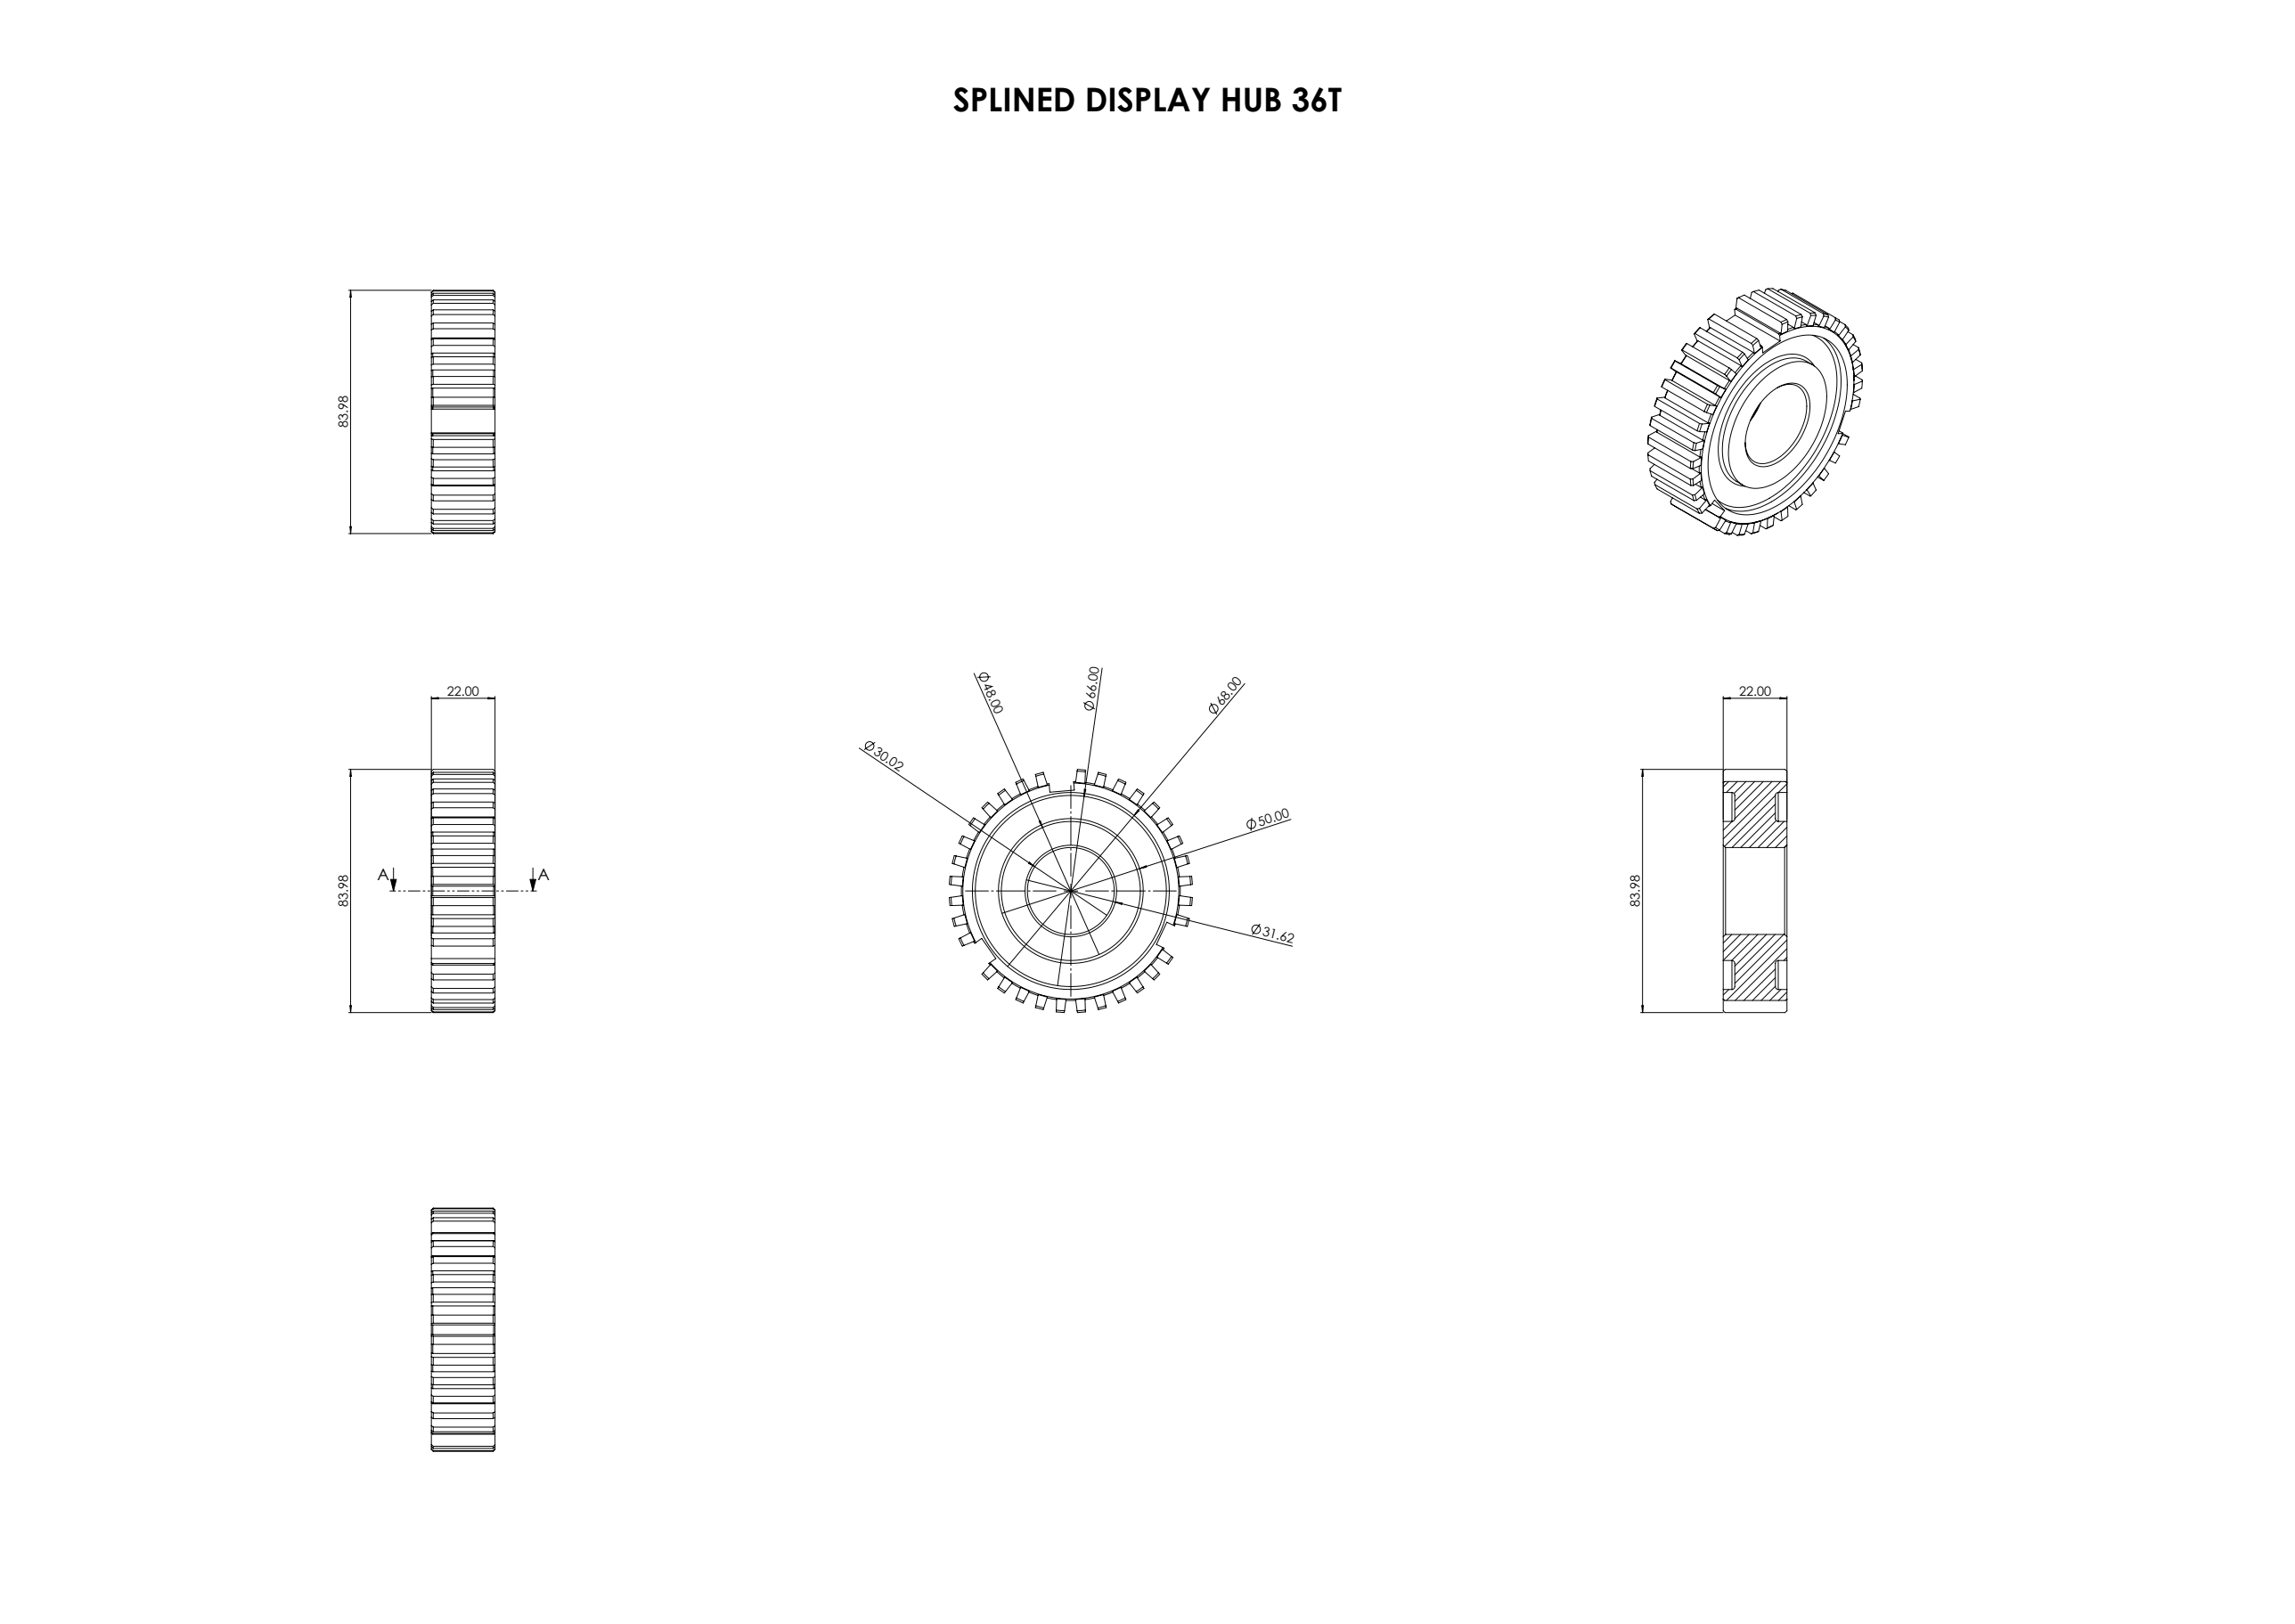
ISO-10303-21;
HEADER;
/* Generated by software containing ST-Developer
 * from STEP Tools, Inc. (www.steptools.com) 
 */

FILE_DESCRIPTION(
/* description */ (''),
/* implementation_level */ '2;1');

FILE_NAME(
/* name */ '02_Splined_Display_Hub_36T.step',
/* time_stamp */ '2026-10-11T08:27:52-07:00',
/* author */ (''),
/* organization */ (''),
/* preprocessor_version */ 'ST-DEVELOPER v20.2',
/* originating_system */ 'Autodesk Translation Framework v15.15.0.0',
/* authorisation */ '');

FILE_SCHEMA (('AUTOMOTIVE_DESIGN { 1 0 10303 214 3 1 1 }'));
ENDSEC;

DATA;
#10=MECHANICAL_DESIGN_GEOMETRIC_PRESENTATION_REPRESENTATION('',(#920),#94301);
#892=SHAPE_REPRESENTATION_RELATIONSHIP('SRR','None',#94372,#906);
#906=ADVANCED_BREP_SHAPE_REPRESENTATION('',(#934),#94288);
#920=STYLED_ITEM('',(#94595),#934);
#934=MANIFOLD_SOLID_BREP('Body1',#51019);
#950=TOROIDAL_SURFACE('',#54103,33.,1.);
#951=TOROIDAL_SURFACE('',#54112,33.,1.);
#952=TOROIDAL_SURFACE('',#54120,25.,1.);
#953=TOROIDAL_SURFACE('',#54126,25.,1.);
#963=FACE_BOUND('',#17327,.T.);
#964=FACE_BOUND('',#17673,.T.);
#965=FACE_BOUND('',#17677,.T.);
#966=FACE_BOUND('',#17686,.T.);
#967=FACE_BOUND('',#17688,.T.);
#968=FACE_BOUND('',#17690,.T.);
#1084=CYLINDRICAL_SURFACE('',#53612,37.8);
#1085=CYLINDRICAL_SURFACE('',#53689,37.8);
#1086=CYLINDRICAL_SURFACE('',#53706,37.8);
#1087=CYLINDRICAL_SURFACE('',#53942,37.8);
#1088=CYLINDRICAL_SURFACE('',#53943,37.8);
#1089=CYLINDRICAL_SURFACE('',#53948,37.8);
#1090=CYLINDRICAL_SURFACE('',#53953,37.8);
#1091=CYLINDRICAL_SURFACE('',#53958,37.8);
#1092=CYLINDRICAL_SURFACE('',#53963,37.8);
#1093=CYLINDRICAL_SURFACE('',#53968,37.8);
#1094=CYLINDRICAL_SURFACE('',#53973,37.8);
#1095=CYLINDRICAL_SURFACE('',#53978,37.8);
#1096=CYLINDRICAL_SURFACE('',#53983,37.8);
#1097=CYLINDRICAL_SURFACE('',#53988,37.8);
#1098=CYLINDRICAL_SURFACE('',#53993,37.8);
#1099=CYLINDRICAL_SURFACE('',#53998,37.8);
#1100=CYLINDRICAL_SURFACE('',#54003,37.8);
#1101=CYLINDRICAL_SURFACE('',#54008,37.8);
#1102=CYLINDRICAL_SURFACE('',#54013,37.8);
#1103=CYLINDRICAL_SURFACE('',#54018,37.8);
#1104=CYLINDRICAL_SURFACE('',#54023,37.8);
#1105=CYLINDRICAL_SURFACE('',#54028,37.8);
#1106=CYLINDRICAL_SURFACE('',#54033,37.8);
#1107=CYLINDRICAL_SURFACE('',#54038,37.8);
#1108=CYLINDRICAL_SURFACE('',#54043,37.8);
#1109=CYLINDRICAL_SURFACE('',#54048,37.8);
#1110=CYLINDRICAL_SURFACE('',#54053,37.8);
#1111=CYLINDRICAL_SURFACE('',#54058,37.8);
#1112=CYLINDRICAL_SURFACE('',#54063,37.8);
#1113=CYLINDRICAL_SURFACE('',#54068,37.8);
#1114=CYLINDRICAL_SURFACE('',#54073,37.8);
#1115=CYLINDRICAL_SURFACE('',#54078,37.8);
#1116=CYLINDRICAL_SURFACE('',#54083,37.8);
#1117=CYLINDRICAL_SURFACE('',#54088,37.8);
#1118=CYLINDRICAL_SURFACE('',#54093,37.8);
#1119=CYLINDRICAL_SURFACE('',#54098,37.8);
#1120=CYLINDRICAL_SURFACE('',#54110,34.);
#1121=CYLINDRICAL_SURFACE('',#54119,34.);
#1122=CYLINDRICAL_SURFACE('',#54124,24.);
#1123=CYLINDRICAL_SURFACE('',#54130,24.);
#1124=CYLINDRICAL_SURFACE('',#54132,15.01);
#4835=LINE('',#77424,#9363);
#4836=LINE('',#77426,#9364);
#4837=LINE('',#77428,#9365);
#4838=LINE('',#77433,#9366);
#4839=LINE('',#77441,#9367);
#4840=LINE('',#77447,#9368);
#4841=LINE('',#77449,#9369);
#4842=LINE('',#77450,#9370);
#4843=LINE('',#77452,#9371);
#4844=LINE('',#77453,#9372);
#4845=LINE('',#77458,#9373);
#4846=LINE('',#77626,#9374);
#4847=LINE('',#77628,#9375);
#4848=LINE('',#77630,#9376);
#4849=LINE('',#77634,#9377);
#4850=LINE('',#77636,#9378);
#4851=LINE('',#77638,#9379);
#4852=LINE('',#77962,#9380);
#4853=LINE('',#77963,#9381);
#4854=LINE('',#77964,#9382);
#4855=LINE('',#77972,#9383);
#4856=LINE('',#77977,#9384);
#4857=LINE('',#77978,#9385);
#4858=LINE('',#77980,#9386);
#4859=LINE('',#78304,#9387);
#4860=LINE('',#78467,#9388);
#4861=LINE('',#78468,#9389);
#4862=LINE('',#78469,#9390);
#4863=LINE('',#78471,#9391);
#4864=LINE('',#78473,#9392);
#4865=LINE('',#78474,#9393);
#4866=LINE('',#78476,#9394);
#4867=LINE('',#78478,#9395);
#4868=LINE('',#78976,#9396);
#4869=LINE('',#78982,#9397);
#4870=LINE('',#78983,#9398);
#4871=LINE('',#78984,#9399);
#4872=LINE('',#78986,#9400);
#4873=LINE('',#78987,#9401);
#4874=LINE('',#78990,#9402);
#4875=LINE('',#78996,#9403);
#4876=LINE('',#79002,#9404);
#4877=LINE('',#79003,#9405);
#4878=LINE('',#79004,#9406);
#4879=LINE('',#79006,#9407);
#4880=LINE('',#79007,#9408);
#4881=LINE('',#79010,#9409);
#4882=LINE('',#79016,#9410);
#4883=LINE('',#79022,#9411);
#4884=LINE('',#79023,#9412);
#4885=LINE('',#79024,#9413);
#4886=LINE('',#79026,#9414);
#4887=LINE('',#79027,#9415);
#4888=LINE('',#79030,#9416);
#4889=LINE('',#79036,#9417);
#4890=LINE('',#79042,#9418);
#4891=LINE('',#79043,#9419);
#4892=LINE('',#79044,#9420);
#4893=LINE('',#79046,#9421);
#4894=LINE('',#79047,#9422);
#4895=LINE('',#79050,#9423);
#4896=LINE('',#79056,#9424);
#4897=LINE('',#79062,#9425);
#4898=LINE('',#79063,#9426);
#4899=LINE('',#79064,#9427);
#4900=LINE('',#79066,#9428);
#4901=LINE('',#79067,#9429);
#4902=LINE('',#79070,#9430);
#4903=LINE('',#79076,#9431);
#4904=LINE('',#79082,#9432);
#4905=LINE('',#79083,#9433);
#4906=LINE('',#79084,#9434);
#4907=LINE('',#79086,#9435);
#4908=LINE('',#79087,#9436);
#4909=LINE('',#79090,#9437);
#4910=LINE('',#79096,#9438);
#4911=LINE('',#79102,#9439);
#4912=LINE('',#79103,#9440);
#4913=LINE('',#79104,#9441);
#4914=LINE('',#79106,#9442);
#4915=LINE('',#79107,#9443);
#4916=LINE('',#79110,#9444);
#4917=LINE('',#79116,#9445);
#4918=LINE('',#79122,#9446);
#4919=LINE('',#79123,#9447);
#4920=LINE('',#79124,#9448);
#4921=LINE('',#79126,#9449);
#4922=LINE('',#79127,#9450);
#4923=LINE('',#79130,#9451);
#4924=LINE('',#79136,#9452);
#4925=LINE('',#79142,#9453);
#4926=LINE('',#79143,#9454);
#4927=LINE('',#79144,#9455);
#4928=LINE('',#79146,#9456);
#4929=LINE('',#79147,#9457);
#4930=LINE('',#79150,#9458);
#4931=LINE('',#79156,#9459);
#4932=LINE('',#79162,#9460);
#4933=LINE('',#79163,#9461);
#4934=LINE('',#79164,#9462);
#4935=LINE('',#79166,#9463);
#4936=LINE('',#79167,#9464);
#4937=LINE('',#79170,#9465);
#4938=LINE('',#79176,#9466);
#4939=LINE('',#79182,#9467);
#4940=LINE('',#79183,#9468);
#4941=LINE('',#79184,#9469);
#4942=LINE('',#79186,#9470);
#4943=LINE('',#79187,#9471);
#4944=LINE('',#79190,#9472);
#4945=LINE('',#79196,#9473);
#4946=LINE('',#79202,#9474);
#4947=LINE('',#79203,#9475);
#4948=LINE('',#79204,#9476);
#4949=LINE('',#79206,#9477);
#4950=LINE('',#79207,#9478);
#4951=LINE('',#79210,#9479);
#4952=LINE('',#79216,#9480);
#4953=LINE('',#79222,#9481);
#4954=LINE('',#79223,#9482);
#4955=LINE('',#79224,#9483);
#4956=LINE('',#79226,#9484);
#4957=LINE('',#79227,#9485);
#4958=LINE('',#79230,#9486);
#4959=LINE('',#79236,#9487);
#4960=LINE('',#79242,#9488);
#4961=LINE('',#79243,#9489);
#4962=LINE('',#79244,#9490);
#4963=LINE('',#79246,#9491);
#4964=LINE('',#79247,#9492);
#4965=LINE('',#79250,#9493);
#4966=LINE('',#79256,#9494);
#4967=LINE('',#79262,#9495);
#4968=LINE('',#79263,#9496);
#4969=LINE('',#79264,#9497);
#4970=LINE('',#79266,#9498);
#4971=LINE('',#79267,#9499);
#4972=LINE('',#79270,#9500);
#4973=LINE('',#79276,#9501);
#4974=LINE('',#79282,#9502);
#4975=LINE('',#79283,#9503);
#4976=LINE('',#79284,#9504);
#4977=LINE('',#79286,#9505);
#4978=LINE('',#79287,#9506);
#4979=LINE('',#79290,#9507);
#4980=LINE('',#79296,#9508);
#4981=LINE('',#79302,#9509);
#4982=LINE('',#79303,#9510);
#4983=LINE('',#79304,#9511);
#4984=LINE('',#79306,#9512);
#4985=LINE('',#79307,#9513);
#4986=LINE('',#79310,#9514);
#4987=LINE('',#79316,#9515);
#4988=LINE('',#79322,#9516);
#4989=LINE('',#79323,#9517);
#4990=LINE('',#79324,#9518);
#4991=LINE('',#79326,#9519);
#4992=LINE('',#79327,#9520);
#4993=LINE('',#79330,#9521);
#4994=LINE('',#79336,#9522);
#4995=LINE('',#79342,#9523);
#4996=LINE('',#79343,#9524);
#4997=LINE('',#79344,#9525);
#4998=LINE('',#79346,#9526);
#4999=LINE('',#79347,#9527);
#5000=LINE('',#79350,#9528);
#5001=LINE('',#79356,#9529);
#5002=LINE('',#79362,#9530);
#5003=LINE('',#79363,#9531);
#5004=LINE('',#79364,#9532);
#5005=LINE('',#79366,#9533);
#5006=LINE('',#79367,#9534);
#5007=LINE('',#79370,#9535);
#5008=LINE('',#79376,#9536);
#5009=LINE('',#79382,#9537);
#5010=LINE('',#79383,#9538);
#5011=LINE('',#79384,#9539);
#5012=LINE('',#79386,#9540);
#5013=LINE('',#79387,#9541);
#5014=LINE('',#79390,#9542);
#5015=LINE('',#79396,#9543);
#5016=LINE('',#79402,#9544);
#5017=LINE('',#79403,#9545);
#5018=LINE('',#79404,#9546);
#5019=LINE('',#79406,#9547);
#5020=LINE('',#79407,#9548);
#5021=LINE('',#79410,#9549);
#5022=LINE('',#79416,#9550);
#5023=LINE('',#79422,#9551);
#5024=LINE('',#79423,#9552);
#5025=LINE('',#79424,#9553);
#5026=LINE('',#79426,#9554);
#5027=LINE('',#79427,#9555);
#5028=LINE('',#79430,#9556);
#5029=LINE('',#79436,#9557);
#5030=LINE('',#79442,#9558);
#5031=LINE('',#79443,#9559);
#5032=LINE('',#79444,#9560);
#5033=LINE('',#79446,#9561);
#5034=LINE('',#79447,#9562);
#5035=LINE('',#79450,#9563);
#5036=LINE('',#79456,#9564);
#5037=LINE('',#79462,#9565);
#5038=LINE('',#79463,#9566);
#5039=LINE('',#79464,#9567);
#5040=LINE('',#79466,#9568);
#5041=LINE('',#79467,#9569);
#5042=LINE('',#79470,#9570);
#5043=LINE('',#79476,#9571);
#5044=LINE('',#79482,#9572);
#5045=LINE('',#79483,#9573);
#5046=LINE('',#79484,#9574);
#5047=LINE('',#79486,#9575);
#5048=LINE('',#79487,#9576);
#5049=LINE('',#79490,#9577);
#5050=LINE('',#79496,#9578);
#5051=LINE('',#79502,#9579);
#5052=LINE('',#79503,#9580);
#5053=LINE('',#79504,#9581);
#5054=LINE('',#79506,#9582);
#5055=LINE('',#79507,#9583);
#5056=LINE('',#79510,#9584);
#5057=LINE('',#79516,#9585);
#5058=LINE('',#79522,#9586);
#5059=LINE('',#79523,#9587);
#5060=LINE('',#79524,#9588);
#5061=LINE('',#79526,#9589);
#5062=LINE('',#79527,#9590);
#5063=LINE('',#79530,#9591);
#5064=LINE('',#79536,#9592);
#5065=LINE('',#79542,#9593);
#5066=LINE('',#79543,#9594);
#5067=LINE('',#79544,#9595);
#5068=LINE('',#79546,#9596);
#5069=LINE('',#79547,#9597);
#5070=LINE('',#79550,#9598);
#5071=LINE('',#79556,#9599);
#5072=LINE('',#79562,#9600);
#5073=LINE('',#79563,#9601);
#5074=LINE('',#79564,#9602);
#5075=LINE('',#79566,#9603);
#5076=LINE('',#79567,#9604);
#5077=LINE('',#79570,#9605);
#5078=LINE('',#79576,#9606);
#5079=LINE('',#79582,#9607);
#5080=LINE('',#79583,#9608);
#5081=LINE('',#79584,#9609);
#5082=LINE('',#79586,#9610);
#5083=LINE('',#79587,#9611);
#5084=LINE('',#79590,#9612);
#5085=LINE('',#79596,#9613);
#5086=LINE('',#79602,#9614);
#5087=LINE('',#79603,#9615);
#5088=LINE('',#79604,#9616);
#5089=LINE('',#79606,#9617);
#5090=LINE('',#79607,#9618);
#5091=LINE('',#79610,#9619);
#5092=LINE('',#79616,#9620);
#5093=LINE('',#79622,#9621);
#5094=LINE('',#79623,#9622);
#5095=LINE('',#79624,#9623);
#5096=LINE('',#79626,#9624);
#5097=LINE('',#79627,#9625);
#5098=LINE('',#79630,#9626);
#5099=LINE('',#79834,#9627);
#5100=LINE('',#79835,#9628);
#5101=LINE('',#79836,#9629);
#5102=LINE('',#79838,#9630);
#5103=LINE('',#79839,#9631);
#5104=LINE('',#79842,#9632);
#5105=LINE('',#79843,#9633);
#5106=LINE('',#79844,#9634);
#5107=LINE('',#79846,#9635);
#5108=LINE('',#79847,#9636);
#5109=LINE('',#79850,#9637);
#5110=LINE('',#79851,#9638);
#5111=LINE('',#79852,#9639);
#5112=LINE('',#79854,#9640);
#5113=LINE('',#79855,#9641);
#5114=LINE('',#79858,#9642);
#5115=LINE('',#79859,#9643);
#5116=LINE('',#79860,#9644);
#5117=LINE('',#79862,#9645);
#5118=LINE('',#79863,#9646);
#5119=LINE('',#79866,#9647);
#5120=LINE('',#79867,#9648);
#5121=LINE('',#79868,#9649);
#5122=LINE('',#79870,#9650);
#5123=LINE('',#79871,#9651);
#5124=LINE('',#79874,#9652);
#5125=LINE('',#79875,#9653);
#5126=LINE('',#79876,#9654);
#5127=LINE('',#79878,#9655);
#5128=LINE('',#79879,#9656);
#5129=LINE('',#79882,#9657);
#5130=LINE('',#79883,#9658);
#5131=LINE('',#79884,#9659);
#5132=LINE('',#79886,#9660);
#5133=LINE('',#79887,#9661);
#5134=LINE('',#79890,#9662);
#5135=LINE('',#79891,#9663);
#5136=LINE('',#79892,#9664);
#5137=LINE('',#79894,#9665);
#5138=LINE('',#79895,#9666);
#5139=LINE('',#79898,#9667);
#5140=LINE('',#79899,#9668);
#5141=LINE('',#79900,#9669);
#5142=LINE('',#79902,#9670);
#5143=LINE('',#79903,#9671);
#5144=LINE('',#79906,#9672);
#5145=LINE('',#79907,#9673);
#5146=LINE('',#79908,#9674);
#5147=LINE('',#79910,#9675);
#5148=LINE('',#79911,#9676);
#5149=LINE('',#79914,#9677);
#5150=LINE('',#79915,#9678);
#5151=LINE('',#79917,#9679);
#5152=LINE('',#79918,#9680);
#5153=LINE('',#79921,#9681);
#5154=LINE('',#79922,#9682);
#5155=LINE('',#79923,#9683);
#5156=LINE('',#79925,#9684);
#5157=LINE('',#79926,#9685);
#5158=LINE('',#79929,#9686);
#5159=LINE('',#79930,#9687);
#5160=LINE('',#79931,#9688);
#5161=LINE('',#79933,#9689);
#5162=LINE('',#79934,#9690);
#5163=LINE('',#79937,#9691);
#5164=LINE('',#79938,#9692);
#5165=LINE('',#79939,#9693);
#5166=LINE('',#79941,#9694);
#5167=LINE('',#79942,#9695);
#5168=LINE('',#79945,#9696);
#5169=LINE('',#79946,#9697);
#5170=LINE('',#79947,#9698);
#5171=LINE('',#79949,#9699);
#5172=LINE('',#79950,#9700);
#5173=LINE('',#79953,#9701);
#5174=LINE('',#79954,#9702);
#5175=LINE('',#79955,#9703);
#5176=LINE('',#79957,#9704);
#5177=LINE('',#79958,#9705);
#5178=LINE('',#79961,#9706);
#5179=LINE('',#79962,#9707);
#5180=LINE('',#79963,#9708);
#5181=LINE('',#79965,#9709);
#5182=LINE('',#79966,#9710);
#5183=LINE('',#79969,#9711);
#5184=LINE('',#79970,#9712);
#5185=LINE('',#79971,#9713);
#5186=LINE('',#79973,#9714);
#5187=LINE('',#79974,#9715);
#5188=LINE('',#79977,#9716);
#5189=LINE('',#79978,#9717);
#5190=LINE('',#79979,#9718);
#5191=LINE('',#79981,#9719);
#5192=LINE('',#79982,#9720);
#5193=LINE('',#79985,#9721);
#5194=LINE('',#79986,#9722);
#5195=LINE('',#79987,#9723);
#5196=LINE('',#79989,#9724);
#5197=LINE('',#79990,#9725);
#5198=LINE('',#79993,#9726);
#5199=LINE('',#79994,#9727);
#5200=LINE('',#79995,#9728);
#5201=LINE('',#79997,#9729);
#5202=LINE('',#79998,#9730);
#5203=LINE('',#80001,#9731);
#5204=LINE('',#80002,#9732);
#5205=LINE('',#80004,#9733);
#5206=LINE('',#80005,#9734);
#5207=LINE('',#80008,#9735);
#5208=LINE('',#80009,#9736);
#5209=LINE('',#80010,#9737);
#5210=LINE('',#80012,#9738);
#5211=LINE('',#80013,#9739);
#5212=LINE('',#80016,#9740);
#5213=LINE('',#80017,#9741);
#5214=LINE('',#80018,#9742);
#5215=LINE('',#80020,#9743);
#5216=LINE('',#80021,#9744);
#5217=LINE('',#80024,#9745);
#5218=LINE('',#80025,#9746);
#5219=LINE('',#80026,#9747);
#5220=LINE('',#80028,#9748);
#5221=LINE('',#80029,#9749);
#5222=LINE('',#80032,#9750);
#5223=LINE('',#80033,#9751);
#5224=LINE('',#80034,#9752);
#5225=LINE('',#80036,#9753);
#5226=LINE('',#80037,#9754);
#5227=LINE('',#80040,#9755);
#5228=LINE('',#80041,#9756);
#5229=LINE('',#80042,#9757);
#5230=LINE('',#80044,#9758);
#5231=LINE('',#80045,#9759);
#5232=LINE('',#80048,#9760);
#5233=LINE('',#80049,#9761);
#5234=LINE('',#80050,#9762);
#5235=LINE('',#80052,#9763);
#5236=LINE('',#80053,#9764);
#5237=LINE('',#80056,#9765);
#5238=LINE('',#80057,#9766);
#5239=LINE('',#80058,#9767);
#5240=LINE('',#80060,#9768);
#5241=LINE('',#80061,#9769);
#5242=LINE('',#80064,#9770);
#5243=LINE('',#80065,#9771);
#5244=LINE('',#80066,#9772);
#5245=LINE('',#80068,#9773);
#5246=LINE('',#80069,#9774);
#5247=LINE('',#80072,#9775);
#5248=LINE('',#80073,#9776);
#5249=LINE('',#80074,#9777);
#5250=LINE('',#80076,#9778);
#5251=LINE('',#80077,#9779);
#5252=LINE('',#80080,#9780);
#5253=LINE('',#80081,#9781);
#5254=LINE('',#80082,#9782);
#5255=LINE('',#80084,#9783);
#5256=LINE('',#80085,#9784);
#5257=LINE('',#80088,#9785);
#5258=LINE('',#80089,#9786);
#5259=LINE('',#80091,#9787);
#5260=LINE('',#80092,#9788);
#5261=LINE('',#80094,#9789);
#5262=LINE('',#80096,#9790);
#5263=LINE('',#80102,#9791);
#5264=LINE('',#80104,#9792);
#5265=LINE('',#80109,#9793);
#5266=LINE('',#80111,#9794);
#5267=LINE('',#80116,#9795);
#5268=LINE('',#80118,#9796);
#5269=LINE('',#80123,#9797);
#5270=LINE('',#80125,#9798);
#5271=LINE('',#80130,#9799);
#5272=LINE('',#80132,#9800);
#5273=LINE('',#80137,#9801);
#5274=LINE('',#80139,#9802);
#5275=LINE('',#80144,#9803);
#5276=LINE('',#80146,#9804);
#5277=LINE('',#80151,#9805);
#5278=LINE('',#80153,#9806);
#5279=LINE('',#80158,#9807);
#5280=LINE('',#80160,#9808);
#5281=LINE('',#80165,#9809);
#5282=LINE('',#80167,#9810);
#5283=LINE('',#80172,#9811);
#5284=LINE('',#80174,#9812);
#5285=LINE('',#80179,#9813);
#5286=LINE('',#80181,#9814);
#5287=LINE('',#80186,#9815);
#5288=LINE('',#80188,#9816);
#5289=LINE('',#80193,#9817);
#5290=LINE('',#80195,#9818);
#5291=LINE('',#80200,#9819);
#5292=LINE('',#80202,#9820);
#5293=LINE('',#80207,#9821);
#5294=LINE('',#80209,#9822);
#5295=LINE('',#80214,#9823);
#5296=LINE('',#80216,#9824);
#5297=LINE('',#80221,#9825);
#5298=LINE('',#80223,#9826);
#5299=LINE('',#80228,#9827);
#5300=LINE('',#80230,#9828);
#5301=LINE('',#80235,#9829);
#5302=LINE('',#80237,#9830);
#5303=LINE('',#80242,#9831);
#5304=LINE('',#80244,#9832);
#5305=LINE('',#80249,#9833);
#5306=LINE('',#80251,#9834);
#5307=LINE('',#80256,#9835);
#5308=LINE('',#80258,#9836);
#5309=LINE('',#80263,#9837);
#5310=LINE('',#80265,#9838);
#5311=LINE('',#80270,#9839);
#5312=LINE('',#80272,#9840);
#5313=LINE('',#80277,#9841);
#5314=LINE('',#80279,#9842);
#5315=LINE('',#80284,#9843);
#5316=LINE('',#80286,#9844);
#5317=LINE('',#80291,#9845);
#5318=LINE('',#80293,#9846);
#5319=LINE('',#80298,#9847);
#5320=LINE('',#80300,#9848);
#5321=LINE('',#80305,#9849);
#5322=LINE('',#80307,#9850);
#5323=LINE('',#80312,#9851);
#5324=LINE('',#80314,#9852);
#5325=LINE('',#80319,#9853);
#5326=LINE('',#80321,#9854);
#5327=LINE('',#80338,#9855);
#5328=LINE('',#80351,#9856);
#5329=LINE('',#80361,#9857);
#5330=LINE('',#80370,#9858);
#5331=LINE('',#80376,#9859);
#5332=LINE('',#80380,#9860);
#5333=LINE('',#80388,#9861);
#9363=VECTOR('',#62889,10.);
#9364=VECTOR('',#62890,10.);
#9365=VECTOR('',#62891,10.);
#9366=VECTOR('',#62892,10.);
#9367=VECTOR('',#62895,10.);
#9368=VECTOR('',#62896,10.);
#9369=VECTOR('',#62897,10.);
#9370=VECTOR('',#62898,10.);
#9371=VECTOR('',#62901,10.);
#9372=VECTOR('',#62902,10.);
#9373=VECTOR('',#62907,10.);
#9374=VECTOR('',#62942,10.);
#9375=VECTOR('',#62943,10.);
#9376=VECTOR('',#62944,10.);
#9377=VECTOR('',#62947,10.);
#9378=VECTOR('',#62948,10.);
#9379=VECTOR('',#62949,10.);
#9380=VECTOR('',#63006,10.);
#9381=VECTOR('',#63007,10.);
#9382=VECTOR('',#63008,10.);
#9383=VECTOR('',#63011,10.);
#9384=VECTOR('',#63012,10.);
#9385=VECTOR('',#63013,10.);
#9386=VECTOR('',#63016,10.);
#9387=VECTOR('',#63073,10.);
#9388=VECTOR('',#63102,10.);
#9389=VECTOR('',#63103,10.);
#9390=VECTOR('',#63104,10.);
#9391=VECTOR('',#63107,10.);
#9392=VECTOR('',#63108,10.);
#9393=VECTOR('',#63109,10.);
#9394=VECTOR('',#63112,10.);
#9395=VECTOR('',#63115,10.);
#9396=VECTOR('',#63250,10.);
#9397=VECTOR('',#63251,10.);
#9398=VECTOR('',#63252,10.);
#9399=VECTOR('',#63253,10.);
#9400=VECTOR('',#63254,10.);
#9401=VECTOR('',#63255,10.);
#9402=VECTOR('',#63258,10.);
#9403=VECTOR('',#63261,10.);
#9404=VECTOR('',#63262,10.);
#9405=VECTOR('',#63263,10.);
#9406=VECTOR('',#63264,10.);
#9407=VECTOR('',#63265,10.);
#9408=VECTOR('',#63266,10.);
#9409=VECTOR('',#63269,10.);
#9410=VECTOR('',#63272,10.);
#9411=VECTOR('',#63273,10.);
#9412=VECTOR('',#63274,10.);
#9413=VECTOR('',#63275,10.);
#9414=VECTOR('',#63276,10.);
#9415=VECTOR('',#63277,10.);
#9416=VECTOR('',#63280,10.);
#9417=VECTOR('',#63283,10.);
#9418=VECTOR('',#63284,10.);
#9419=VECTOR('',#63285,10.);
#9420=VECTOR('',#63286,10.);
#9421=VECTOR('',#63287,10.);
#9422=VECTOR('',#63288,10.);
#9423=VECTOR('',#63291,10.);
#9424=VECTOR('',#63294,10.);
#9425=VECTOR('',#63295,10.);
#9426=VECTOR('',#63296,10.);
#9427=VECTOR('',#63297,10.);
#9428=VECTOR('',#63298,10.);
#9429=VECTOR('',#63299,10.);
#9430=VECTOR('',#63302,10.);
#9431=VECTOR('',#63305,10.);
#9432=VECTOR('',#63306,10.);
#9433=VECTOR('',#63307,10.);
#9434=VECTOR('',#63308,10.);
#9435=VECTOR('',#63309,10.);
#9436=VECTOR('',#63310,10.);
#9437=VECTOR('',#63313,10.);
#9438=VECTOR('',#63316,10.);
#9439=VECTOR('',#63317,10.);
#9440=VECTOR('',#63318,10.);
#9441=VECTOR('',#63319,10.);
#9442=VECTOR('',#63320,10.);
#9443=VECTOR('',#63321,10.);
#9444=VECTOR('',#63324,10.);
#9445=VECTOR('',#63327,10.);
#9446=VECTOR('',#63328,10.);
#9447=VECTOR('',#63329,10.);
#9448=VECTOR('',#63330,10.);
#9449=VECTOR('',#63331,10.);
#9450=VECTOR('',#63332,10.);
#9451=VECTOR('',#63335,10.);
#9452=VECTOR('',#63338,10.);
#9453=VECTOR('',#63339,10.);
#9454=VECTOR('',#63340,10.);
#9455=VECTOR('',#63341,10.);
#9456=VECTOR('',#63342,10.);
#9457=VECTOR('',#63343,10.);
#9458=VECTOR('',#63346,10.);
#9459=VECTOR('',#63349,10.);
#9460=VECTOR('',#63350,10.);
#9461=VECTOR('',#63351,10.);
#9462=VECTOR('',#63352,10.);
#9463=VECTOR('',#63353,10.);
#9464=VECTOR('',#63354,10.);
#9465=VECTOR('',#63357,10.);
#9466=VECTOR('',#63360,10.);
#9467=VECTOR('',#63361,10.);
#9468=VECTOR('',#63362,10.);
#9469=VECTOR('',#63363,10.);
#9470=VECTOR('',#63364,10.);
#9471=VECTOR('',#63365,10.);
#9472=VECTOR('',#63368,10.);
#9473=VECTOR('',#63371,10.);
#9474=VECTOR('',#63372,10.);
#9475=VECTOR('',#63373,10.);
#9476=VECTOR('',#63374,10.);
#9477=VECTOR('',#63375,10.);
#9478=VECTOR('',#63376,10.);
#9479=VECTOR('',#63379,10.);
#9480=VECTOR('',#63382,10.);
#9481=VECTOR('',#63383,10.);
#9482=VECTOR('',#63384,10.);
#9483=VECTOR('',#63385,10.);
#9484=VECTOR('',#63386,10.);
#9485=VECTOR('',#63387,10.);
#9486=VECTOR('',#63390,10.);
#9487=VECTOR('',#63393,10.);
#9488=VECTOR('',#63394,10.);
#9489=VECTOR('',#63395,10.);
#9490=VECTOR('',#63396,10.);
#9491=VECTOR('',#63397,10.);
#9492=VECTOR('',#63398,10.);
#9493=VECTOR('',#63401,10.);
#9494=VECTOR('',#63404,10.);
#9495=VECTOR('',#63405,10.);
#9496=VECTOR('',#63406,10.);
#9497=VECTOR('',#63407,10.);
#9498=VECTOR('',#63408,10.);
#9499=VECTOR('',#63409,10.);
#9500=VECTOR('',#63412,10.);
#9501=VECTOR('',#63415,10.);
#9502=VECTOR('',#63416,10.);
#9503=VECTOR('',#63417,10.);
#9504=VECTOR('',#63418,10.);
#9505=VECTOR('',#63419,10.);
#9506=VECTOR('',#63420,10.);
#9507=VECTOR('',#63423,10.);
#9508=VECTOR('',#63426,10.);
#9509=VECTOR('',#63427,10.);
#9510=VECTOR('',#63428,10.);
#9511=VECTOR('',#63429,10.);
#9512=VECTOR('',#63430,10.);
#9513=VECTOR('',#63431,10.);
#9514=VECTOR('',#63434,10.);
#9515=VECTOR('',#63437,10.);
#9516=VECTOR('',#63438,10.);
#9517=VECTOR('',#63439,10.);
#9518=VECTOR('',#63440,10.);
#9519=VECTOR('',#63441,10.);
#9520=VECTOR('',#63442,10.);
#9521=VECTOR('',#63445,10.);
#9522=VECTOR('',#63448,10.);
#9523=VECTOR('',#63449,10.);
#9524=VECTOR('',#63450,10.);
#9525=VECTOR('',#63451,10.);
#9526=VECTOR('',#63452,10.);
#9527=VECTOR('',#63453,10.);
#9528=VECTOR('',#63456,10.);
#9529=VECTOR('',#63459,10.);
#9530=VECTOR('',#63460,10.);
#9531=VECTOR('',#63461,10.);
#9532=VECTOR('',#63462,10.);
#9533=VECTOR('',#63463,10.);
#9534=VECTOR('',#63464,10.);
#9535=VECTOR('',#63467,10.);
#9536=VECTOR('',#63470,10.);
#9537=VECTOR('',#63471,10.);
#9538=VECTOR('',#63472,10.);
#9539=VECTOR('',#63473,10.);
#9540=VECTOR('',#63474,10.);
#9541=VECTOR('',#63475,10.);
#9542=VECTOR('',#63478,10.);
#9543=VECTOR('',#63481,10.);
#9544=VECTOR('',#63482,10.);
#9545=VECTOR('',#63483,10.);
#9546=VECTOR('',#63484,10.);
#9547=VECTOR('',#63485,10.);
#9548=VECTOR('',#63486,10.);
#9549=VECTOR('',#63489,10.);
#9550=VECTOR('',#63492,10.);
#9551=VECTOR('',#63493,10.);
#9552=VECTOR('',#63494,10.);
#9553=VECTOR('',#63495,10.);
#9554=VECTOR('',#63496,10.);
#9555=VECTOR('',#63497,10.);
#9556=VECTOR('',#63500,10.);
#9557=VECTOR('',#63503,10.);
#9558=VECTOR('',#63504,10.);
#9559=VECTOR('',#63505,10.);
#9560=VECTOR('',#63506,10.);
#9561=VECTOR('',#63507,10.);
#9562=VECTOR('',#63508,10.);
#9563=VECTOR('',#63511,10.);
#9564=VECTOR('',#63514,10.);
#9565=VECTOR('',#63515,10.);
#9566=VECTOR('',#63516,10.);
#9567=VECTOR('',#63517,10.);
#9568=VECTOR('',#63518,10.);
#9569=VECTOR('',#63519,10.);
#9570=VECTOR('',#63522,10.);
#9571=VECTOR('',#63525,10.);
#9572=VECTOR('',#63526,10.);
#9573=VECTOR('',#63527,10.);
#9574=VECTOR('',#63528,10.);
#9575=VECTOR('',#63529,10.);
#9576=VECTOR('',#63530,10.);
#9577=VECTOR('',#63533,10.);
#9578=VECTOR('',#63536,10.);
#9579=VECTOR('',#63537,10.);
#9580=VECTOR('',#63538,10.);
#9581=VECTOR('',#63539,10.);
#9582=VECTOR('',#63540,10.);
#9583=VECTOR('',#63541,10.);
#9584=VECTOR('',#63544,10.);
#9585=VECTOR('',#63547,10.);
#9586=VECTOR('',#63548,10.);
#9587=VECTOR('',#63549,10.);
#9588=VECTOR('',#63550,10.);
#9589=VECTOR('',#63551,10.);
#9590=VECTOR('',#63552,10.);
#9591=VECTOR('',#63555,10.);
#9592=VECTOR('',#63558,10.);
#9593=VECTOR('',#63559,10.);
#9594=VECTOR('',#63560,10.);
#9595=VECTOR('',#63561,10.);
#9596=VECTOR('',#63562,10.);
#9597=VECTOR('',#63563,10.);
#9598=VECTOR('',#63566,10.);
#9599=VECTOR('',#63569,10.);
#9600=VECTOR('',#63570,10.);
#9601=VECTOR('',#63571,10.);
#9602=VECTOR('',#63572,10.);
#9603=VECTOR('',#63573,10.);
#9604=VECTOR('',#63574,10.);
#9605=VECTOR('',#63577,10.);
#9606=VECTOR('',#63580,10.);
#9607=VECTOR('',#63581,10.);
#9608=VECTOR('',#63582,10.);
#9609=VECTOR('',#63583,10.);
#9610=VECTOR('',#63584,10.);
#9611=VECTOR('',#63585,10.);
#9612=VECTOR('',#63588,10.);
#9613=VECTOR('',#63591,10.);
#9614=VECTOR('',#63592,10.);
#9615=VECTOR('',#63593,10.);
#9616=VECTOR('',#63594,10.);
#9617=VECTOR('',#63595,10.);
#9618=VECTOR('',#63596,10.);
#9619=VECTOR('',#63599,10.);
#9620=VECTOR('',#63602,10.);
#9621=VECTOR('',#63603,10.);
#9622=VECTOR('',#63604,10.);
#9623=VECTOR('',#63605,10.);
#9624=VECTOR('',#63606,10.);
#9625=VECTOR('',#63607,10.);
#9626=VECTOR('',#63610,10.);
#9627=VECTOR('',#63745,10.);
#9628=VECTOR('',#63746,10.);
#9629=VECTOR('',#63747,10.);
#9630=VECTOR('',#63748,10.);
#9631=VECTOR('',#63749,10.);
#9632=VECTOR('',#63752,10.);
#9633=VECTOR('',#63753,10.);
#9634=VECTOR('',#63754,10.);
#9635=VECTOR('',#63755,10.);
#9636=VECTOR('',#63756,10.);
#9637=VECTOR('',#63759,10.);
#9638=VECTOR('',#63760,10.);
#9639=VECTOR('',#63761,10.);
#9640=VECTOR('',#63762,10.);
#9641=VECTOR('',#63763,10.);
#9642=VECTOR('',#63766,10.);
#9643=VECTOR('',#63767,10.);
#9644=VECTOR('',#63768,10.);
#9645=VECTOR('',#63769,10.);
#9646=VECTOR('',#63770,10.);
#9647=VECTOR('',#63773,10.);
#9648=VECTOR('',#63774,10.);
#9649=VECTOR('',#63775,10.);
#9650=VECTOR('',#63776,10.);
#9651=VECTOR('',#63777,10.);
#9652=VECTOR('',#63780,10.);
#9653=VECTOR('',#63781,10.);
#9654=VECTOR('',#63782,10.);
#9655=VECTOR('',#63783,10.);
#9656=VECTOR('',#63784,10.);
#9657=VECTOR('',#63787,10.);
#9658=VECTOR('',#63788,10.);
#9659=VECTOR('',#63789,10.);
#9660=VECTOR('',#63790,10.);
#9661=VECTOR('',#63791,10.);
#9662=VECTOR('',#63794,10.);
#9663=VECTOR('',#63795,10.);
#9664=VECTOR('',#63796,10.);
#9665=VECTOR('',#63797,10.);
#9666=VECTOR('',#63798,10.);
#9667=VECTOR('',#63801,10.);
#9668=VECTOR('',#63802,10.);
#9669=VECTOR('',#63803,10.);
#9670=VECTOR('',#63804,10.);
#9671=VECTOR('',#63805,10.);
#9672=VECTOR('',#63808,10.);
#9673=VECTOR('',#63809,10.);
#9674=VECTOR('',#63810,10.);
#9675=VECTOR('',#63811,10.);
#9676=VECTOR('',#63812,10.);
#9677=VECTOR('',#63815,10.);
#9678=VECTOR('',#63816,10.);
#9679=VECTOR('',#63817,10.);
#9680=VECTOR('',#63818,10.);
#9681=VECTOR('',#63821,10.);
#9682=VECTOR('',#63822,10.);
#9683=VECTOR('',#63823,10.);
#9684=VECTOR('',#63824,10.);
#9685=VECTOR('',#63825,10.);
#9686=VECTOR('',#63828,10.);
#9687=VECTOR('',#63829,10.);
#9688=VECTOR('',#63830,10.);
#9689=VECTOR('',#63831,10.);
#9690=VECTOR('',#63832,10.);
#9691=VECTOR('',#63835,10.);
#9692=VECTOR('',#63836,10.);
#9693=VECTOR('',#63837,10.);
#9694=VECTOR('',#63838,10.);
#9695=VECTOR('',#63839,10.);
#9696=VECTOR('',#63842,10.);
#9697=VECTOR('',#63843,10.);
#9698=VECTOR('',#63844,10.);
#9699=VECTOR('',#63845,10.);
#9700=VECTOR('',#63846,10.);
#9701=VECTOR('',#63849,10.);
#9702=VECTOR('',#63850,10.);
#9703=VECTOR('',#63851,10.);
#9704=VECTOR('',#63852,10.);
#9705=VECTOR('',#63853,10.);
#9706=VECTOR('',#63856,10.);
#9707=VECTOR('',#63857,10.);
#9708=VECTOR('',#63858,10.);
#9709=VECTOR('',#63859,10.);
#9710=VECTOR('',#63860,10.);
#9711=VECTOR('',#63863,10.);
#9712=VECTOR('',#63864,10.);
#9713=VECTOR('',#63865,10.);
#9714=VECTOR('',#63866,10.);
#9715=VECTOR('',#63867,10.);
#9716=VECTOR('',#63870,10.);
#9717=VECTOR('',#63871,10.);
#9718=VECTOR('',#63872,10.);
#9719=VECTOR('',#63873,10.);
#9720=VECTOR('',#63874,10.);
#9721=VECTOR('',#63877,10.);
#9722=VECTOR('',#63878,10.);
#9723=VECTOR('',#63879,10.);
#9724=VECTOR('',#63880,10.);
#9725=VECTOR('',#63881,10.);
#9726=VECTOR('',#63884,10.);
#9727=VECTOR('',#63885,10.);
#9728=VECTOR('',#63886,10.);
#9729=VECTOR('',#63887,10.);
#9730=VECTOR('',#63888,10.);
#9731=VECTOR('',#63891,10.);
#9732=VECTOR('',#63892,10.);
#9733=VECTOR('',#63893,10.);
#9734=VECTOR('',#63894,10.);
#9735=VECTOR('',#63897,10.);
#9736=VECTOR('',#63898,10.);
#9737=VECTOR('',#63899,10.);
#9738=VECTOR('',#63900,10.);
#9739=VECTOR('',#63901,10.);
#9740=VECTOR('',#63904,10.);
#9741=VECTOR('',#63905,10.);
#9742=VECTOR('',#63906,10.);
#9743=VECTOR('',#63907,10.);
#9744=VECTOR('',#63908,10.);
#9745=VECTOR('',#63911,10.);
#9746=VECTOR('',#63912,10.);
#9747=VECTOR('',#63913,10.);
#9748=VECTOR('',#63914,10.);
#9749=VECTOR('',#63915,10.);
#9750=VECTOR('',#63918,10.);
#9751=VECTOR('',#63919,10.);
#9752=VECTOR('',#63920,10.);
#9753=VECTOR('',#63921,10.);
#9754=VECTOR('',#63922,10.);
#9755=VECTOR('',#63925,10.);
#9756=VECTOR('',#63926,10.);
#9757=VECTOR('',#63927,10.);
#9758=VECTOR('',#63928,10.);
#9759=VECTOR('',#63929,10.);
#9760=VECTOR('',#63932,10.);
#9761=VECTOR('',#63933,10.);
#9762=VECTOR('',#63934,10.);
#9763=VECTOR('',#63935,10.);
#9764=VECTOR('',#63936,10.);
#9765=VECTOR('',#63939,10.);
#9766=VECTOR('',#63940,10.);
#9767=VECTOR('',#63941,10.);
#9768=VECTOR('',#63942,10.);
#9769=VECTOR('',#63943,10.);
#9770=VECTOR('',#63946,10.);
#9771=VECTOR('',#63947,10.);
#9772=VECTOR('',#63948,10.);
#9773=VECTOR('',#63949,10.);
#9774=VECTOR('',#63950,10.);
#9775=VECTOR('',#63953,10.);
#9776=VECTOR('',#63954,10.);
#9777=VECTOR('',#63955,10.);
#9778=VECTOR('',#63956,10.);
#9779=VECTOR('',#63957,10.);
#9780=VECTOR('',#63960,10.);
#9781=VECTOR('',#63961,10.);
#9782=VECTOR('',#63962,10.);
#9783=VECTOR('',#63963,10.);
#9784=VECTOR('',#63964,10.);
#9785=VECTOR('',#63967,10.);
#9786=VECTOR('',#63968,10.);
#9787=VECTOR('',#63969,10.);
#9788=VECTOR('',#63970,10.);
#9789=VECTOR('',#63973,10.);
#9790=VECTOR('',#63976,10.);
#9791=VECTOR('',#63987,10.);
#9792=VECTOR('',#63990,10.);
#9793=VECTOR('',#63999,10.);
#9794=VECTOR('',#64002,10.);
#9795=VECTOR('',#64011,10.);
#9796=VECTOR('',#64014,10.);
#9797=VECTOR('',#64023,10.);
#9798=VECTOR('',#64026,10.);
#9799=VECTOR('',#64035,10.);
#9800=VECTOR('',#64038,10.);
#9801=VECTOR('',#64047,10.);
#9802=VECTOR('',#64050,10.);
#9803=VECTOR('',#64059,10.);
#9804=VECTOR('',#64062,10.);
#9805=VECTOR('',#64071,10.);
#9806=VECTOR('',#64074,10.);
#9807=VECTOR('',#64083,10.);
#9808=VECTOR('',#64086,10.);
#9809=VECTOR('',#64095,10.);
#9810=VECTOR('',#64098,10.);
#9811=VECTOR('',#64107,10.);
#9812=VECTOR('',#64110,10.);
#9813=VECTOR('',#64119,10.);
#9814=VECTOR('',#64122,10.);
#9815=VECTOR('',#64131,10.);
#9816=VECTOR('',#64134,10.);
#9817=VECTOR('',#64143,10.);
#9818=VECTOR('',#64146,10.);
#9819=VECTOR('',#64155,10.);
#9820=VECTOR('',#64158,10.);
#9821=VECTOR('',#64167,10.);
#9822=VECTOR('',#64170,10.);
#9823=VECTOR('',#64179,10.);
#9824=VECTOR('',#64182,10.);
#9825=VECTOR('',#64191,10.);
#9826=VECTOR('',#64194,10.);
#9827=VECTOR('',#64203,10.);
#9828=VECTOR('',#64206,10.);
#9829=VECTOR('',#64215,10.);
#9830=VECTOR('',#64218,10.);
#9831=VECTOR('',#64227,10.);
#9832=VECTOR('',#64230,10.);
#9833=VECTOR('',#64239,10.);
#9834=VECTOR('',#64242,10.);
#9835=VECTOR('',#64251,10.);
#9836=VECTOR('',#64254,10.);
#9837=VECTOR('',#64263,10.);
#9838=VECTOR('',#64266,10.);
#9839=VECTOR('',#64275,10.);
#9840=VECTOR('',#64278,10.);
#9841=VECTOR('',#64287,10.);
#9842=VECTOR('',#64290,10.);
#9843=VECTOR('',#64299,10.);
#9844=VECTOR('',#64302,10.);
#9845=VECTOR('',#64311,10.);
#9846=VECTOR('',#64314,10.);
#9847=VECTOR('',#64323,10.);
#9848=VECTOR('',#64326,10.);
#9849=VECTOR('',#64335,10.);
#9850=VECTOR('',#64338,10.);
#9851=VECTOR('',#64347,10.);
#9852=VECTOR('',#64350,10.);
#9853=VECTOR('',#64359,10.);
#9854=VECTOR('',#64362,10.);
#9855=VECTOR('',#64385,34.);
#9856=VECTOR('',#64402,34.);
#9857=VECTOR('',#64415,24.);
#9858=VECTOR('',#64426,24.);
#9859=VECTOR('',#64433,15.01);
#9860=VECTOR('',#64438,15.41);
#9861=VECTOR('',#64451,15.41);
#12480=PLANE('',#53609);
#12481=PLANE('',#53610);
#12482=PLANE('',#53611);
#12483=PLANE('',#53629);
#12484=PLANE('',#53659);
#12485=PLANE('',#53660);
#12486=PLANE('',#53661);
#12487=PLANE('',#53703);
#12488=PLANE('',#53704);
#12489=PLANE('',#53705);
#12490=PLANE('',#53773);
#12491=PLANE('',#53774);
#12492=PLANE('',#53775);
#12493=PLANE('',#53776);
#12494=PLANE('',#53777);
#12495=PLANE('',#53778);
#12496=PLANE('',#53779);
#12497=PLANE('',#53780);
#12498=PLANE('',#53781);
#12499=PLANE('',#53782);
#12500=PLANE('',#53783);
#12501=PLANE('',#53784);
#12502=PLANE('',#53785);
#12503=PLANE('',#53786);
#12504=PLANE('',#53787);
#12505=PLANE('',#53788);
#12506=PLANE('',#53789);
#12507=PLANE('',#53790);
#12508=PLANE('',#53791);
#12509=PLANE('',#53792);
#12510=PLANE('',#53793);
#12511=PLANE('',#53794);
#12512=PLANE('',#53795);
#12513=PLANE('',#53796);
#12514=PLANE('',#53797);
#12515=PLANE('',#53798);
#12516=PLANE('',#53799);
#12517=PLANE('',#53800);
#12518=PLANE('',#53801);
#12519=PLANE('',#53802);
#12520=PLANE('',#53803);
#12521=PLANE('',#53804);
#12522=PLANE('',#53805);
#12523=PLANE('',#53806);
#12524=PLANE('',#53807);
#12525=PLANE('',#53808);
#12526=PLANE('',#53809);
#12527=PLANE('',#53810);
#12528=PLANE('',#53811);
#12529=PLANE('',#53812);
#12530=PLANE('',#53813);
#12531=PLANE('',#53814);
#12532=PLANE('',#53815);
#12533=PLANE('',#53816);
#12534=PLANE('',#53817);
#12535=PLANE('',#53818);
#12536=PLANE('',#53819);
#12537=PLANE('',#53820);
#12538=PLANE('',#53821);
#12539=PLANE('',#53822);
#12540=PLANE('',#53823);
#12541=PLANE('',#53824);
#12542=PLANE('',#53825);
#12543=PLANE('',#53826);
#12544=PLANE('',#53827);
#12545=PLANE('',#53828);
#12546=PLANE('',#53829);
#12547=PLANE('',#53830);
#12548=PLANE('',#53831);
#12549=PLANE('',#53832);
#12550=PLANE('',#53833);
#12551=PLANE('',#53834);
#12552=PLANE('',#53835);
#12553=PLANE('',#53836);
#12554=PLANE('',#53837);
#12555=PLANE('',#53838);
#12556=PLANE('',#53905);
#12557=PLANE('',#53906);
#12558=PLANE('',#53907);
#12559=PLANE('',#53908);
#12560=PLANE('',#53909);
#12561=PLANE('',#53910);
#12562=PLANE('',#53911);
#12563=PLANE('',#53912);
#12564=PLANE('',#53913);
#12565=PLANE('',#53914);
#12566=PLANE('',#53915);
#12567=PLANE('',#53916);
#12568=PLANE('',#53917);
#12569=PLANE('',#53918);
#12570=PLANE('',#53919);
#12571=PLANE('',#53920);
#12572=PLANE('',#53921);
#12573=PLANE('',#53922);
#12574=PLANE('',#53923);
#12575=PLANE('',#53924);
#12576=PLANE('',#53925);
#12577=PLANE('',#53926);
#12578=PLANE('',#53927);
#12579=PLANE('',#53928);
#12580=PLANE('',#53929);
#12581=PLANE('',#53930);
#12582=PLANE('',#53931);
#12583=PLANE('',#53932);
#12584=PLANE('',#53933);
#12585=PLANE('',#53934);
#12586=PLANE('',#53935);
#12587=PLANE('',#53936);
#12588=PLANE('',#53937);
#12589=PLANE('',#53938);
#12590=PLANE('',#53939);
#12591=PLANE('',#53940);
#12592=PLANE('',#53941);
#12593=PLANE('',#53944);
#12594=PLANE('',#53945);
#12595=PLANE('',#53946);
#12596=PLANE('',#53947);
#12597=PLANE('',#53949);
#12598=PLANE('',#53950);
#12599=PLANE('',#53951);
#12600=PLANE('',#53952);
#12601=PLANE('',#53954);
#12602=PLANE('',#53955);
#12603=PLANE('',#53956);
#12604=PLANE('',#53957);
#12605=PLANE('',#53959);
#12606=PLANE('',#53960);
#12607=PLANE('',#53961);
#12608=PLANE('',#53962);
#12609=PLANE('',#53964);
#12610=PLANE('',#53965);
#12611=PLANE('',#53966);
#12612=PLANE('',#53967);
#12613=PLANE('',#53969);
#12614=PLANE('',#53970);
#12615=PLANE('',#53971);
#12616=PLANE('',#53972);
#12617=PLANE('',#53974);
#12618=PLANE('',#53975);
#12619=PLANE('',#53976);
#12620=PLANE('',#53977);
#12621=PLANE('',#53979);
#12622=PLANE('',#53980);
#12623=PLANE('',#53981);
#12624=PLANE('',#53982);
#12625=PLANE('',#53984);
#12626=PLANE('',#53985);
#12627=PLANE('',#53986);
#12628=PLANE('',#53987);
#12629=PLANE('',#53989);
#12630=PLANE('',#53990);
#12631=PLANE('',#53991);
#12632=PLANE('',#53992);
#12633=PLANE('',#53994);
#12634=PLANE('',#53995);
#12635=PLANE('',#53996);
#12636=PLANE('',#53997);
#12637=PLANE('',#53999);
#12638=PLANE('',#54000);
#12639=PLANE('',#54001);
#12640=PLANE('',#54002);
#12641=PLANE('',#54004);
#12642=PLANE('',#54005);
#12643=PLANE('',#54006);
#12644=PLANE('',#54007);
#12645=PLANE('',#54009);
#12646=PLANE('',#54010);
#12647=PLANE('',#54011);
#12648=PLANE('',#54012);
#12649=PLANE('',#54014);
#12650=PLANE('',#54015);
#12651=PLANE('',#54016);
#12652=PLANE('',#54017);
#12653=PLANE('',#54019);
#12654=PLANE('',#54020);
#12655=PLANE('',#54021);
#12656=PLANE('',#54022);
#12657=PLANE('',#54024);
#12658=PLANE('',#54025);
#12659=PLANE('',#54026);
#12660=PLANE('',#54027);
#12661=PLANE('',#54029);
#12662=PLANE('',#54030);
#12663=PLANE('',#54031);
#12664=PLANE('',#54032);
#12665=PLANE('',#54034);
#12666=PLANE('',#54035);
#12667=PLANE('',#54036);
#12668=PLANE('',#54037);
#12669=PLANE('',#54039);
#12670=PLANE('',#54040);
#12671=PLANE('',#54041);
#12672=PLANE('',#54042);
#12673=PLANE('',#54044);
#12674=PLANE('',#54045);
#12675=PLANE('',#54046);
#12676=PLANE('',#54047);
#12677=PLANE('',#54049);
#12678=PLANE('',#54050);
#12679=PLANE('',#54051);
#12680=PLANE('',#54052);
#12681=PLANE('',#54054);
#12682=PLANE('',#54055);
#12683=PLANE('',#54056);
#12684=PLANE('',#54057);
#12685=PLANE('',#54059);
#12686=PLANE('',#54060);
#12687=PLANE('',#54061);
#12688=PLANE('',#54062);
#12689=PLANE('',#54064);
#12690=PLANE('',#54065);
#12691=PLANE('',#54066);
#12692=PLANE('',#54067);
#12693=PLANE('',#54069);
#12694=PLANE('',#54070);
#12695=PLANE('',#54071);
#12696=PLANE('',#54072);
#12697=PLANE('',#54074);
#12698=PLANE('',#54075);
#12699=PLANE('',#54076);
#12700=PLANE('',#54077);
#12701=PLANE('',#54079);
#12702=PLANE('',#54080);
#12703=PLANE('',#54081);
#12704=PLANE('',#54082);
#12705=PLANE('',#54084);
#12706=PLANE('',#54085);
#12707=PLANE('',#54086);
#12708=PLANE('',#54087);
#12709=PLANE('',#54089);
#12710=PLANE('',#54090);
#12711=PLANE('',#54091);
#12712=PLANE('',#54092);
#12713=PLANE('',#54094);
#12714=PLANE('',#54095);
#12715=PLANE('',#54096);
#12716=PLANE('',#54097);
#12717=PLANE('',#54099);
#12718=PLANE('',#54100);
#12719=PLANE('',#54101);
#12720=PLANE('',#54102);
#12721=PLANE('',#54108);
#12722=PLANE('',#54117);
#12723=PLANE('',#54137);
#12724=PLANE('',#54138);
#12725=PLANE('',#54139);
#14635=FACE_OUTER_BOUND('',#17321,.T.);
#14636=FACE_OUTER_BOUND('',#17322,.T.);
#14637=FACE_OUTER_BOUND('',#17323,.T.);
#14638=FACE_OUTER_BOUND('',#17324,.T.);
#14639=FACE_OUTER_BOUND('',#17325,.T.);
#14640=FACE_OUTER_BOUND('',#17326,.T.);
#14641=FACE_OUTER_BOUND('',#17328,.T.);
#14642=FACE_OUTER_BOUND('',#17329,.T.);
#14643=FACE_OUTER_BOUND('',#17330,.T.);
#14644=FACE_OUTER_BOUND('',#17331,.T.);
#14645=FACE_OUTER_BOUND('',#17332,.T.);
#14646=FACE_OUTER_BOUND('',#17333,.T.);
#14647=FACE_OUTER_BOUND('',#17334,.T.);
#14648=FACE_OUTER_BOUND('',#17335,.T.);
#14649=FACE_OUTER_BOUND('',#17336,.T.);
#14650=FACE_OUTER_BOUND('',#17337,.T.);
#14651=FACE_OUTER_BOUND('',#17338,.T.);
#14652=FACE_OUTER_BOUND('',#17339,.T.);
#14653=FACE_OUTER_BOUND('',#17340,.T.);
#14654=FACE_OUTER_BOUND('',#17341,.T.);
#14655=FACE_OUTER_BOUND('',#17342,.T.);
#14656=FACE_OUTER_BOUND('',#17343,.T.);
#14657=FACE_OUTER_BOUND('',#17344,.T.);
#14658=FACE_OUTER_BOUND('',#17345,.T.);
#14659=FACE_OUTER_BOUND('',#17346,.T.);
#14660=FACE_OUTER_BOUND('',#17347,.T.);
#14661=FACE_OUTER_BOUND('',#17348,.T.);
#14662=FACE_OUTER_BOUND('',#17349,.T.);
#14663=FACE_OUTER_BOUND('',#17350,.T.);
#14664=FACE_OUTER_BOUND('',#17351,.T.);
#14665=FACE_OUTER_BOUND('',#17352,.T.);
#14666=FACE_OUTER_BOUND('',#17353,.T.);
#14667=FACE_OUTER_BOUND('',#17354,.T.);
#14668=FACE_OUTER_BOUND('',#17355,.T.);
#14669=FACE_OUTER_BOUND('',#17356,.T.);
#14670=FACE_OUTER_BOUND('',#17357,.T.);
#14671=FACE_OUTER_BOUND('',#17358,.T.);
#14672=FACE_OUTER_BOUND('',#17359,.T.);
#14673=FACE_OUTER_BOUND('',#17360,.T.);
#14674=FACE_OUTER_BOUND('',#17361,.T.);
#14675=FACE_OUTER_BOUND('',#17362,.T.);
#14676=FACE_OUTER_BOUND('',#17363,.T.);
#14677=FACE_OUTER_BOUND('',#17364,.T.);
#14678=FACE_OUTER_BOUND('',#17365,.T.);
#14679=FACE_OUTER_BOUND('',#17366,.T.);
#14680=FACE_OUTER_BOUND('',#17367,.T.);
#14681=FACE_OUTER_BOUND('',#17368,.T.);
#14682=FACE_OUTER_BOUND('',#17369,.T.);
#14683=FACE_OUTER_BOUND('',#17370,.T.);
#14684=FACE_OUTER_BOUND('',#17371,.T.);
#14685=FACE_OUTER_BOUND('',#17372,.T.);
#14686=FACE_OUTER_BOUND('',#17373,.T.);
#14687=FACE_OUTER_BOUND('',#17374,.T.);
#14688=FACE_OUTER_BOUND('',#17375,.T.);
#14689=FACE_OUTER_BOUND('',#17376,.T.);
#14690=FACE_OUTER_BOUND('',#17377,.T.);
#14691=FACE_OUTER_BOUND('',#17378,.T.);
#14692=FACE_OUTER_BOUND('',#17379,.T.);
#14693=FACE_OUTER_BOUND('',#17380,.T.);
#14694=FACE_OUTER_BOUND('',#17381,.T.);
#14695=FACE_OUTER_BOUND('',#17382,.T.);
#14696=FACE_OUTER_BOUND('',#17383,.T.);
#14697=FACE_OUTER_BOUND('',#17384,.T.);
#14698=FACE_OUTER_BOUND('',#17385,.T.);
#14699=FACE_OUTER_BOUND('',#17386,.T.);
#14700=FACE_OUTER_BOUND('',#17387,.T.);
#14701=FACE_OUTER_BOUND('',#17388,.T.);
#14702=FACE_OUTER_BOUND('',#17389,.T.);
#14703=FACE_OUTER_BOUND('',#17390,.T.);
#14704=FACE_OUTER_BOUND('',#17391,.T.);
#14705=FACE_OUTER_BOUND('',#17392,.T.);
#14706=FACE_OUTER_BOUND('',#17393,.T.);
#14707=FACE_OUTER_BOUND('',#17394,.T.);
#14708=FACE_OUTER_BOUND('',#17395,.T.);
#14709=FACE_OUTER_BOUND('',#17396,.T.);
#14710=FACE_OUTER_BOUND('',#17397,.T.);
#14711=FACE_OUTER_BOUND('',#17398,.T.);
#14712=FACE_OUTER_BOUND('',#17399,.T.);
#14713=FACE_OUTER_BOUND('',#17400,.T.);
#14714=FACE_OUTER_BOUND('',#17401,.T.);
#14715=FACE_OUTER_BOUND('',#17402,.T.);
#14716=FACE_OUTER_BOUND('',#17403,.T.);
#14717=FACE_OUTER_BOUND('',#17404,.T.);
#14718=FACE_OUTER_BOUND('',#17405,.T.);
#14719=FACE_OUTER_BOUND('',#17406,.T.);
#14720=FACE_OUTER_BOUND('',#17407,.T.);
#14721=FACE_OUTER_BOUND('',#17408,.T.);
#14722=FACE_OUTER_BOUND('',#17409,.T.);
#14723=FACE_OUTER_BOUND('',#17410,.T.);
#14724=FACE_OUTER_BOUND('',#17411,.T.);
#14725=FACE_OUTER_BOUND('',#17412,.T.);
#14726=FACE_OUTER_BOUND('',#17413,.T.);
#14727=FACE_OUTER_BOUND('',#17414,.T.);
#14728=FACE_OUTER_BOUND('',#17415,.T.);
#14729=FACE_OUTER_BOUND('',#17416,.T.);
#14730=FACE_OUTER_BOUND('',#17417,.T.);
#14731=FACE_OUTER_BOUND('',#17418,.T.);
#14732=FACE_OUTER_BOUND('',#17419,.T.);
#14733=FACE_OUTER_BOUND('',#17420,.T.);
#14734=FACE_OUTER_BOUND('',#17421,.T.);
#14735=FACE_OUTER_BOUND('',#17422,.T.);
#14736=FACE_OUTER_BOUND('',#17423,.T.);
#14737=FACE_OUTER_BOUND('',#17424,.T.);
#14738=FACE_OUTER_BOUND('',#17425,.T.);
#14739=FACE_OUTER_BOUND('',#17426,.T.);
#14740=FACE_OUTER_BOUND('',#17427,.T.);
#14741=FACE_OUTER_BOUND('',#17428,.T.);
#14742=FACE_OUTER_BOUND('',#17429,.T.);
#14743=FACE_OUTER_BOUND('',#17430,.T.);
#14744=FACE_OUTER_BOUND('',#17431,.T.);
#14745=FACE_OUTER_BOUND('',#17432,.T.);
#14746=FACE_OUTER_BOUND('',#17433,.T.);
#14747=FACE_OUTER_BOUND('',#17434,.T.);
#14748=FACE_OUTER_BOUND('',#17435,.T.);
#14749=FACE_OUTER_BOUND('',#17436,.T.);
#14750=FACE_OUTER_BOUND('',#17437,.T.);
#14751=FACE_OUTER_BOUND('',#17438,.T.);
#14752=FACE_OUTER_BOUND('',#17439,.T.);
#14753=FACE_OUTER_BOUND('',#17440,.T.);
#14754=FACE_OUTER_BOUND('',#17441,.T.);
#14755=FACE_OUTER_BOUND('',#17442,.T.);
#14756=FACE_OUTER_BOUND('',#17443,.T.);
#14757=FACE_OUTER_BOUND('',#17444,.T.);
#14758=FACE_OUTER_BOUND('',#17445,.T.);
#14759=FACE_OUTER_BOUND('',#17446,.T.);
#14760=FACE_OUTER_BOUND('',#17447,.T.);
#14761=FACE_OUTER_BOUND('',#17448,.T.);
#14762=FACE_OUTER_BOUND('',#17449,.T.);
#14763=FACE_OUTER_BOUND('',#17450,.T.);
#14764=FACE_OUTER_BOUND('',#17451,.T.);
#14765=FACE_OUTER_BOUND('',#17452,.T.);
#14766=FACE_OUTER_BOUND('',#17453,.T.);
#14767=FACE_OUTER_BOUND('',#17454,.T.);
#14768=FACE_OUTER_BOUND('',#17455,.T.);
#14769=FACE_OUTER_BOUND('',#17456,.T.);
#14770=FACE_OUTER_BOUND('',#17457,.T.);
#14771=FACE_OUTER_BOUND('',#17458,.T.);
#14772=FACE_OUTER_BOUND('',#17459,.T.);
#14773=FACE_OUTER_BOUND('',#17460,.T.);
#14774=FACE_OUTER_BOUND('',#17461,.T.);
#14775=FACE_OUTER_BOUND('',#17462,.T.);
#14776=FACE_OUTER_BOUND('',#17463,.T.);
#14777=FACE_OUTER_BOUND('',#17464,.T.);
#14778=FACE_OUTER_BOUND('',#17465,.T.);
#14779=FACE_OUTER_BOUND('',#17466,.T.);
#14780=FACE_OUTER_BOUND('',#17467,.T.);
#14781=FACE_OUTER_BOUND('',#17468,.T.);
#14782=FACE_OUTER_BOUND('',#17469,.T.);
#14783=FACE_OUTER_BOUND('',#17470,.T.);
#14784=FACE_OUTER_BOUND('',#17471,.T.);
#14785=FACE_OUTER_BOUND('',#17472,.T.);
#14786=FACE_OUTER_BOUND('',#17473,.T.);
#14787=FACE_OUTER_BOUND('',#17474,.T.);
#14788=FACE_OUTER_BOUND('',#17475,.T.);
#14789=FACE_OUTER_BOUND('',#17476,.T.);
#14790=FACE_OUTER_BOUND('',#17477,.T.);
#14791=FACE_OUTER_BOUND('',#17478,.T.);
#14792=FACE_OUTER_BOUND('',#17479,.T.);
#14793=FACE_OUTER_BOUND('',#17480,.T.);
#14794=FACE_OUTER_BOUND('',#17481,.T.);
#14795=FACE_OUTER_BOUND('',#17482,.T.);
#14796=FACE_OUTER_BOUND('',#17483,.T.);
#14797=FACE_OUTER_BOUND('',#17484,.T.);
#14798=FACE_OUTER_BOUND('',#17485,.T.);
#14799=FACE_OUTER_BOUND('',#17486,.T.);
#14800=FACE_OUTER_BOUND('',#17487,.T.);
#14801=FACE_OUTER_BOUND('',#17488,.T.);
#14802=FACE_OUTER_BOUND('',#17489,.T.);
#14803=FACE_OUTER_BOUND('',#17490,.T.);
#14804=FACE_OUTER_BOUND('',#17491,.T.);
#14805=FACE_OUTER_BOUND('',#17492,.T.);
#14806=FACE_OUTER_BOUND('',#17493,.T.);
#14807=FACE_OUTER_BOUND('',#17494,.T.);
#14808=FACE_OUTER_BOUND('',#17495,.T.);
#14809=FACE_OUTER_BOUND('',#17496,.T.);
#14810=FACE_OUTER_BOUND('',#17497,.T.);
#14811=FACE_OUTER_BOUND('',#17498,.T.);
#14812=FACE_OUTER_BOUND('',#17499,.T.);
#14813=FACE_OUTER_BOUND('',#17500,.T.);
#14814=FACE_OUTER_BOUND('',#17501,.T.);
#14815=FACE_OUTER_BOUND('',#17502,.T.);
#14816=FACE_OUTER_BOUND('',#17503,.T.);
#14817=FACE_OUTER_BOUND('',#17504,.T.);
#14818=FACE_OUTER_BOUND('',#17505,.T.);
#14819=FACE_OUTER_BOUND('',#17506,.T.);
#14820=FACE_OUTER_BOUND('',#17507,.T.);
#14821=FACE_OUTER_BOUND('',#17508,.T.);
#14822=FACE_OUTER_BOUND('',#17509,.T.);
#14823=FACE_OUTER_BOUND('',#17510,.T.);
#14824=FACE_OUTER_BOUND('',#17511,.T.);
#14825=FACE_OUTER_BOUND('',#17512,.T.);
#14826=FACE_OUTER_BOUND('',#17513,.T.);
#14827=FACE_OUTER_BOUND('',#17514,.T.);
#14828=FACE_OUTER_BOUND('',#17515,.T.);
#14829=FACE_OUTER_BOUND('',#17516,.T.);
#14830=FACE_OUTER_BOUND('',#17517,.T.);
#14831=FACE_OUTER_BOUND('',#17518,.T.);
#14832=FACE_OUTER_BOUND('',#17519,.T.);
#14833=FACE_OUTER_BOUND('',#17520,.T.);
#14834=FACE_OUTER_BOUND('',#17521,.T.);
#14835=FACE_OUTER_BOUND('',#17522,.T.);
#14836=FACE_OUTER_BOUND('',#17523,.T.);
#14837=FACE_OUTER_BOUND('',#17524,.T.);
#14838=FACE_OUTER_BOUND('',#17525,.T.);
#14839=FACE_OUTER_BOUND('',#17526,.T.);
#14840=FACE_OUTER_BOUND('',#17527,.T.);
#14841=FACE_OUTER_BOUND('',#17528,.T.);
#14842=FACE_OUTER_BOUND('',#17529,.T.);
#14843=FACE_OUTER_BOUND('',#17530,.T.);
#14844=FACE_OUTER_BOUND('',#17531,.T.);
#14845=FACE_OUTER_BOUND('',#17532,.T.);
#14846=FACE_OUTER_BOUND('',#17533,.T.);
#14847=FACE_OUTER_BOUND('',#17534,.T.);
#14848=FACE_OUTER_BOUND('',#17535,.T.);
#14849=FACE_OUTER_BOUND('',#17536,.T.);
#14850=FACE_OUTER_BOUND('',#17537,.T.);
#14851=FACE_OUTER_BOUND('',#17538,.T.);
#14852=FACE_OUTER_BOUND('',#17539,.T.);
#14853=FACE_OUTER_BOUND('',#17540,.T.);
#14854=FACE_OUTER_BOUND('',#17541,.T.);
#14855=FACE_OUTER_BOUND('',#17542,.T.);
#14856=FACE_OUTER_BOUND('',#17543,.T.);
#14857=FACE_OUTER_BOUND('',#17544,.T.);
#14858=FACE_OUTER_BOUND('',#17545,.T.);
#14859=FACE_OUTER_BOUND('',#17546,.T.);
#14860=FACE_OUTER_BOUND('',#17547,.T.);
#14861=FACE_OUTER_BOUND('',#17548,.T.);
#14862=FACE_OUTER_BOUND('',#17549,.T.);
#14863=FACE_OUTER_BOUND('',#17550,.T.);
#14864=FACE_OUTER_BOUND('',#17551,.T.);
#14865=FACE_OUTER_BOUND('',#17552,.T.);
#14866=FACE_OUTER_BOUND('',#17553,.T.);
#14867=FACE_OUTER_BOUND('',#17554,.T.);
#14868=FACE_OUTER_BOUND('',#17555,.T.);
#14869=FACE_OUTER_BOUND('',#17556,.T.);
#14870=FACE_OUTER_BOUND('',#17557,.T.);
#14871=FACE_OUTER_BOUND('',#17558,.T.);
#14872=FACE_OUTER_BOUND('',#17559,.T.);
#14873=FACE_OUTER_BOUND('',#17560,.T.);
#14874=FACE_OUTER_BOUND('',#17561,.T.);
#14875=FACE_OUTER_BOUND('',#17562,.T.);
#14876=FACE_OUTER_BOUND('',#17563,.T.);
#14877=FACE_OUTER_BOUND('',#17564,.T.);
#14878=FACE_OUTER_BOUND('',#17565,.T.);
#14879=FACE_OUTER_BOUND('',#17566,.T.);
#14880=FACE_OUTER_BOUND('',#17567,.T.);
#14881=FACE_OUTER_BOUND('',#17568,.T.);
#14882=FACE_OUTER_BOUND('',#17569,.T.);
#14883=FACE_OUTER_BOUND('',#17570,.T.);
#14884=FACE_OUTER_BOUND('',#17571,.T.);
#14885=FACE_OUTER_BOUND('',#17572,.T.);
#14886=FACE_OUTER_BOUND('',#17573,.T.);
#14887=FACE_OUTER_BOUND('',#17574,.T.);
#14888=FACE_OUTER_BOUND('',#17575,.T.);
#14889=FACE_OUTER_BOUND('',#17576,.T.);
#14890=FACE_OUTER_BOUND('',#17577,.T.);
#14891=FACE_OUTER_BOUND('',#17578,.T.);
#14892=FACE_OUTER_BOUND('',#17579,.T.);
#14893=FACE_OUTER_BOUND('',#17580,.T.);
#14894=FACE_OUTER_BOUND('',#17581,.T.);
#14895=FACE_OUTER_BOUND('',#17582,.T.);
#14896=FACE_OUTER_BOUND('',#17583,.T.);
#14897=FACE_OUTER_BOUND('',#17584,.T.);
#14898=FACE_OUTER_BOUND('',#17585,.T.);
#14899=FACE_OUTER_BOUND('',#17586,.T.);
#14900=FACE_OUTER_BOUND('',#17587,.T.);
#14901=FACE_OUTER_BOUND('',#17588,.T.);
#14902=FACE_OUTER_BOUND('',#17589,.T.);
#14903=FACE_OUTER_BOUND('',#17590,.T.);
#14904=FACE_OUTER_BOUND('',#17591,.T.);
#14905=FACE_OUTER_BOUND('',#17592,.T.);
#14906=FACE_OUTER_BOUND('',#17593,.T.);
#14907=FACE_OUTER_BOUND('',#17594,.T.);
#14908=FACE_OUTER_BOUND('',#17595,.T.);
#14909=FACE_OUTER_BOUND('',#17596,.T.);
#14910=FACE_OUTER_BOUND('',#17597,.T.);
#14911=FACE_OUTER_BOUND('',#17598,.T.);
#14912=FACE_OUTER_BOUND('',#17599,.T.);
#14913=FACE_OUTER_BOUND('',#17600,.T.);
#14914=FACE_OUTER_BOUND('',#17601,.T.);
#14915=FACE_OUTER_BOUND('',#17602,.T.);
#14916=FACE_OUTER_BOUND('',#17603,.T.);
#14917=FACE_OUTER_BOUND('',#17604,.T.);
#14918=FACE_OUTER_BOUND('',#17605,.T.);
#14919=FACE_OUTER_BOUND('',#17606,.T.);
#14920=FACE_OUTER_BOUND('',#17607,.T.);
#14921=FACE_OUTER_BOUND('',#17608,.T.);
#14922=FACE_OUTER_BOUND('',#17609,.T.);
#14923=FACE_OUTER_BOUND('',#17610,.T.);
#14924=FACE_OUTER_BOUND('',#17611,.T.);
#14925=FACE_OUTER_BOUND('',#17612,.T.);
#14926=FACE_OUTER_BOUND('',#17613,.T.);
#14927=FACE_OUTER_BOUND('',#17614,.T.);
#14928=FACE_OUTER_BOUND('',#17615,.T.);
#14929=FACE_OUTER_BOUND('',#17616,.T.);
#14930=FACE_OUTER_BOUND('',#17617,.T.);
#14931=FACE_OUTER_BOUND('',#17618,.T.);
#14932=FACE_OUTER_BOUND('',#17619,.T.);
#14933=FACE_OUTER_BOUND('',#17620,.T.);
#14934=FACE_OUTER_BOUND('',#17621,.T.);
#14935=FACE_OUTER_BOUND('',#17622,.T.);
#14936=FACE_OUTER_BOUND('',#17623,.T.);
#14937=FACE_OUTER_BOUND('',#17624,.T.);
#14938=FACE_OUTER_BOUND('',#17625,.T.);
#14939=FACE_OUTER_BOUND('',#17626,.T.);
#14940=FACE_OUTER_BOUND('',#17627,.T.);
#14941=FACE_OUTER_BOUND('',#17628,.T.);
#14942=FACE_OUTER_BOUND('',#17629,.T.);
#14943=FACE_OUTER_BOUND('',#17630,.T.);
#14944=FACE_OUTER_BOUND('',#17631,.T.);
#14945=FACE_OUTER_BOUND('',#17632,.T.);
#14946=FACE_OUTER_BOUND('',#17633,.T.);
#14947=FACE_OUTER_BOUND('',#17634,.T.);
#14948=FACE_OUTER_BOUND('',#17635,.T.);
#14949=FACE_OUTER_BOUND('',#17636,.T.);
#14950=FACE_OUTER_BOUND('',#17637,.T.);
#14951=FACE_OUTER_BOUND('',#17638,.T.);
#14952=FACE_OUTER_BOUND('',#17639,.T.);
#14953=FACE_OUTER_BOUND('',#17640,.T.);
#14954=FACE_OUTER_BOUND('',#17641,.T.);
#14955=FACE_OUTER_BOUND('',#17642,.T.);
#14956=FACE_OUTER_BOUND('',#17643,.T.);
#14957=FACE_OUTER_BOUND('',#17644,.T.);
#14958=FACE_OUTER_BOUND('',#17645,.T.);
#14959=FACE_OUTER_BOUND('',#17646,.T.);
#14960=FACE_OUTER_BOUND('',#17647,.T.);
#14961=FACE_OUTER_BOUND('',#17648,.T.);
#14962=FACE_OUTER_BOUND('',#17649,.T.);
#14963=FACE_OUTER_BOUND('',#17650,.T.);
#14964=FACE_OUTER_BOUND('',#17651,.T.);
#14965=FACE_OUTER_BOUND('',#17652,.T.);
#14966=FACE_OUTER_BOUND('',#17653,.T.);
#14967=FACE_OUTER_BOUND('',#17654,.T.);
#14968=FACE_OUTER_BOUND('',#17655,.T.);
#14969=FACE_OUTER_BOUND('',#17656,.T.);
#14970=FACE_OUTER_BOUND('',#17657,.T.);
#14971=FACE_OUTER_BOUND('',#17658,.T.);
#14972=FACE_OUTER_BOUND('',#17659,.T.);
#14973=FACE_OUTER_BOUND('',#17660,.T.);
#14974=FACE_OUTER_BOUND('',#17661,.T.);
#14975=FACE_OUTER_BOUND('',#17662,.T.);
#14976=FACE_OUTER_BOUND('',#17663,.T.);
#14977=FACE_OUTER_BOUND('',#17664,.T.);
#14978=FACE_OUTER_BOUND('',#17665,.T.);
#14979=FACE_OUTER_BOUND('',#17666,.T.);
#14980=FACE_OUTER_BOUND('',#17667,.T.);
#14981=FACE_OUTER_BOUND('',#17668,.T.);
#14982=FACE_OUTER_BOUND('',#17669,.T.);
#14983=FACE_OUTER_BOUND('',#17670,.T.);
#14984=FACE_OUTER_BOUND('',#17671,.T.);
#14985=FACE_OUTER_BOUND('',#17672,.T.);
#14986=FACE_OUTER_BOUND('',#17674,.T.);
#14987=FACE_OUTER_BOUND('',#17675,.T.);
#14988=FACE_OUTER_BOUND('',#17676,.T.);
#14989=FACE_OUTER_BOUND('',#17678,.T.);
#14990=FACE_OUTER_BOUND('',#17679,.T.);
#14991=FACE_OUTER_BOUND('',#17680,.T.);
#14992=FACE_OUTER_BOUND('',#17681,.T.);
#14993=FACE_OUTER_BOUND('',#17682,.T.);
#14994=FACE_OUTER_BOUND('',#17683,.T.);
#14995=FACE_OUTER_BOUND('',#17684,.T.);
#14996=FACE_OUTER_BOUND('',#17685,.T.);
#14997=FACE_OUTER_BOUND('',#17687,.T.);
#14998=FACE_OUTER_BOUND('',#17689,.T.);
#14999=FACE_OUTER_BOUND('',#17691,.T.);
#17321=EDGE_LOOP('',(#41203,#41204,#41205,#41206,#41207,#41208));
#17322=EDGE_LOOP('',(#41209,#41210,#41211,#41212,#41213,#41214));
#17323=EDGE_LOOP('',(#41215,#41216,#41217,#41218));
#17324=EDGE_LOOP('',(#41219,#41220,#41221,#41222));
#17325=EDGE_LOOP('',(#41223,#41224,#41225,#41226,#41227,#41228,#41229,#41230,
#41231,#41232,#41233,#41234,#41235,#41236,#41237,#41238,#41239,#41240,#41241,
#41242,#41243,#41244,#41245,#41246,#41247,#41248,#41249,#41250,#41251,#41252,
#41253,#41254,#41255,#41256,#41257,#41258,#41259,#41260,#41261,#41262,#41263,
#41264,#41265,#41266,#41267,#41268,#41269,#41270));
#17326=EDGE_LOOP('',(#41271,#41272,#41273,#41274,#41275,#41276,#41277,#41278,
#41279,#41280,#41281,#41282));
#17327=EDGE_LOOP('',(#41283));
#17328=EDGE_LOOP('',(#41284,#41285,#41286,#41287,#41288,#41289,#41290,#41291,
#41292,#41293,#41294,#41295,#41296,#41297,#41298,#41299,#41300,#41301,#41302,
#41303,#41304,#41305,#41306,#41307,#41308,#41309,#41310,#41311,#41312,#41313,
#41314,#41315,#41316,#41317,#41318,#41319,#41320,#41321,#41322,#41323,#41324,
#41325,#41326,#41327,#41328,#41329,#41330,#41331));
#17329=EDGE_LOOP('',(#41332,#41333,#41334,#41335,#41336,#41337,#41338,#41339,
#41340,#41341,#41342,#41343,#41344,#41345,#41346,#41347,#41348,#41349,#41350,
#41351,#41352,#41353,#41354,#41355,#41356,#41357,#41358,#41359,#41360,#41361,
#41362,#41363,#41364,#41365,#41366,#41367,#41368,#41369,#41370,#41371,#41372,
#41373,#41374,#41375,#41376,#41377,#41378,#41379));
#17330=EDGE_LOOP('',(#41380,#41381,#41382,#41383,#41384,#41385));
#17331=EDGE_LOOP('',(#41386,#41387,#41388,#41389,#41390,#41391));
#17332=EDGE_LOOP('',(#41392,#41393,#41394,#41395));
#17333=EDGE_LOOP('',(#41396,#41397,#41398,#41399,#41400,#41401,#41402,#41403,
#41404,#41405,#41406,#41407,#41408,#41409,#41410,#41411,#41412,#41413,#41414,
#41415,#41416,#41417,#41418,#41419,#41420,#41421,#41422,#41423,#41424,#41425,
#41426,#41427,#41428,#41429,#41430,#41431,#41432,#41433,#41434,#41435,#41436,
#41437,#41438,#41439,#41440,#41441,#41442,#41443));
#17334=EDGE_LOOP('',(#41444,#41445,#41446,#41447,#41448,#41449,#41450,#41451,
#41452,#41453,#41454,#41455,#41456,#41457,#41458,#41459,#41460,#41461,#41462,
#41463,#41464,#41465,#41466,#41467,#41468,#41469,#41470,#41471,#41472,#41473,
#41474,#41475,#41476,#41477,#41478,#41479,#41480,#41481,#41482,#41483,#41484,
#41485,#41486,#41487,#41488,#41489,#41490,#41491));
#17335=EDGE_LOOP('',(#41492,#41493,#41494,#41495));
#17336=EDGE_LOOP('',(#41496,#41497,#41498,#41499,#41500,#41501,#41502,#41503,
#41504,#41505,#41506,#41507,#41508,#41509,#41510,#41511,#41512,#41513,#41514,
#41515,#41516,#41517,#41518,#41519,#41520,#41521,#41522,#41523,#41524,#41525,
#41526,#41527,#41528,#41529,#41530,#41531,#41532,#41533,#41534,#41535,#41536,
#41537,#41538,#41539,#41540,#41541,#41542,#41543));
#17337=EDGE_LOOP('',(#41544,#41545,#41546,#41547,#41548,#41549));
#17338=EDGE_LOOP('',(#41550,#41551,#41552,#41553,#41554,#41555));
#17339=EDGE_LOOP('',(#41556,#41557,#41558,#41559));
#17340=EDGE_LOOP('',(#41560,#41561,#41562,#41563));
#17341=EDGE_LOOP('',(#41564,#41565,#41566,#41567));
#17342=EDGE_LOOP('',(#41568,#41569,#41570,#41571));
#17343=EDGE_LOOP('',(#41572,#41573,#41574,#41575));
#17344=EDGE_LOOP('',(#41576,#41577,#41578,#41579));
#17345=EDGE_LOOP('',(#41580,#41581,#41582,#41583));
#17346=EDGE_LOOP('',(#41584,#41585,#41586,#41587));
#17347=EDGE_LOOP('',(#41588,#41589,#41590,#41591));
#17348=EDGE_LOOP('',(#41592,#41593,#41594,#41595));
#17349=EDGE_LOOP('',(#41596,#41597,#41598,#41599));
#17350=EDGE_LOOP('',(#41600,#41601,#41602,#41603));
#17351=EDGE_LOOP('',(#41604,#41605,#41606,#41607));
#17352=EDGE_LOOP('',(#41608,#41609,#41610,#41611));
#17353=EDGE_LOOP('',(#41612,#41613,#41614,#41615));
#17354=EDGE_LOOP('',(#41616,#41617,#41618,#41619));
#17355=EDGE_LOOP('',(#41620,#41621,#41622,#41623));
#17356=EDGE_LOOP('',(#41624,#41625,#41626,#41627));
#17357=EDGE_LOOP('',(#41628,#41629,#41630,#41631));
#17358=EDGE_LOOP('',(#41632,#41633,#41634,#41635));
#17359=EDGE_LOOP('',(#41636,#41637,#41638,#41639));
#17360=EDGE_LOOP('',(#41640,#41641,#41642,#41643));
#17361=EDGE_LOOP('',(#41644,#41645,#41646,#41647));
#17362=EDGE_LOOP('',(#41648,#41649,#41650,#41651));
#17363=EDGE_LOOP('',(#41652,#41653,#41654,#41655));
#17364=EDGE_LOOP('',(#41656,#41657,#41658,#41659));
#17365=EDGE_LOOP('',(#41660,#41661,#41662,#41663));
#17366=EDGE_LOOP('',(#41664,#41665,#41666,#41667));
#17367=EDGE_LOOP('',(#41668,#41669,#41670,#41671));
#17368=EDGE_LOOP('',(#41672,#41673,#41674,#41675));
#17369=EDGE_LOOP('',(#41676,#41677,#41678,#41679));
#17370=EDGE_LOOP('',(#41680,#41681,#41682,#41683));
#17371=EDGE_LOOP('',(#41684,#41685,#41686,#41687));
#17372=EDGE_LOOP('',(#41688,#41689,#41690,#41691));
#17373=EDGE_LOOP('',(#41692,#41693,#41694,#41695));
#17374=EDGE_LOOP('',(#41696,#41697,#41698,#41699,#41700,#41701,#41702,#41703,
#41704,#41705));
#17375=EDGE_LOOP('',(#41706,#41707,#41708,#41709));
#17376=EDGE_LOOP('',(#41710,#41711,#41712,#41713,#41714,#41715,#41716,#41717,
#41718,#41719));
#17377=EDGE_LOOP('',(#41720,#41721,#41722,#41723));
#17378=EDGE_LOOP('',(#41724,#41725,#41726,#41727,#41728,#41729,#41730,#41731,
#41732,#41733));
#17379=EDGE_LOOP('',(#41734,#41735,#41736,#41737));
#17380=EDGE_LOOP('',(#41738,#41739,#41740,#41741,#41742,#41743,#41744,#41745,
#41746,#41747));
#17381=EDGE_LOOP('',(#41748,#41749,#41750,#41751));
#17382=EDGE_LOOP('',(#41752,#41753,#41754,#41755,#41756,#41757,#41758,#41759,
#41760,#41761));
#17383=EDGE_LOOP('',(#41762,#41763,#41764,#41765));
#17384=EDGE_LOOP('',(#41766,#41767,#41768,#41769,#41770,#41771,#41772,#41773,
#41774,#41775));
#17385=EDGE_LOOP('',(#41776,#41777,#41778,#41779));
#17386=EDGE_LOOP('',(#41780,#41781,#41782,#41783,#41784,#41785,#41786,#41787,
#41788,#41789));
#17387=EDGE_LOOP('',(#41790,#41791,#41792,#41793));
#17388=EDGE_LOOP('',(#41794,#41795,#41796,#41797,#41798,#41799,#41800,#41801,
#41802,#41803));
#17389=EDGE_LOOP('',(#41804,#41805,#41806,#41807));
#17390=EDGE_LOOP('',(#41808,#41809,#41810,#41811,#41812,#41813,#41814,#41815,
#41816,#41817));
#17391=EDGE_LOOP('',(#41818,#41819,#41820,#41821));
#17392=EDGE_LOOP('',(#41822,#41823,#41824,#41825,#41826,#41827,#41828,#41829,
#41830,#41831));
#17393=EDGE_LOOP('',(#41832,#41833,#41834,#41835));
#17394=EDGE_LOOP('',(#41836,#41837,#41838,#41839,#41840,#41841,#41842,#41843,
#41844,#41845));
#17395=EDGE_LOOP('',(#41846,#41847,#41848,#41849));
#17396=EDGE_LOOP('',(#41850,#41851,#41852,#41853,#41854,#41855,#41856,#41857,
#41858,#41859));
#17397=EDGE_LOOP('',(#41860,#41861,#41862,#41863));
#17398=EDGE_LOOP('',(#41864,#41865,#41866,#41867,#41868,#41869,#41870,#41871,
#41872,#41873));
#17399=EDGE_LOOP('',(#41874,#41875,#41876,#41877));
#17400=EDGE_LOOP('',(#41878,#41879,#41880,#41881,#41882,#41883,#41884,#41885,
#41886,#41887));
#17401=EDGE_LOOP('',(#41888,#41889,#41890,#41891));
#17402=EDGE_LOOP('',(#41892,#41893,#41894,#41895,#41896,#41897,#41898,#41899,
#41900,#41901));
#17403=EDGE_LOOP('',(#41902,#41903,#41904,#41905));
#17404=EDGE_LOOP('',(#41906,#41907,#41908,#41909,#41910,#41911,#41912,#41913,
#41914,#41915));
#17405=EDGE_LOOP('',(#41916,#41917,#41918,#41919));
#17406=EDGE_LOOP('',(#41920,#41921,#41922,#41923,#41924,#41925,#41926,#41927,
#41928,#41929));
#17407=EDGE_LOOP('',(#41930,#41931,#41932,#41933));
#17408=EDGE_LOOP('',(#41934,#41935,#41936,#41937,#41938,#41939,#41940,#41941,
#41942,#41943));
#17409=EDGE_LOOP('',(#41944,#41945,#41946,#41947));
#17410=EDGE_LOOP('',(#41948,#41949,#41950,#41951,#41952,#41953,#41954,#41955,
#41956,#41957));
#17411=EDGE_LOOP('',(#41958,#41959,#41960,#41961));
#17412=EDGE_LOOP('',(#41962,#41963,#41964,#41965,#41966,#41967,#41968,#41969,
#41970,#41971));
#17413=EDGE_LOOP('',(#41972,#41973,#41974,#41975));
#17414=EDGE_LOOP('',(#41976,#41977,#41978,#41979,#41980,#41981,#41982,#41983,
#41984,#41985));
#17415=EDGE_LOOP('',(#41986,#41987,#41988,#41989));
#17416=EDGE_LOOP('',(#41990,#41991,#41992,#41993,#41994,#41995,#41996,#41997,
#41998,#41999));
#17417=EDGE_LOOP('',(#42000,#42001,#42002,#42003));
#17418=EDGE_LOOP('',(#42004,#42005,#42006,#42007,#42008,#42009,#42010,#42011,
#42012,#42013));
#17419=EDGE_LOOP('',(#42014,#42015,#42016,#42017));
#17420=EDGE_LOOP('',(#42018,#42019,#42020,#42021,#42022,#42023,#42024,#42025,
#42026,#42027));
#17421=EDGE_LOOP('',(#42028,#42029,#42030,#42031));
#17422=EDGE_LOOP('',(#42032,#42033,#42034,#42035,#42036,#42037,#42038,#42039,
#42040,#42041));
#17423=EDGE_LOOP('',(#42042,#42043,#42044,#42045));
#17424=EDGE_LOOP('',(#42046,#42047,#42048,#42049,#42050,#42051,#42052,#42053,
#42054,#42055));
#17425=EDGE_LOOP('',(#42056,#42057,#42058,#42059));
#17426=EDGE_LOOP('',(#42060,#42061,#42062,#42063,#42064,#42065,#42066,#42067,
#42068,#42069));
#17427=EDGE_LOOP('',(#42070,#42071,#42072,#42073));
#17428=EDGE_LOOP('',(#42074,#42075,#42076,#42077,#42078,#42079,#42080,#42081,
#42082,#42083));
#17429=EDGE_LOOP('',(#42084,#42085,#42086,#42087));
#17430=EDGE_LOOP('',(#42088,#42089,#42090,#42091,#42092,#42093,#42094,#42095,
#42096,#42097));
#17431=EDGE_LOOP('',(#42098,#42099,#42100,#42101));
#17432=EDGE_LOOP('',(#42102,#42103,#42104,#42105,#42106,#42107,#42108,#42109,
#42110,#42111));
#17433=EDGE_LOOP('',(#42112,#42113,#42114,#42115));
#17434=EDGE_LOOP('',(#42116,#42117,#42118,#42119,#42120,#42121,#42122,#42123,
#42124,#42125));
#17435=EDGE_LOOP('',(#42126,#42127,#42128,#42129));
#17436=EDGE_LOOP('',(#42130,#42131,#42132,#42133,#42134,#42135,#42136,#42137,
#42138,#42139));
#17437=EDGE_LOOP('',(#42140,#42141,#42142,#42143));
#17438=EDGE_LOOP('',(#42144,#42145,#42146,#42147,#42148,#42149,#42150,#42151,
#42152,#42153));
#17439=EDGE_LOOP('',(#42154,#42155,#42156,#42157));
#17440=EDGE_LOOP('',(#42158,#42159,#42160,#42161));
#17441=EDGE_LOOP('',(#42162,#42163,#42164,#42165));
#17442=EDGE_LOOP('',(#42166,#42167,#42168,#42169));
#17443=EDGE_LOOP('',(#42170,#42171,#42172,#42173));
#17444=EDGE_LOOP('',(#42174,#42175,#42176,#42177));
#17445=EDGE_LOOP('',(#42178,#42179,#42180,#42181));
#17446=EDGE_LOOP('',(#42182,#42183,#42184,#42185));
#17447=EDGE_LOOP('',(#42186,#42187,#42188,#42189));
#17448=EDGE_LOOP('',(#42190,#42191,#42192,#42193));
#17449=EDGE_LOOP('',(#42194,#42195,#42196,#42197));
#17450=EDGE_LOOP('',(#42198,#42199,#42200,#42201));
#17451=EDGE_LOOP('',(#42202,#42203,#42204,#42205));
#17452=EDGE_LOOP('',(#42206,#42207,#42208,#42209));
#17453=EDGE_LOOP('',(#42210,#42211,#42212,#42213));
#17454=EDGE_LOOP('',(#42214,#42215,#42216,#42217));
#17455=EDGE_LOOP('',(#42218,#42219,#42220,#42221));
#17456=EDGE_LOOP('',(#42222,#42223,#42224,#42225));
#17457=EDGE_LOOP('',(#42226,#42227,#42228,#42229));
#17458=EDGE_LOOP('',(#42230,#42231,#42232,#42233));
#17459=EDGE_LOOP('',(#42234,#42235,#42236,#42237));
#17460=EDGE_LOOP('',(#42238,#42239,#42240,#42241));
#17461=EDGE_LOOP('',(#42242,#42243,#42244,#42245));
#17462=EDGE_LOOP('',(#42246,#42247,#42248,#42249));
#17463=EDGE_LOOP('',(#42250,#42251,#42252,#42253));
#17464=EDGE_LOOP('',(#42254,#42255,#42256,#42257));
#17465=EDGE_LOOP('',(#42258,#42259,#42260,#42261));
#17466=EDGE_LOOP('',(#42262,#42263,#42264,#42265));
#17467=EDGE_LOOP('',(#42266,#42267,#42268,#42269));
#17468=EDGE_LOOP('',(#42270,#42271,#42272,#42273));
#17469=EDGE_LOOP('',(#42274,#42275,#42276,#42277));
#17470=EDGE_LOOP('',(#42278,#42279,#42280,#42281));
#17471=EDGE_LOOP('',(#42282,#42283,#42284,#42285));
#17472=EDGE_LOOP('',(#42286,#42287,#42288,#42289));
#17473=EDGE_LOOP('',(#42290,#42291,#42292,#42293,#42294,#42295,#42296,#42297,
#42298,#42299));
#17474=EDGE_LOOP('',(#42300,#42301,#42302,#42303,#42304,#42305,#42306,#42307,
#42308,#42309));
#17475=EDGE_LOOP('',(#42310,#42311,#42312,#42313,#42314,#42315,#42316,#42317,
#42318,#42319));
#17476=EDGE_LOOP('',(#42320,#42321,#42322,#42323,#42324,#42325,#42326,#42327,
#42328,#42329));
#17477=EDGE_LOOP('',(#42330,#42331,#42332,#42333,#42334,#42335,#42336,#42337,
#42338,#42339));
#17478=EDGE_LOOP('',(#42340,#42341,#42342,#42343,#42344,#42345,#42346,#42347,
#42348,#42349));
#17479=EDGE_LOOP('',(#42350,#42351,#42352,#42353,#42354,#42355,#42356,#42357,
#42358,#42359));
#17480=EDGE_LOOP('',(#42360,#42361,#42362,#42363,#42364,#42365,#42366,#42367,
#42368,#42369));
#17481=EDGE_LOOP('',(#42370,#42371,#42372,#42373,#42374,#42375,#42376,#42377,
#42378,#42379));
#17482=EDGE_LOOP('',(#42380,#42381,#42382,#42383,#42384,#42385,#42386,#42387,
#42388,#42389));
#17483=EDGE_LOOP('',(#42390,#42391,#42392,#42393,#42394,#42395,#42396,#42397,
#42398,#42399));
#17484=EDGE_LOOP('',(#42400,#42401,#42402,#42403,#42404,#42405,#42406,#42407,
#42408,#42409));
#17485=EDGE_LOOP('',(#42410,#42411,#42412,#42413,#42414,#42415,#42416,#42417,
#42418,#42419));
#17486=EDGE_LOOP('',(#42420,#42421,#42422,#42423,#42424,#42425,#42426,#42427,
#42428,#42429));
#17487=EDGE_LOOP('',(#42430,#42431,#42432,#42433,#42434,#42435,#42436,#42437,
#42438,#42439));
#17488=EDGE_LOOP('',(#42440,#42441,#42442,#42443,#42444,#42445,#42446,#42447,
#42448,#42449));
#17489=EDGE_LOOP('',(#42450,#42451,#42452,#42453,#42454,#42455,#42456,#42457,
#42458,#42459));
#17490=EDGE_LOOP('',(#42460,#42461,#42462,#42463,#42464,#42465,#42466,#42467,
#42468,#42469));
#17491=EDGE_LOOP('',(#42470,#42471,#42472,#42473,#42474,#42475,#42476,#42477,
#42478,#42479));
#17492=EDGE_LOOP('',(#42480,#42481,#42482,#42483,#42484,#42485,#42486,#42487,
#42488,#42489));
#17493=EDGE_LOOP('',(#42490,#42491,#42492,#42493,#42494,#42495,#42496,#42497,
#42498,#42499));
#17494=EDGE_LOOP('',(#42500,#42501,#42502,#42503,#42504,#42505,#42506,#42507,
#42508,#42509));
#17495=EDGE_LOOP('',(#42510,#42511,#42512,#42513,#42514,#42515,#42516,#42517,
#42518,#42519));
#17496=EDGE_LOOP('',(#42520,#42521,#42522,#42523,#42524,#42525,#42526,#42527,
#42528,#42529));
#17497=EDGE_LOOP('',(#42530,#42531,#42532,#42533,#42534,#42535,#42536,#42537,
#42538,#42539));
#17498=EDGE_LOOP('',(#42540,#42541,#42542,#42543,#42544,#42545,#42546,#42547,
#42548,#42549));
#17499=EDGE_LOOP('',(#42550,#42551,#42552,#42553,#42554,#42555,#42556,#42557,
#42558,#42559));
#17500=EDGE_LOOP('',(#42560,#42561,#42562,#42563,#42564,#42565,#42566,#42567,
#42568,#42569));
#17501=EDGE_LOOP('',(#42570,#42571,#42572,#42573,#42574,#42575,#42576,#42577,
#42578,#42579));
#17502=EDGE_LOOP('',(#42580,#42581,#42582,#42583,#42584,#42585,#42586,#42587,
#42588,#42589));
#17503=EDGE_LOOP('',(#42590,#42591,#42592,#42593,#42594,#42595,#42596,#42597,
#42598,#42599));
#17504=EDGE_LOOP('',(#42600,#42601,#42602,#42603,#42604,#42605,#42606,#42607,
#42608,#42609));
#17505=EDGE_LOOP('',(#42610,#42611,#42612,#42613,#42614,#42615,#42616,#42617,
#42618,#42619));
#17506=EDGE_LOOP('',(#42620,#42621,#42622,#42623));
#17507=EDGE_LOOP('',(#42624,#42625,#42626,#42627));
#17508=EDGE_LOOP('',(#42628,#42629,#42630,#42631));
#17509=EDGE_LOOP('',(#42632,#42633,#42634,#42635));
#17510=EDGE_LOOP('',(#42636,#42637,#42638,#42639));
#17511=EDGE_LOOP('',(#42640,#42641,#42642,#42643));
#17512=EDGE_LOOP('',(#42644,#42645,#42646,#42647));
#17513=EDGE_LOOP('',(#42648,#42649,#42650,#42651));
#17514=EDGE_LOOP('',(#42652,#42653,#42654,#42655));
#17515=EDGE_LOOP('',(#42656,#42657,#42658,#42659));
#17516=EDGE_LOOP('',(#42660,#42661,#42662,#42663));
#17517=EDGE_LOOP('',(#42664,#42665,#42666,#42667));
#17518=EDGE_LOOP('',(#42668,#42669,#42670,#42671));
#17519=EDGE_LOOP('',(#42672,#42673,#42674,#42675));
#17520=EDGE_LOOP('',(#42676,#42677,#42678,#42679));
#17521=EDGE_LOOP('',(#42680,#42681,#42682,#42683));
#17522=EDGE_LOOP('',(#42684,#42685,#42686,#42687));
#17523=EDGE_LOOP('',(#42688,#42689,#42690,#42691));
#17524=EDGE_LOOP('',(#42692,#42693,#42694,#42695));
#17525=EDGE_LOOP('',(#42696,#42697,#42698,#42699));
#17526=EDGE_LOOP('',(#42700,#42701,#42702,#42703));
#17527=EDGE_LOOP('',(#42704,#42705,#42706,#42707));
#17528=EDGE_LOOP('',(#42708,#42709,#42710,#42711));
#17529=EDGE_LOOP('',(#42712,#42713,#42714,#42715));
#17530=EDGE_LOOP('',(#42716,#42717,#42718,#42719));
#17531=EDGE_LOOP('',(#42720,#42721,#42722,#42723));
#17532=EDGE_LOOP('',(#42724,#42725,#42726,#42727));
#17533=EDGE_LOOP('',(#42728,#42729,#42730,#42731));
#17534=EDGE_LOOP('',(#42732,#42733,#42734,#42735));
#17535=EDGE_LOOP('',(#42736,#42737,#42738,#42739));
#17536=EDGE_LOOP('',(#42740,#42741,#42742,#42743));
#17537=EDGE_LOOP('',(#42744,#42745,#42746,#42747));
#17538=EDGE_LOOP('',(#42748,#42749,#42750,#42751));
#17539=EDGE_LOOP('',(#42752,#42753,#42754,#42755));
#17540=EDGE_LOOP('',(#42756,#42757,#42758,#42759));
#17541=EDGE_LOOP('',(#42760,#42761,#42762,#42763));
#17542=EDGE_LOOP('',(#42764,#42765,#42766,#42767));
#17543=EDGE_LOOP('',(#42768,#42769,#42770,#42771));
#17544=EDGE_LOOP('',(#42772,#42773,#42774,#42775));
#17545=EDGE_LOOP('',(#42776,#42777,#42778,#42779));
#17546=EDGE_LOOP('',(#42780,#42781,#42782,#42783));
#17547=EDGE_LOOP('',(#42784,#42785,#42786,#42787));
#17548=EDGE_LOOP('',(#42788,#42789,#42790,#42791));
#17549=EDGE_LOOP('',(#42792,#42793,#42794,#42795));
#17550=EDGE_LOOP('',(#42796,#42797,#42798,#42799));
#17551=EDGE_LOOP('',(#42800,#42801,#42802,#42803));
#17552=EDGE_LOOP('',(#42804,#42805,#42806,#42807));
#17553=EDGE_LOOP('',(#42808,#42809,#42810,#42811));
#17554=EDGE_LOOP('',(#42812,#42813,#42814,#42815));
#17555=EDGE_LOOP('',(#42816,#42817,#42818,#42819));
#17556=EDGE_LOOP('',(#42820,#42821,#42822,#42823));
#17557=EDGE_LOOP('',(#42824,#42825,#42826,#42827));
#17558=EDGE_LOOP('',(#42828,#42829,#42830,#42831));
#17559=EDGE_LOOP('',(#42832,#42833,#42834,#42835));
#17560=EDGE_LOOP('',(#42836,#42837,#42838,#42839));
#17561=EDGE_LOOP('',(#42840,#42841,#42842,#42843));
#17562=EDGE_LOOP('',(#42844,#42845,#42846,#42847));
#17563=EDGE_LOOP('',(#42848,#42849,#42850,#42851));
#17564=EDGE_LOOP('',(#42852,#42853,#42854,#42855));
#17565=EDGE_LOOP('',(#42856,#42857,#42858,#42859));
#17566=EDGE_LOOP('',(#42860,#42861,#42862,#42863));
#17567=EDGE_LOOP('',(#42864,#42865,#42866,#42867));
#17568=EDGE_LOOP('',(#42868,#42869,#42870,#42871));
#17569=EDGE_LOOP('',(#42872,#42873,#42874,#42875));
#17570=EDGE_LOOP('',(#42876,#42877,#42878,#42879));
#17571=EDGE_LOOP('',(#42880,#42881,#42882,#42883));
#17572=EDGE_LOOP('',(#42884,#42885,#42886,#42887));
#17573=EDGE_LOOP('',(#42888,#42889,#42890,#42891));
#17574=EDGE_LOOP('',(#42892,#42893,#42894,#42895));
#17575=EDGE_LOOP('',(#42896,#42897,#42898,#42899));
#17576=EDGE_LOOP('',(#42900,#42901,#42902,#42903));
#17577=EDGE_LOOP('',(#42904,#42905,#42906,#42907));
#17578=EDGE_LOOP('',(#42908,#42909,#42910,#42911));
#17579=EDGE_LOOP('',(#42912,#42913,#42914,#42915));
#17580=EDGE_LOOP('',(#42916,#42917,#42918,#42919));
#17581=EDGE_LOOP('',(#42920,#42921,#42922,#42923));
#17582=EDGE_LOOP('',(#42924,#42925,#42926,#42927));
#17583=EDGE_LOOP('',(#42928,#42929,#42930,#42931));
#17584=EDGE_LOOP('',(#42932,#42933,#42934,#42935));
#17585=EDGE_LOOP('',(#42936,#42937,#42938,#42939));
#17586=EDGE_LOOP('',(#42940,#42941,#42942,#42943));
#17587=EDGE_LOOP('',(#42944,#42945,#42946,#42947));
#17588=EDGE_LOOP('',(#42948,#42949,#42950,#42951));
#17589=EDGE_LOOP('',(#42952,#42953,#42954,#42955));
#17590=EDGE_LOOP('',(#42956,#42957,#42958,#42959));
#17591=EDGE_LOOP('',(#42960,#42961,#42962,#42963));
#17592=EDGE_LOOP('',(#42964,#42965,#42966,#42967));
#17593=EDGE_LOOP('',(#42968,#42969,#42970,#42971));
#17594=EDGE_LOOP('',(#42972,#42973,#42974,#42975));
#17595=EDGE_LOOP('',(#42976,#42977,#42978,#42979));
#17596=EDGE_LOOP('',(#42980,#42981,#42982,#42983));
#17597=EDGE_LOOP('',(#42984,#42985,#42986,#42987));
#17598=EDGE_LOOP('',(#42988,#42989,#42990,#42991));
#17599=EDGE_LOOP('',(#42992,#42993,#42994,#42995));
#17600=EDGE_LOOP('',(#42996,#42997,#42998,#42999));
#17601=EDGE_LOOP('',(#43000,#43001,#43002,#43003));
#17602=EDGE_LOOP('',(#43004,#43005,#43006,#43007));
#17603=EDGE_LOOP('',(#43008,#43009,#43010,#43011));
#17604=EDGE_LOOP('',(#43012,#43013,#43014,#43015));
#17605=EDGE_LOOP('',(#43016,#43017,#43018,#43019));
#17606=EDGE_LOOP('',(#43020,#43021,#43022,#43023));
#17607=EDGE_LOOP('',(#43024,#43025,#43026,#43027));
#17608=EDGE_LOOP('',(#43028,#43029,#43030,#43031));
#17609=EDGE_LOOP('',(#43032,#43033,#43034,#43035));
#17610=EDGE_LOOP('',(#43036,#43037,#43038,#43039));
#17611=EDGE_LOOP('',(#43040,#43041,#43042,#43043));
#17612=EDGE_LOOP('',(#43044,#43045,#43046,#43047));
#17613=EDGE_LOOP('',(#43048,#43049,#43050,#43051));
#17614=EDGE_LOOP('',(#43052,#43053,#43054,#43055));
#17615=EDGE_LOOP('',(#43056,#43057,#43058,#43059));
#17616=EDGE_LOOP('',(#43060,#43061,#43062,#43063));
#17617=EDGE_LOOP('',(#43064,#43065,#43066,#43067));
#17618=EDGE_LOOP('',(#43068,#43069,#43070,#43071));
#17619=EDGE_LOOP('',(#43072,#43073,#43074,#43075));
#17620=EDGE_LOOP('',(#43076,#43077,#43078,#43079));
#17621=EDGE_LOOP('',(#43080,#43081,#43082,#43083));
#17622=EDGE_LOOP('',(#43084,#43085,#43086,#43087));
#17623=EDGE_LOOP('',(#43088,#43089,#43090,#43091));
#17624=EDGE_LOOP('',(#43092,#43093,#43094,#43095));
#17625=EDGE_LOOP('',(#43096,#43097,#43098,#43099));
#17626=EDGE_LOOP('',(#43100,#43101,#43102,#43103));
#17627=EDGE_LOOP('',(#43104,#43105,#43106,#43107));
#17628=EDGE_LOOP('',(#43108,#43109,#43110,#43111));
#17629=EDGE_LOOP('',(#43112,#43113,#43114,#43115));
#17630=EDGE_LOOP('',(#43116,#43117,#43118,#43119));
#17631=EDGE_LOOP('',(#43120,#43121,#43122,#43123));
#17632=EDGE_LOOP('',(#43124,#43125,#43126,#43127));
#17633=EDGE_LOOP('',(#43128,#43129,#43130,#43131));
#17634=EDGE_LOOP('',(#43132,#43133,#43134,#43135));
#17635=EDGE_LOOP('',(#43136,#43137,#43138,#43139));
#17636=EDGE_LOOP('',(#43140,#43141,#43142,#43143));
#17637=EDGE_LOOP('',(#43144,#43145,#43146,#43147));
#17638=EDGE_LOOP('',(#43148,#43149,#43150,#43151));
#17639=EDGE_LOOP('',(#43152,#43153,#43154,#43155));
#17640=EDGE_LOOP('',(#43156,#43157,#43158,#43159));
#17641=EDGE_LOOP('',(#43160,#43161,#43162,#43163));
#17642=EDGE_LOOP('',(#43164,#43165,#43166,#43167));
#17643=EDGE_LOOP('',(#43168,#43169,#43170,#43171));
#17644=EDGE_LOOP('',(#43172,#43173,#43174,#43175));
#17645=EDGE_LOOP('',(#43176,#43177,#43178,#43179));
#17646=EDGE_LOOP('',(#43180,#43181,#43182,#43183));
#17647=EDGE_LOOP('',(#43184,#43185,#43186,#43187));
#17648=EDGE_LOOP('',(#43188,#43189,#43190,#43191));
#17649=EDGE_LOOP('',(#43192,#43193,#43194,#43195));
#17650=EDGE_LOOP('',(#43196,#43197,#43198,#43199));
#17651=EDGE_LOOP('',(#43200,#43201,#43202,#43203));
#17652=EDGE_LOOP('',(#43204,#43205,#43206,#43207));
#17653=EDGE_LOOP('',(#43208,#43209,#43210,#43211));
#17654=EDGE_LOOP('',(#43212,#43213,#43214,#43215));
#17655=EDGE_LOOP('',(#43216,#43217,#43218,#43219));
#17656=EDGE_LOOP('',(#43220,#43221,#43222,#43223));
#17657=EDGE_LOOP('',(#43224,#43225,#43226,#43227));
#17658=EDGE_LOOP('',(#43228,#43229,#43230,#43231));
#17659=EDGE_LOOP('',(#43232,#43233,#43234,#43235));
#17660=EDGE_LOOP('',(#43236,#43237,#43238,#43239));
#17661=EDGE_LOOP('',(#43240,#43241,#43242,#43243));
#17662=EDGE_LOOP('',(#43244,#43245,#43246,#43247));
#17663=EDGE_LOOP('',(#43248,#43249,#43250,#43251));
#17664=EDGE_LOOP('',(#43252,#43253,#43254,#43255));
#17665=EDGE_LOOP('',(#43256,#43257,#43258,#43259));
#17666=EDGE_LOOP('',(#43260,#43261,#43262,#43263));
#17667=EDGE_LOOP('',(#43264,#43265,#43266,#43267));
#17668=EDGE_LOOP('',(#43268,#43269,#43270,#43271));
#17669=EDGE_LOOP('',(#43272,#43273,#43274,#43275));
#17670=EDGE_LOOP('',(#43276,#43277,#43278,#43279));
#17671=EDGE_LOOP('',(#43280,#43281,#43282,#43283,#43284));
#17672=EDGE_LOOP('',(#43285));
#17673=EDGE_LOOP('',(#43286));
#17674=EDGE_LOOP('',(#43287,#43288,#43289,#43290,#43291));
#17675=EDGE_LOOP('',(#43292,#43293,#43294,#43295,#43296));
#17676=EDGE_LOOP('',(#43297));
#17677=EDGE_LOOP('',(#43298));
#17678=EDGE_LOOP('',(#43299,#43300,#43301,#43302,#43303));
#17679=EDGE_LOOP('',(#43304,#43305,#43306,#43307,#43308));
#17680=EDGE_LOOP('',(#43309,#43310,#43311,#43312,#43313));
#17681=EDGE_LOOP('',(#43314,#43315,#43316,#43317,#43318));
#17682=EDGE_LOOP('',(#43319,#43320,#43321,#43322,#43323));
#17683=EDGE_LOOP('',(#43324,#43325,#43326,#43327));
#17684=EDGE_LOOP('',(#43328,#43329,#43330,#43331));
#17685=EDGE_LOOP('',(#43332));
#17686=EDGE_LOOP('',(#43333));
#17687=EDGE_LOOP('',(#43334,#43335,#43336,#43337,#43338,#43339,#43340,#43341,
#43342,#43343,#43344,#43345));
#17688=EDGE_LOOP('',(#43346));
#17689=EDGE_LOOP('',(#43347));
#17690=EDGE_LOOP('',(#43348));
#17691=EDGE_LOOP('',(#43349,#43350,#43351,#43352));
#19132=(
BOUNDED_CURVE()
B_SPLINE_CURVE(2,(#77420,#77421,#77422),.UNSPECIFIED.,.F.,.F.)
B_SPLINE_CURVE_WITH_KNOTS((3,3),(0.,0.0709397118056797),.UNSPECIFIED.)
CURVE()
GEOMETRIC_REPRESENTATION_ITEM()
RATIONAL_B_SPLINE_CURVE((1.,1.00002244954425,1.))
REPRESENTATION_ITEM('')
);
#19133=(
BOUNDED_CURVE()
B_SPLINE_CURVE(2,(#77430,#77431,#77432),.UNSPECIFIED.,.F.,.F.)
B_SPLINE_CURVE_WITH_KNOTS((3,3),(0.,0.0709397118056795),.UNSPECIFIED.)
CURVE()
GEOMETRIC_REPRESENTATION_ITEM()
RATIONAL_B_SPLINE_CURVE((1.,1.00002245192274,1.))
REPRESENTATION_ITEM('')
);
#19134=(
BOUNDED_CURVE()
B_SPLINE_CURVE(2,(#77437,#77438,#77439),.UNSPECIFIED.,.F.,.F.)
B_SPLINE_CURVE_WITH_KNOTS((3,3),(0.,0.0709397118056794),.UNSPECIFIED.)
CURVE()
GEOMETRIC_REPRESENTATION_ITEM()
RATIONAL_B_SPLINE_CURVE((1.,1.00002245169207,1.))
REPRESENTATION_ITEM('')
);
#19135=(
BOUNDED_CURVE()
B_SPLINE_CURVE(2,(#77443,#77444,#77445),.UNSPECIFIED.,.F.,.F.)
B_SPLINE_CURVE_WITH_KNOTS((3,3),(0.,0.0709397118056792),.UNSPECIFIED.)
CURVE()
GEOMETRIC_REPRESENTATION_ITEM()
RATIONAL_B_SPLINE_CURVE((1.,1.00002245215096,1.))
REPRESENTATION_ITEM('')
);
#19136=(
BOUNDED_CURVE()
B_SPLINE_CURVE(2,(#77464,#77465,#77466),.UNSPECIFIED.,.F.,.F.)
B_SPLINE_CURVE_WITH_KNOTS((3,3),(0.,0.0709397118056795),.UNSPECIFIED.)
CURVE()
GEOMETRIC_REPRESENTATION_ITEM()
RATIONAL_B_SPLINE_CURVE((1.,1.00002245040396,1.))
REPRESENTATION_ITEM('')
);
#19137=(
BOUNDED_CURVE()
B_SPLINE_CURVE(2,(#77470,#77471,#77472),.UNSPECIFIED.,.F.,.F.)
B_SPLINE_CURVE_WITH_KNOTS((3,3),(0.,0.0424100228697519),.UNSPECIFIED.)
CURVE()
GEOMETRIC_REPRESENTATION_ITEM()
RATIONAL_B_SPLINE_CURVE((1.,1.00001338511468,1.0000107512927))
REPRESENTATION_ITEM('')
);
#19138=(
BOUNDED_CURVE()
B_SPLINE_CURVE(2,(#77474,#77475,#77476),.UNSPECIFIED.,.F.,.F.)
B_SPLINE_CURVE_WITH_KNOTS((3,3),(0.339146964126514,0.668418076018302),
 .UNSPECIFIED.)
CURVE()
GEOMETRIC_REPRESENTATION_ITEM()
RATIONAL_B_SPLINE_CURVE((1.00400190544534,1.00495889669788,1.00400190544534))
REPRESENTATION_ITEM('')
);
#19139=(
BOUNDED_CURVE()
B_SPLINE_CURVE(2,(#77478,#77479,#77480),.UNSPECIFIED.,.F.,.F.)
B_SPLINE_CURVE_WITH_KNOTS((3,3),(0.0284639715386128,0.07087399516029),
 .UNSPECIFIED.)
CURVE()
GEOMETRIC_REPRESENTATION_ITEM()
RATIONAL_B_SPLINE_CURVE((1.00001075071627,1.00001338439739,1.))
REPRESENTATION_ITEM('')
);
#19140=(
BOUNDED_CURVE()
B_SPLINE_CURVE(2,(#77484,#77485,#77486),.UNSPECIFIED.,.F.,.F.)
B_SPLINE_CURVE_WITH_KNOTS((3,3),(0.,0.0424100228448336),.UNSPECIFIED.)
CURVE()
GEOMETRIC_REPRESENTATION_ITEM()
RATIONAL_B_SPLINE_CURVE((1.,1.00001338576537,1.00001075181536))
REPRESENTATION_ITEM('')
);
#19141=(
BOUNDED_CURVE()
B_SPLINE_CURVE(2,(#77488,#77489,#77490),.UNSPECIFIED.,.F.,.F.)
B_SPLINE_CURVE_WITH_KNOTS((3,3),(0.339146964126517,0.668418076018306),
 .UNSPECIFIED.)
CURVE()
GEOMETRIC_REPRESENTATION_ITEM()
RATIONAL_B_SPLINE_CURVE((1.00400190544534,1.00495889669788,1.00400190544534))
REPRESENTATION_ITEM('')
);
#19142=(
BOUNDED_CURVE()
B_SPLINE_CURVE(2,(#77492,#77493,#77494),.UNSPECIFIED.,.F.,.F.)
B_SPLINE_CURVE_WITH_KNOTS((3,3),(0.0284639718304313,0.0708739951602905),
 .UNSPECIFIED.)
CURVE()
GEOMETRIC_REPRESENTATION_ITEM()
RATIONAL_B_SPLINE_CURVE((1.00001075171905,1.00001338564569,1.))
REPRESENTATION_ITEM('')
);
#19143=(
BOUNDED_CURVE()
B_SPLINE_CURVE(2,(#77498,#77499,#77500),.UNSPECIFIED.,.F.,.F.)
B_SPLINE_CURVE_WITH_KNOTS((3,3),(0.,0.0424100233232146),.UNSPECIFIED.)
CURVE()
GEOMETRIC_REPRESENTATION_ITEM()
RATIONAL_B_SPLINE_CURVE((1.,1.00001338411593,1.00001075049031))
REPRESENTATION_ITEM('')
);
#19144=(
BOUNDED_CURVE()
B_SPLINE_CURVE(2,(#77502,#77503,#77504),.UNSPECIFIED.,.F.,.F.)
B_SPLINE_CURVE_WITH_KNOTS((3,3),(0.339146964126517,0.668418076018303),
 .UNSPECIFIED.)
CURVE()
GEOMETRIC_REPRESENTATION_ITEM()
RATIONAL_B_SPLINE_CURVE((1.00400190544534,1.00495889669787,1.00400190544534))
REPRESENTATION_ITEM('')
);
#19145=(
BOUNDED_CURVE()
B_SPLINE_CURVE(2,(#77506,#77507,#77508),.UNSPECIFIED.,.F.,.F.)
B_SPLINE_CURVE_WITH_KNOTS((3,3),(0.0284639713681571,0.0708739951602903),
 .UNSPECIFIED.)
CURVE()
GEOMETRIC_REPRESENTATION_ITEM()
RATIONAL_B_SPLINE_CURVE((1.00001075037836,1.00001338397678,1.))
REPRESENTATION_ITEM('')
);
#19146=(
BOUNDED_CURVE()
B_SPLINE_CURVE(2,(#77512,#77513,#77514),.UNSPECIFIED.,.F.,.F.)
B_SPLINE_CURVE_WITH_KNOTS((3,3),(0.,0.0424100226311801),.UNSPECIFIED.)
CURVE()
GEOMETRIC_REPRESENTATION_ITEM()
RATIONAL_B_SPLINE_CURVE((1.,1.00001338548565,1.00001075159076))
REPRESENTATION_ITEM('')
);
#19147=(
BOUNDED_CURVE()
B_SPLINE_CURVE(2,(#77516,#77517,#77518),.UNSPECIFIED.,.F.,.F.)
B_SPLINE_CURVE_WITH_KNOTS((3,3),(0.339146964126518,0.668418076018302),
 .UNSPECIFIED.)
CURVE()
GEOMETRIC_REPRESENTATION_ITEM()
RATIONAL_B_SPLINE_CURVE((1.00400190544533,1.00495889669787,1.00400190544533))
REPRESENTATION_ITEM('')
);
#19148=(
BOUNDED_CURVE()
B_SPLINE_CURVE(2,(#77520,#77521,#77522),.UNSPECIFIED.,.F.,.F.)
B_SPLINE_CURVE_WITH_KNOTS((3,3),(0.0284639720100238,0.07087399516029),
 .UNSPECIFIED.)
CURVE()
GEOMETRIC_REPRESENTATION_ITEM()
RATIONAL_B_SPLINE_CURVE((1.00001075118356,1.00001338497894,1.))
REPRESENTATION_ITEM('')
);
#19149=(
BOUNDED_CURVE()
B_SPLINE_CURVE(2,(#77526,#77527,#77528),.UNSPECIFIED.,.F.,.F.)
B_SPLINE_CURVE_WITH_KNOTS((3,3),(0.,0.0424100230241298),.UNSPECIFIED.)
CURVE()
GEOMETRIC_REPRESENTATION_ITEM()
RATIONAL_B_SPLINE_CURVE((1.,1.00001338698316,1.00001075279346))
REPRESENTATION_ITEM('')
);
#19150=(
BOUNDED_CURVE()
B_SPLINE_CURVE(2,(#77530,#77531,#77532),.UNSPECIFIED.,.F.,.F.)
B_SPLINE_CURVE_WITH_KNOTS((3,3),(0.339146964126515,0.668418076018307),
 .UNSPECIFIED.)
CURVE()
GEOMETRIC_REPRESENTATION_ITEM()
RATIONAL_B_SPLINE_CURVE((1.00400190544536,1.0049588966979,1.00400190544536))
REPRESENTATION_ITEM('')
);
#19151=(
BOUNDED_CURVE()
B_SPLINE_CURVE(2,(#77534,#77535,#77536),.UNSPECIFIED.,.F.,.F.)
B_SPLINE_CURVE_WITH_KNOTS((3,3),(0.0284639721115161,0.0708739951602901),
 .UNSPECIFIED.)
CURVE()
GEOMETRIC_REPRESENTATION_ITEM()
RATIONAL_B_SPLINE_CURVE((1.00001075066776,1.00001338433673,1.))
REPRESENTATION_ITEM('')
);
#19152=(
BOUNDED_CURVE()
B_SPLINE_CURVE(2,(#77540,#77541,#77542),.UNSPECIFIED.,.F.,.F.)
B_SPLINE_CURVE_WITH_KNOTS((3,3),(0.,0.0424100237464711),.UNSPECIFIED.)
CURVE()
GEOMETRIC_REPRESENTATION_ITEM()
RATIONAL_B_SPLINE_CURVE((1.,1.00001338457639,1.00001075086))
REPRESENTATION_ITEM('')
);
#19153=(
BOUNDED_CURVE()
B_SPLINE_CURVE(2,(#77544,#77545,#77546),.UNSPECIFIED.,.F.,.F.)
B_SPLINE_CURVE_WITH_KNOTS((3,3),(0.339146964126521,0.668418076018307),
 .UNSPECIFIED.)
CURVE()
GEOMETRIC_REPRESENTATION_ITEM()
RATIONAL_B_SPLINE_CURVE((1.00400190544534,1.00495889669787,1.00400190544534))
REPRESENTATION_ITEM('')
);
#19154=(
BOUNDED_CURVE()
B_SPLINE_CURVE(2,(#77548,#77549,#77550),.UNSPECIFIED.,.F.,.F.)
B_SPLINE_CURVE_WITH_KNOTS((3,3),(0.0284639714302619,0.0708739951602905),
 .UNSPECIFIED.)
CURVE()
GEOMETRIC_REPRESENTATION_ITEM()
RATIONAL_B_SPLINE_CURVE((1.00001075131298,1.00001338514034,1.))
REPRESENTATION_ITEM('')
);
#19155=(
BOUNDED_CURVE()
B_SPLINE_CURVE(2,(#77554,#77555,#77556),.UNSPECIFIED.,.F.,.F.)
B_SPLINE_CURVE_WITH_KNOTS((3,3),(0.,0.0424100231669585),.UNSPECIFIED.)
CURVE()
GEOMETRIC_REPRESENTATION_ITEM()
RATIONAL_B_SPLINE_CURVE((1.,1.00001338549266,1.00001075159619))
REPRESENTATION_ITEM('')
);
#19156=(
BOUNDED_CURVE()
B_SPLINE_CURVE(2,(#77558,#77559,#77560),.UNSPECIFIED.,.F.,.F.)
B_SPLINE_CURVE_WITH_KNOTS((3,3),(0.339146964126509,0.668418076018305),
 .UNSPECIFIED.)
CURVE()
GEOMETRIC_REPRESENTATION_ITEM()
RATIONAL_B_SPLINE_CURVE((1.00400190544537,1.00495889669791,1.00400190544537))
REPRESENTATION_ITEM('')
);
#19157=(
BOUNDED_CURVE()
B_SPLINE_CURVE(2,(#77562,#77563,#77564),.UNSPECIFIED.,.F.,.F.)
B_SPLINE_CURVE_WITH_KNOTS((3,3),(0.0284639724895236,0.0708739951602903),
 .UNSPECIFIED.)
CURVE()
GEOMETRIC_REPRESENTATION_ITEM()
RATIONAL_B_SPLINE_CURVE((1.00001075242956,1.00001338652996,1.))
REPRESENTATION_ITEM('')
);
#19158=(
BOUNDED_CURVE()
B_SPLINE_CURVE(2,(#77568,#77569,#77570),.UNSPECIFIED.,.F.,.F.)
B_SPLINE_CURVE_WITH_KNOTS((3,3),(0.,0.0424100230945575),.UNSPECIFIED.)
CURVE()
GEOMETRIC_REPRESENTATION_ITEM()
RATIONAL_B_SPLINE_CURVE((1.,1.00001338444694,1.00001075075626))
REPRESENTATION_ITEM('')
);
#19159=(
BOUNDED_CURVE()
B_SPLINE_CURVE(2,(#77572,#77573,#77574),.UNSPECIFIED.,.F.,.F.)
B_SPLINE_CURVE_WITH_KNOTS((3,3),(0.339146964126516,0.668418076018306),
 .UNSPECIFIED.)
CURVE()
GEOMETRIC_REPRESENTATION_ITEM()
RATIONAL_B_SPLINE_CURVE((1.00400190544535,1.00495889669789,1.00400190544535))
REPRESENTATION_ITEM('')
);
#19160=(
BOUNDED_CURVE()
B_SPLINE_CURVE(2,(#77576,#77577,#77578),.UNSPECIFIED.,.F.,.F.)
B_SPLINE_CURVE_WITH_KNOTS((3,3),(0.0284639718822116,0.0708739951602902),
 .UNSPECIFIED.)
CURVE()
GEOMETRIC_REPRESENTATION_ITEM()
RATIONAL_B_SPLINE_CURVE((1.00001075159531,1.00001338549162,1.))
REPRESENTATION_ITEM('')
);
#19161=(
BOUNDED_CURVE()
B_SPLINE_CURVE(2,(#77582,#77583,#77584),.UNSPECIFIED.,.F.,.F.)
B_SPLINE_CURVE_WITH_KNOTS((3,3),(0.,0.0424100233379413),.UNSPECIFIED.)
CURVE()
GEOMETRIC_REPRESENTATION_ITEM()
RATIONAL_B_SPLINE_CURVE((1.,1.0000133853148,1.00001075145326))
REPRESENTATION_ITEM('')
);
#19162=(
BOUNDED_CURVE()
B_SPLINE_CURVE(2,(#77586,#77587,#77588),.UNSPECIFIED.,.F.,.F.)
B_SPLINE_CURVE_WITH_KNOTS((3,3),(0.339146964126514,0.668418076018307),
 .UNSPECIFIED.)
CURVE()
GEOMETRIC_REPRESENTATION_ITEM()
RATIONAL_B_SPLINE_CURVE((1.00400190544536,1.0049588966979,1.00400190544536))
REPRESENTATION_ITEM('')
);
#19163=(
BOUNDED_CURVE()
B_SPLINE_CURVE(2,(#77590,#77591,#77592),.UNSPECIFIED.,.F.,.F.)
B_SPLINE_CURVE_WITH_KNOTS((3,3),(0.0284639723011819,0.0708739951602902),
 .UNSPECIFIED.)
CURVE()
GEOMETRIC_REPRESENTATION_ITEM()
RATIONAL_B_SPLINE_CURVE((1.00001075145909,1.00001338532183,1.))
REPRESENTATION_ITEM('')
);
#19164=(
BOUNDED_CURVE()
B_SPLINE_CURVE(2,(#77596,#77597,#77598),.UNSPECIFIED.,.F.,.F.)
B_SPLINE_CURVE_WITH_KNOTS((3,3),(0.,0.0424100235660184),.UNSPECIFIED.)
CURVE()
GEOMETRIC_REPRESENTATION_ITEM()
RATIONAL_B_SPLINE_CURVE((1.,1.0000133839457,1.00001075035348))
REPRESENTATION_ITEM('')
);
#19165=(
BOUNDED_CURVE()
B_SPLINE_CURVE(2,(#77600,#77601,#77602),.UNSPECIFIED.,.F.,.F.)
B_SPLINE_CURVE_WITH_KNOTS((3,3),(0.339146964126508,0.668418076018301),
 .UNSPECIFIED.)
CURVE()
GEOMETRIC_REPRESENTATION_ITEM()
RATIONAL_B_SPLINE_CURVE((1.00400190544536,1.0049588966979,1.00400190544536))
REPRESENTATION_ITEM('')
);
#19166=(
BOUNDED_CURVE()
B_SPLINE_CURVE(2,(#77604,#77605,#77606),.UNSPECIFIED.,.F.,.F.)
B_SPLINE_CURVE_WITH_KNOTS((3,3),(0.0284639720583302,0.0708739951602905),
 .UNSPECIFIED.)
CURVE()
GEOMETRIC_REPRESENTATION_ITEM()
RATIONAL_B_SPLINE_CURVE((1.00001075112448,1.00001338490536,1.))
REPRESENTATION_ITEM('')
);
#19167=(
BOUNDED_CURVE()
B_SPLINE_CURVE(2,(#77610,#77611,#77612),.UNSPECIFIED.,.F.,.F.)
B_SPLINE_CURVE_WITH_KNOTS((3,3),(0.,0.0424100228529261),.UNSPECIFIED.)
CURVE()
GEOMETRIC_REPRESENTATION_ITEM()
RATIONAL_B_SPLINE_CURVE((1.,1.00001338602191,1.00001075202142))
REPRESENTATION_ITEM('')
);
#19168=(
BOUNDED_CURVE()
B_SPLINE_CURVE(2,(#77614,#77615,#77616),.UNSPECIFIED.,.F.,.F.)
B_SPLINE_CURVE_WITH_KNOTS((3,3),(0.339146964126517,0.668418076018306),
 .UNSPECIFIED.)
CURVE()
GEOMETRIC_REPRESENTATION_ITEM()
RATIONAL_B_SPLINE_CURVE((1.00400190544534,1.00495889669788,1.00400190544534))
REPRESENTATION_ITEM('')
);
#19169=(
BOUNDED_CURVE()
B_SPLINE_CURVE(2,(#77618,#77619,#77620),.UNSPECIFIED.,.F.,.F.)
B_SPLINE_CURVE_WITH_KNOTS((3,3),(0.028463971052142,0.0708739951602904),
 .UNSPECIFIED.)
CURVE()
GEOMETRIC_REPRESENTATION_ITEM()
RATIONAL_B_SPLINE_CURVE((1.00001075114436,1.00001338493058,1.))
REPRESENTATION_ITEM('')
);
#19170=(
BOUNDED_CURVE()
B_SPLINE_CURVE(2,(#77646,#77647,#77648),.UNSPECIFIED.,.F.,.F.)
B_SPLINE_CURVE_WITH_KNOTS((3,3),(0.,0.0424100231388671),.UNSPECIFIED.)
CURVE()
GEOMETRIC_REPRESENTATION_ITEM()
RATIONAL_B_SPLINE_CURVE((1.,1.00001338664572,1.00001075252237))
REPRESENTATION_ITEM('')
);
#19171=(
BOUNDED_CURVE()
B_SPLINE_CURVE(2,(#77650,#77651,#77652),.UNSPECIFIED.,.F.,.F.)
B_SPLINE_CURVE_WITH_KNOTS((3,3),(0.339146964126515,0.668418076018309),
 .UNSPECIFIED.)
CURVE()
GEOMETRIC_REPRESENTATION_ITEM()
RATIONAL_B_SPLINE_CURVE((1.00400190544536,1.0049588966979,1.00400190544536))
REPRESENTATION_ITEM('')
);
#19172=(
BOUNDED_CURVE()
B_SPLINE_CURVE(2,(#77654,#77655,#77656),.UNSPECIFIED.,.F.,.F.)
B_SPLINE_CURVE_WITH_KNOTS((3,3),(0.0284639723015322,0.0708739951602894),
 .UNSPECIFIED.)
CURVE()
GEOMETRIC_REPRESENTATION_ITEM()
RATIONAL_B_SPLINE_CURVE((1.00001075245622,1.00001338656323,1.))
REPRESENTATION_ITEM('')
);
#19173=(
BOUNDED_CURVE()
B_SPLINE_CURVE(2,(#77660,#77661,#77662),.UNSPECIFIED.,.F.,.F.)
B_SPLINE_CURVE_WITH_KNOTS((3,3),(0.,0.0424100231020988),.UNSPECIFIED.)
CURVE()
GEOMETRIC_REPRESENTATION_ITEM()
RATIONAL_B_SPLINE_CURVE((1.,1.00001338440371,1.00001075072154))
REPRESENTATION_ITEM('')
);
#19174=(
BOUNDED_CURVE()
B_SPLINE_CURVE(2,(#77664,#77665,#77666),.UNSPECIFIED.,.F.,.F.)
B_SPLINE_CURVE_WITH_KNOTS((3,3),(0.339146964126511,0.668418076018296),
 .UNSPECIFIED.)
CURVE()
GEOMETRIC_REPRESENTATION_ITEM()
RATIONAL_B_SPLINE_CURVE((1.00400190544533,1.00495889669787,1.00400190544533))
REPRESENTATION_ITEM('')
);
#19175=(
BOUNDED_CURVE()
B_SPLINE_CURVE(2,(#77668,#77669,#77670),.UNSPECIFIED.,.F.,.F.)
B_SPLINE_CURVE_WITH_KNOTS((3,3),(0.0284639708332421,0.0708739951602892),
 .UNSPECIFIED.)
CURVE()
GEOMETRIC_REPRESENTATION_ITEM()
RATIONAL_B_SPLINE_CURVE((1.00001075092413,1.00001338465651,1.))
REPRESENTATION_ITEM('')
);
#19176=(
BOUNDED_CURVE()
B_SPLINE_CURVE(2,(#77674,#77675,#77676),.UNSPECIFIED.,.F.,.F.)
B_SPLINE_CURVE_WITH_KNOTS((3,3),(0.,0.0424100226742728),.UNSPECIFIED.)
CURVE()
GEOMETRIC_REPRESENTATION_ITEM()
RATIONAL_B_SPLINE_CURVE((1.,1.00001338671076,1.00001075257479))
REPRESENTATION_ITEM('')
);
#19177=(
BOUNDED_CURVE()
B_SPLINE_CURVE(2,(#77678,#77679,#77680),.UNSPECIFIED.,.F.,.F.)
B_SPLINE_CURVE_WITH_KNOTS((3,3),(0.339146964126517,0.668418076018305),
 .UNSPECIFIED.)
CURVE()
GEOMETRIC_REPRESENTATION_ITEM()
RATIONAL_B_SPLINE_CURVE((1.00400190544534,1.00495889669788,1.00400190544534))
REPRESENTATION_ITEM('')
);
#19178=(
BOUNDED_CURVE()
B_SPLINE_CURVE(2,(#77682,#77683,#77684),.UNSPECIFIED.,.F.,.F.)
B_SPLINE_CURVE_WITH_KNOTS((3,3),(0.0284639727500967,0.0708739951602894),
 .UNSPECIFIED.)
CURVE()
GEOMETRIC_REPRESENTATION_ITEM()
RATIONAL_B_SPLINE_CURVE((1.00001075141119,1.00001338526198,1.))
REPRESENTATION_ITEM('')
);
#19179=(
BOUNDED_CURVE()
B_SPLINE_CURVE(2,(#77688,#77689,#77690),.UNSPECIFIED.,.F.,.F.)
B_SPLINE_CURVE_WITH_KNOTS((3,3),(0.,0.0424100234036622),.UNSPECIFIED.)
CURVE()
GEOMETRIC_REPRESENTATION_ITEM()
RATIONAL_B_SPLINE_CURVE((1.,1.00001338508687,1.00001075127016))
REPRESENTATION_ITEM('')
);
#19180=(
BOUNDED_CURVE()
B_SPLINE_CURVE(2,(#77692,#77693,#77694),.UNSPECIFIED.,.F.,.F.)
B_SPLINE_CURVE_WITH_KNOTS((3,3),(0.339146964126515,0.668418076018302),
 .UNSPECIFIED.)
CURVE()
GEOMETRIC_REPRESENTATION_ITEM()
RATIONAL_B_SPLINE_CURVE((1.00400190544534,1.00495889669787,1.00400190544534))
REPRESENTATION_ITEM('')
);
#19181=(
BOUNDED_CURVE()
B_SPLINE_CURVE(2,(#77696,#77697,#77698),.UNSPECIFIED.,.F.,.F.)
B_SPLINE_CURVE_WITH_KNOTS((3,3),(0.0284639712775601,0.0708739951602893),
 .UNSPECIFIED.)
CURVE()
GEOMETRIC_REPRESENTATION_ITEM()
RATIONAL_B_SPLINE_CURVE((1.00001075126605,1.00001338508198,1.))
REPRESENTATION_ITEM('')
);
#19182=(
BOUNDED_CURVE()
B_SPLINE_CURVE(2,(#77702,#77703,#77704),.UNSPECIFIED.,.F.,.F.)
B_SPLINE_CURVE_WITH_KNOTS((3,3),(0.,0.0424100240945264),.UNSPECIFIED.)
CURVE()
GEOMETRIC_REPRESENTATION_ITEM()
RATIONAL_B_SPLINE_CURVE((1.,1.00001338487308,1.00001075109818))
REPRESENTATION_ITEM('')
);
#19183=(
BOUNDED_CURVE()
B_SPLINE_CURVE(2,(#77706,#77707,#77708),.UNSPECIFIED.,.F.,.F.)
B_SPLINE_CURVE_WITH_KNOTS((3,3),(0.339146964126523,0.668418076018308),
 .UNSPECIFIED.)
CURVE()
GEOMETRIC_REPRESENTATION_ITEM()
RATIONAL_B_SPLINE_CURVE((1.00400190544534,1.00495889669787,1.00400190544534))
REPRESENTATION_ITEM('')
);
#19184=(
BOUNDED_CURVE()
B_SPLINE_CURVE(2,(#77710,#77711,#77712),.UNSPECIFIED.,.F.,.F.)
B_SPLINE_CURVE_WITH_KNOTS((3,3),(0.0284639720159432,0.0708739951602889),
 .UNSPECIFIED.)
CURVE()
GEOMETRIC_REPRESENTATION_ITEM()
RATIONAL_B_SPLINE_CURVE((1.00001075167528,1.00001338559111,1.))
REPRESENTATION_ITEM('')
);
#19185=(
BOUNDED_CURVE()
B_SPLINE_CURVE(2,(#77716,#77717,#77718),.UNSPECIFIED.,.F.,.F.)
B_SPLINE_CURVE_WITH_KNOTS((3,3),(0.,0.0424100244249126),.UNSPECIFIED.)
CURVE()
GEOMETRIC_REPRESENTATION_ITEM()
RATIONAL_B_SPLINE_CURVE((1.,1.0000133850762,1.0000107512612))
REPRESENTATION_ITEM('')
);
#19186=(
BOUNDED_CURVE()
B_SPLINE_CURVE(2,(#77720,#77721,#77722),.UNSPECIFIED.,.F.,.F.)
B_SPLINE_CURVE_WITH_KNOTS((3,3),(0.339146964126521,0.668418076018309),
 .UNSPECIFIED.)
CURVE()
GEOMETRIC_REPRESENTATION_ITEM()
RATIONAL_B_SPLINE_CURVE((1.00400190544534,1.00495889669788,1.00400190544534))
REPRESENTATION_ITEM('')
);
#19187=(
BOUNDED_CURVE()
B_SPLINE_CURVE(2,(#77724,#77725,#77726),.UNSPECIFIED.,.F.,.F.)
B_SPLINE_CURVE_WITH_KNOTS((3,3),(0.0284639713982658,0.0708739951602894),
 .UNSPECIFIED.)
CURVE()
GEOMETRIC_REPRESENTATION_ITEM()
RATIONAL_B_SPLINE_CURVE((1.0000107515649,1.00001338545398,1.))
REPRESENTATION_ITEM('')
);
#19188=(
BOUNDED_CURVE()
B_SPLINE_CURVE(2,(#77730,#77731,#77732),.UNSPECIFIED.,.F.,.F.)
B_SPLINE_CURVE_WITH_KNOTS((3,3),(0.,0.0424100230579472),.UNSPECIFIED.)
CURVE()
GEOMETRIC_REPRESENTATION_ITEM()
RATIONAL_B_SPLINE_CURVE((1.,1.00001338543977,1.00001075155375))
REPRESENTATION_ITEM('')
);
#19189=(
BOUNDED_CURVE()
B_SPLINE_CURVE(2,(#77734,#77735,#77736),.UNSPECIFIED.,.F.,.F.)
B_SPLINE_CURVE_WITH_KNOTS((3,3),(0.339146964126514,0.668418076018301),
 .UNSPECIFIED.)
CURVE()
GEOMETRIC_REPRESENTATION_ITEM()
RATIONAL_B_SPLINE_CURVE((1.00400190544534,1.00495889669788,1.00400190544534))
REPRESENTATION_ITEM('')
);
#19190=(
BOUNDED_CURVE()
B_SPLINE_CURVE(2,(#77738,#77739,#77740),.UNSPECIFIED.,.F.,.F.)
B_SPLINE_CURVE_WITH_KNOTS((3,3),(0.0284639721460146,0.0708739951602892),
 .UNSPECIFIED.)
CURVE()
GEOMETRIC_REPRESENTATION_ITEM()
RATIONAL_B_SPLINE_CURVE((1.00001075127041,1.00001338508699,1.))
REPRESENTATION_ITEM('')
);
#19191=(
BOUNDED_CURVE()
B_SPLINE_CURVE(2,(#77744,#77745,#77746),.UNSPECIFIED.,.F.,.F.)
B_SPLINE_CURVE_WITH_KNOTS((3,3),(0.,0.04241002310436),.UNSPECIFIED.)
CURVE()
GEOMETRIC_REPRESENTATION_ITEM()
RATIONAL_B_SPLINE_CURVE((1.,1.00001338427162,1.00001075061544))
REPRESENTATION_ITEM('')
);
#19192=(
BOUNDED_CURVE()
B_SPLINE_CURVE(2,(#77748,#77749,#77750),.UNSPECIFIED.,.F.,.F.)
B_SPLINE_CURVE_WITH_KNOTS((3,3),(0.339146964126508,0.668418076018301),
 .UNSPECIFIED.)
CURVE()
GEOMETRIC_REPRESENTATION_ITEM()
RATIONAL_B_SPLINE_CURVE((1.00400190544536,1.0049588966979,1.00400190544536))
REPRESENTATION_ITEM('')
);
#19193=(
BOUNDED_CURVE()
B_SPLINE_CURVE(2,(#77752,#77753,#77754),.UNSPECIFIED.,.F.,.F.)
B_SPLINE_CURVE_WITH_KNOTS((3,3),(0.0284639718065398,0.0708739951602892),
 .UNSPECIFIED.)
CURVE()
GEOMETRIC_REPRESENTATION_ITEM()
RATIONAL_B_SPLINE_CURVE((1.00001075054903,1.00001338418905,1.))
REPRESENTATION_ITEM('')
);
#19194=(
BOUNDED_CURVE()
B_SPLINE_CURVE(2,(#77758,#77759,#77760),.UNSPECIFIED.,.F.,.F.)
B_SPLINE_CURVE_WITH_KNOTS((3,3),(0.,0.0424100238902531),.UNSPECIFIED.)
CURVE()
GEOMETRIC_REPRESENTATION_ITEM()
RATIONAL_B_SPLINE_CURVE((1.,1.00001338471342,1.00001075097001))
REPRESENTATION_ITEM('')
);
#19195=(
BOUNDED_CURVE()
B_SPLINE_CURVE(2,(#77762,#77763,#77764),.UNSPECIFIED.,.F.,.F.)
B_SPLINE_CURVE_WITH_KNOTS((3,3),(0.339146964126505,0.668418076018296),
 .UNSPECIFIED.)
CURVE()
GEOMETRIC_REPRESENTATION_ITEM()
RATIONAL_B_SPLINE_CURVE((1.00400190544535,1.00495889669789,1.00400190544535))
REPRESENTATION_ITEM('')
);
#19196=(
BOUNDED_CURVE()
B_SPLINE_CURVE(2,(#77766,#77767,#77768),.UNSPECIFIED.,.F.,.F.)
B_SPLINE_CURVE_WITH_KNOTS((3,3),(0.0284639726785229,0.0708739951602891),
 .UNSPECIFIED.)
CURVE()
GEOMETRIC_REPRESENTATION_ITEM()
RATIONAL_B_SPLINE_CURVE((1.00001075174529,1.00001338567796,1.))
REPRESENTATION_ITEM('')
);
#19197=(
BOUNDED_CURVE()
B_SPLINE_CURVE(2,(#77772,#77773,#77774),.UNSPECIFIED.,.F.,.F.)
B_SPLINE_CURVE_WITH_KNOTS((3,3),(0.,0.0424100231217665),.UNSPECIFIED.)
CURVE()
GEOMETRIC_REPRESENTATION_ITEM()
RATIONAL_B_SPLINE_CURVE((1.,1.00001338590548,1.00001075192779))
REPRESENTATION_ITEM('')
);
#19198=(
BOUNDED_CURVE()
B_SPLINE_CURVE(2,(#77776,#77777,#77778),.UNSPECIFIED.,.F.,.F.)
B_SPLINE_CURVE_WITH_KNOTS((3,3),(0.339146964126517,0.668418076018306),
 .UNSPECIFIED.)
CURVE()
GEOMETRIC_REPRESENTATION_ITEM()
RATIONAL_B_SPLINE_CURVE((1.00400190544534,1.00495889669788,1.00400190544534))
REPRESENTATION_ITEM('')
);
#19199=(
BOUNDED_CURVE()
B_SPLINE_CURVE(2,(#77780,#77781,#77782),.UNSPECIFIED.,.F.,.F.)
B_SPLINE_CURVE_WITH_KNOTS((3,3),(0.0284639722994484,0.0708739951602894),
 .UNSPECIFIED.)
CURVE()
GEOMETRIC_REPRESENTATION_ITEM()
RATIONAL_B_SPLINE_CURVE((1.00001075268953,1.0000133868537,1.))
REPRESENTATION_ITEM('')
);
#19200=(
BOUNDED_CURVE()
B_SPLINE_CURVE(2,(#77786,#77787,#77788),.UNSPECIFIED.,.F.,.F.)
B_SPLINE_CURVE_WITH_KNOTS((3,3),(0.,0.0424100235663187),.UNSPECIFIED.)
CURVE()
GEOMETRIC_REPRESENTATION_ITEM()
RATIONAL_B_SPLINE_CURVE((1.,1.00001338431496,1.00001075065008))
REPRESENTATION_ITEM('')
);
#19201=(
BOUNDED_CURVE()
B_SPLINE_CURVE(2,(#77790,#77791,#77792),.UNSPECIFIED.,.F.,.F.)
B_SPLINE_CURVE_WITH_KNOTS((3,3),(0.339146964126511,0.668418076018303),
 .UNSPECIFIED.)
CURVE()
GEOMETRIC_REPRESENTATION_ITEM()
RATIONAL_B_SPLINE_CURVE((1.00400190544536,1.0049588966979,1.00400190544536))
REPRESENTATION_ITEM('')
);
#19202=(
BOUNDED_CURVE()
B_SPLINE_CURVE(2,(#77794,#77795,#77796),.UNSPECIFIED.,.F.,.F.)
B_SPLINE_CURVE_WITH_KNOTS((3,3),(0.0284639715440609,0.0708739951602894),
 .UNSPECIFIED.)
CURVE()
GEOMETRIC_REPRESENTATION_ITEM()
RATIONAL_B_SPLINE_CURVE((1.00001075063711,1.00001338429884,1.))
REPRESENTATION_ITEM('')
);
#19203=(
BOUNDED_CURVE()
B_SPLINE_CURVE(2,(#77799,#77800,#77801),.UNSPECIFIED.,.F.,.F.)
B_SPLINE_CURVE_WITH_KNOTS((3,3),(0.,0.0709397118056797),.UNSPECIFIED.)
CURVE()
GEOMETRIC_REPRESENTATION_ITEM()
RATIONAL_B_SPLINE_CURVE((1.,1.00002245139626,1.))
REPRESENTATION_ITEM('')
);
#19204=(
BOUNDED_CURVE()
B_SPLINE_CURVE(2,(#77804,#77805,#77806),.UNSPECIFIED.,.F.,.F.)
B_SPLINE_CURVE_WITH_KNOTS((3,3),(0.,0.0709397118056796),.UNSPECIFIED.)
CURVE()
GEOMETRIC_REPRESENTATION_ITEM()
RATIONAL_B_SPLINE_CURVE((1.,1.00002245118033,1.))
REPRESENTATION_ITEM('')
);
#19205=(
BOUNDED_CURVE()
B_SPLINE_CURVE(2,(#77810,#77811,#77812),.UNSPECIFIED.,.F.,.F.)
B_SPLINE_CURVE_WITH_KNOTS((3,3),(0.,0.0424100230703566),.UNSPECIFIED.)
CURVE()
GEOMETRIC_REPRESENTATION_ITEM()
RATIONAL_B_SPLINE_CURVE((1.,1.00001338676863,1.00001075262112))
REPRESENTATION_ITEM('')
);
#19206=(
BOUNDED_CURVE()
B_SPLINE_CURVE(2,(#77814,#77815,#77816),.UNSPECIFIED.,.F.,.F.)
B_SPLINE_CURVE_WITH_KNOTS((3,3),(0.339146964126514,0.668418076018302),
 .UNSPECIFIED.)
CURVE()
GEOMETRIC_REPRESENTATION_ITEM()
RATIONAL_B_SPLINE_CURVE((1.00400190544535,1.00495889669788,1.00400190544535))
REPRESENTATION_ITEM('')
);
#19207=(
BOUNDED_CURVE()
B_SPLINE_CURVE(2,(#77818,#77819,#77820),.UNSPECIFIED.,.F.,.F.)
B_SPLINE_CURVE_WITH_KNOTS((3,3),(0.0284639721307315,0.0708739951602897),
 .UNSPECIFIED.)
CURVE()
GEOMETRIC_REPRESENTATION_ITEM()
RATIONAL_B_SPLINE_CURVE((1.00001075251047,1.00001338663085,1.))
REPRESENTATION_ITEM('')
);
#19208=(
BOUNDED_CURVE()
B_SPLINE_CURVE(2,(#77824,#77825,#77826),.UNSPECIFIED.,.F.,.F.)
B_SPLINE_CURVE_WITH_KNOTS((3,3),(0.,0.0424100231451836),.UNSPECIFIED.)
CURVE()
GEOMETRIC_REPRESENTATION_ITEM()
RATIONAL_B_SPLINE_CURVE((1.,1.0000133845857,1.0000107508677))
REPRESENTATION_ITEM('')
);
#19209=(
BOUNDED_CURVE()
B_SPLINE_CURVE(2,(#77828,#77829,#77830),.UNSPECIFIED.,.F.,.F.)
B_SPLINE_CURVE_WITH_KNOTS((3,3),(0.33914696412651,0.668418076018305),
 .UNSPECIFIED.)
CURVE()
GEOMETRIC_REPRESENTATION_ITEM()
RATIONAL_B_SPLINE_CURVE((1.00400190544536,1.0049588966979,1.00400190544536))
REPRESENTATION_ITEM('')
);
#19210=(
BOUNDED_CURVE()
B_SPLINE_CURVE(2,(#77832,#77833,#77834),.UNSPECIFIED.,.F.,.F.)
B_SPLINE_CURVE_WITH_KNOTS((3,3),(0.0284639724981747,0.0708739951602894),
 .UNSPECIFIED.)
CURVE()
GEOMETRIC_REPRESENTATION_ITEM()
RATIONAL_B_SPLINE_CURVE((1.00001075165203,1.00001338556194,1.))
REPRESENTATION_ITEM('')
);
#19211=(
BOUNDED_CURVE()
B_SPLINE_CURVE(2,(#77838,#77839,#77840),.UNSPECIFIED.,.F.,.F.)
B_SPLINE_CURVE_WITH_KNOTS((3,3),(0.,0.0424100229360319),.UNSPECIFIED.)
CURVE()
GEOMETRIC_REPRESENTATION_ITEM()
RATIONAL_B_SPLINE_CURVE((1.,1.00001338532576,1.00001075146222))
REPRESENTATION_ITEM('')
);
#19212=(
BOUNDED_CURVE()
B_SPLINE_CURVE(2,(#77842,#77843,#77844),.UNSPECIFIED.,.F.,.F.)
B_SPLINE_CURVE_WITH_KNOTS((3,3),(0.339146964126522,0.668418076018311),
 .UNSPECIFIED.)
CURVE()
GEOMETRIC_REPRESENTATION_ITEM()
RATIONAL_B_SPLINE_CURVE((1.00400190544535,1.00495889669788,1.00400190544535))
REPRESENTATION_ITEM('')
);
#19213=(
BOUNDED_CURVE()
B_SPLINE_CURVE(2,(#77846,#77847,#77848),.UNSPECIFIED.,.F.,.F.)
B_SPLINE_CURVE_WITH_KNOTS((3,3),(0.0284639726217467,0.0708739951602899),
 .UNSPECIFIED.)
CURVE()
GEOMETRIC_REPRESENTATION_ITEM()
RATIONAL_B_SPLINE_CURVE((1.00001075156159,1.00001338544929,1.))
REPRESENTATION_ITEM('')
);
#19214=(
BOUNDED_CURVE()
B_SPLINE_CURVE(2,(#77852,#77853,#77854),.UNSPECIFIED.,.F.,.F.)
B_SPLINE_CURVE_WITH_KNOTS((3,3),(0.,0.0424100234950521),.UNSPECIFIED.)
CURVE()
GEOMETRIC_REPRESENTATION_ITEM()
RATIONAL_B_SPLINE_CURVE((1.,1.00001338503236,1.00001075122634))
REPRESENTATION_ITEM('')
);
#19215=(
BOUNDED_CURVE()
B_SPLINE_CURVE(2,(#77856,#77857,#77858),.UNSPECIFIED.,.F.,.F.)
B_SPLINE_CURVE_WITH_KNOTS((3,3),(0.339146964126523,0.668418076018307),
 .UNSPECIFIED.)
CURVE()
GEOMETRIC_REPRESENTATION_ITEM()
RATIONAL_B_SPLINE_CURVE((1.00400190544533,1.00495889669786,1.00400190544533))
REPRESENTATION_ITEM('')
);
#19216=(
BOUNDED_CURVE()
B_SPLINE_CURVE(2,(#77860,#77861,#77862),.UNSPECIFIED.,.F.,.F.)
B_SPLINE_CURVE_WITH_KNOTS((3,3),(0.0284639715189242,0.0708739951602895),
 .UNSPECIFIED.)
CURVE()
GEOMETRIC_REPRESENTATION_ITEM()
RATIONAL_B_SPLINE_CURVE((1.00001075178646,1.00001338572976,1.))
REPRESENTATION_ITEM('')
);
#19217=(
BOUNDED_CURVE()
B_SPLINE_CURVE(2,(#77866,#77867,#77868),.UNSPECIFIED.,.F.,.F.)
B_SPLINE_CURVE_WITH_KNOTS((3,3),(0.,0.0424100236202695),.UNSPECIFIED.)
CURVE()
GEOMETRIC_REPRESENTATION_ITEM()
RATIONAL_B_SPLINE_CURVE((1.,1.00001338464189,1.00001075091266))
REPRESENTATION_ITEM('')
);
#19218=(
BOUNDED_CURVE()
B_SPLINE_CURVE(2,(#77870,#77871,#77872),.UNSPECIFIED.,.F.,.F.)
B_SPLINE_CURVE_WITH_KNOTS((3,3),(0.339146964126517,0.668418076018307),
 .UNSPECIFIED.)
CURVE()
GEOMETRIC_REPRESENTATION_ITEM()
RATIONAL_B_SPLINE_CURVE((1.00400190544535,1.00495889669789,1.00400190544535))
REPRESENTATION_ITEM('')
);
#19219=(
BOUNDED_CURVE()
B_SPLINE_CURVE(2,(#77874,#77875,#77876),.UNSPECIFIED.,.F.,.F.)
B_SPLINE_CURVE_WITH_KNOTS((3,3),(0.0284639715457675,0.0708739951602893),
 .UNSPECIFIED.)
CURVE()
GEOMETRIC_REPRESENTATION_ITEM()
RATIONAL_B_SPLINE_CURVE((1.00001075081926,1.00001338452561,1.))
REPRESENTATION_ITEM('')
);
#19220=(
BOUNDED_CURVE()
B_SPLINE_CURVE(2,(#77880,#77881,#77882),.UNSPECIFIED.,.F.,.F.)
B_SPLINE_CURVE_WITH_KNOTS((3,3),(0.,0.0424100233833892),.UNSPECIFIED.)
CURVE()
GEOMETRIC_REPRESENTATION_ITEM()
RATIONAL_B_SPLINE_CURVE((1.,1.00001338550802,1.00001075160844))
REPRESENTATION_ITEM('')
);
#19221=(
BOUNDED_CURVE()
B_SPLINE_CURVE(2,(#77884,#77885,#77886),.UNSPECIFIED.,.F.,.F.)
B_SPLINE_CURVE_WITH_KNOTS((3,3),(0.339146964126518,0.668418076018304),
 .UNSPECIFIED.)
CURVE()
GEOMETRIC_REPRESENTATION_ITEM()
RATIONAL_B_SPLINE_CURVE((1.00400190544534,1.00495889669787,1.00400190544534))
REPRESENTATION_ITEM('')
);
#19222=(
BOUNDED_CURVE()
B_SPLINE_CURVE(2,(#77888,#77889,#77890),.UNSPECIFIED.,.F.,.F.)
B_SPLINE_CURVE_WITH_KNOTS((3,3),(0.0284639718266628,0.0708739951602895),
 .UNSPECIFIED.)
CURVE()
GEOMETRIC_REPRESENTATION_ITEM()
RATIONAL_B_SPLINE_CURVE((1.00001075166489,1.00001338557827,1.))
REPRESENTATION_ITEM('')
);
#19223=(
BOUNDED_CURVE()
B_SPLINE_CURVE(2,(#77894,#77895,#77896),.UNSPECIFIED.,.F.,.F.)
B_SPLINE_CURVE_WITH_KNOTS((3,3),(0.,0.0424100233211347),.UNSPECIFIED.)
CURVE()
GEOMETRIC_REPRESENTATION_ITEM()
RATIONAL_B_SPLINE_CURVE((1.,1.00001338542288,1.00001075154008))
REPRESENTATION_ITEM('')
);
#19224=(
BOUNDED_CURVE()
B_SPLINE_CURVE(2,(#77898,#77899,#77900),.UNSPECIFIED.,.F.,.F.)
B_SPLINE_CURVE_WITH_KNOTS((3,3),(0.339146964126512,0.668418076018303),
 .UNSPECIFIED.)
CURVE()
GEOMETRIC_REPRESENTATION_ITEM()
RATIONAL_B_SPLINE_CURVE((1.00400190544535,1.00495889669789,1.00400190544535))
REPRESENTATION_ITEM('')
);
#19225=(
BOUNDED_CURVE()
B_SPLINE_CURVE(2,(#77902,#77903,#77904),.UNSPECIFIED.,.F.,.F.)
B_SPLINE_CURVE_WITH_KNOTS((3,3),(0.028463972158878,0.0708739951602892),
 .UNSPECIFIED.)
CURVE()
GEOMETRIC_REPRESENTATION_ITEM()
RATIONAL_B_SPLINE_CURVE((1.00001075106213,1.00001338482769,1.))
REPRESENTATION_ITEM('')
);
#19226=(
BOUNDED_CURVE()
B_SPLINE_CURVE(2,(#77908,#77909,#77910),.UNSPECIFIED.,.F.,.F.)
B_SPLINE_CURVE_WITH_KNOTS((3,3),(0.,0.0424100233711627),.UNSPECIFIED.)
CURVE()
GEOMETRIC_REPRESENTATION_ITEM()
RATIONAL_B_SPLINE_CURVE((1.,1.00001338461061,1.00001075088763))
REPRESENTATION_ITEM('')
);
#19227=(
BOUNDED_CURVE()
B_SPLINE_CURVE(2,(#77912,#77913,#77914),.UNSPECIFIED.,.F.,.F.)
B_SPLINE_CURVE_WITH_KNOTS((3,3),(0.339146964126523,0.668418076018308),
 .UNSPECIFIED.)
CURVE()
GEOMETRIC_REPRESENTATION_ITEM()
RATIONAL_B_SPLINE_CURVE((1.00400190544534,1.00495889669787,1.00400190544534))
REPRESENTATION_ITEM('')
);
#19228=(
BOUNDED_CURVE()
B_SPLINE_CURVE(2,(#77916,#77917,#77918),.UNSPECIFIED.,.F.,.F.)
B_SPLINE_CURVE_WITH_KNOTS((3,3),(0.0284639720394568,0.0708739951602894),
 .UNSPECIFIED.)
CURVE()
GEOMETRIC_REPRESENTATION_ITEM()
RATIONAL_B_SPLINE_CURVE((1.00001075151129,1.00001338538694,1.))
REPRESENTATION_ITEM('')
);
#19229=(
BOUNDED_CURVE()
B_SPLINE_CURVE(2,(#77922,#77923,#77924),.UNSPECIFIED.,.F.,.F.)
B_SPLINE_CURVE_WITH_KNOTS((3,3),(0.,0.042410023028666),.UNSPECIFIED.)
CURVE()
GEOMETRIC_REPRESENTATION_ITEM()
RATIONAL_B_SPLINE_CURVE((1.,1.00001338527187,1.0000107514189))
REPRESENTATION_ITEM('')
);
#19230=(
BOUNDED_CURVE()
B_SPLINE_CURVE(2,(#77926,#77927,#77928),.UNSPECIFIED.,.F.,.F.)
B_SPLINE_CURVE_WITH_KNOTS((3,3),(0.339146964126521,0.668418076018309),
 .UNSPECIFIED.)
CURVE()
GEOMETRIC_REPRESENTATION_ITEM()
RATIONAL_B_SPLINE_CURVE((1.00400190544534,1.00495889669788,1.00400190544534))
REPRESENTATION_ITEM('')
);
#19231=(
BOUNDED_CURVE()
B_SPLINE_CURVE(2,(#77930,#77931,#77932),.UNSPECIFIED.,.F.,.F.)
B_SPLINE_CURVE_WITH_KNOTS((3,3),(0.0284639713944435,0.0708739951602898),
 .UNSPECIFIED.)
CURVE()
GEOMETRIC_REPRESENTATION_ITEM()
RATIONAL_B_SPLINE_CURVE((1.00001075185111,1.00001338581031,1.))
REPRESENTATION_ITEM('')
);
#19232=(
BOUNDED_CURVE()
B_SPLINE_CURVE(2,(#77936,#77937,#77938),.UNSPECIFIED.,.F.,.F.)
B_SPLINE_CURVE_WITH_KNOTS((3,3),(0.,0.0424100230585016),.UNSPECIFIED.)
CURVE()
GEOMETRIC_REPRESENTATION_ITEM()
RATIONAL_B_SPLINE_CURVE((1.,1.00001338563914,1.00001075171389))
REPRESENTATION_ITEM('')
);
#19233=(
BOUNDED_CURVE()
B_SPLINE_CURVE(2,(#77940,#77941,#77942),.UNSPECIFIED.,.F.,.F.)
B_SPLINE_CURVE_WITH_KNOTS((3,3),(0.339146964126512,0.668418076018301),
 .UNSPECIFIED.)
CURVE()
GEOMETRIC_REPRESENTATION_ITEM()
RATIONAL_B_SPLINE_CURVE((1.00400190544535,1.00495889669789,1.00400190544535))
REPRESENTATION_ITEM('')
);
#19234=(
BOUNDED_CURVE()
B_SPLINE_CURVE(2,(#77944,#77945,#77946),.UNSPECIFIED.,.F.,.F.)
B_SPLINE_CURVE_WITH_KNOTS((3,3),(0.0284639714315111,0.0708739951602896),
 .UNSPECIFIED.)
CURVE()
GEOMETRIC_REPRESENTATION_ITEM()
RATIONAL_B_SPLINE_CURVE((1.00001075192806,1.00001338590609,1.))
REPRESENTATION_ITEM('')
);
#19235=(
BOUNDED_CURVE()
B_SPLINE_CURVE(2,(#77950,#77951,#77952),.UNSPECIFIED.,.F.,.F.)
B_SPLINE_CURVE_WITH_KNOTS((3,3),(0.,0.0424100231762053),.UNSPECIFIED.)
CURVE()
GEOMETRIC_REPRESENTATION_ITEM()
RATIONAL_B_SPLINE_CURVE((1.,1.00001338544772,1.00001075156009))
REPRESENTATION_ITEM('')
);
#19236=(
BOUNDED_CURVE()
B_SPLINE_CURVE(2,(#77954,#77955,#77956),.UNSPECIFIED.,.F.,.F.)
B_SPLINE_CURVE_WITH_KNOTS((3,3),(0.339146964126514,0.668418076018301),
 .UNSPECIFIED.)
CURVE()
GEOMETRIC_REPRESENTATION_ITEM()
RATIONAL_B_SPLINE_CURVE((1.00400190544534,1.00495889669788,1.00400190544534))
REPRESENTATION_ITEM('')
);
#19237=(
BOUNDED_CURVE()
B_SPLINE_CURVE(2,(#77957,#77958,#77959),.UNSPECIFIED.,.F.,.F.)
B_SPLINE_CURVE_WITH_KNOTS((3,3),(0.0284639718065639,0.070873995160289),
 .UNSPECIFIED.)
CURVE()
GEOMETRIC_REPRESENTATION_ITEM()
RATIONAL_B_SPLINE_CURVE((1.00001075095126,1.00001338468982,1.))
REPRESENTATION_ITEM('')
);
#19238=(
BOUNDED_CURVE()
B_SPLINE_CURVE(2,(#77968,#77969,#77970),.UNSPECIFIED.,.F.,.F.)
B_SPLINE_CURVE_WITH_KNOTS((3,3),(0.,0.0709397118056795),.UNSPECIFIED.)
CURVE()
GEOMETRIC_REPRESENTATION_ITEM()
RATIONAL_B_SPLINE_CURVE((1.,1.00002245218476,1.))
REPRESENTATION_ITEM('')
);
#19239=(
BOUNDED_CURVE()
B_SPLINE_CURVE(2,(#77973,#77974,#77975),.UNSPECIFIED.,.F.,.F.)
B_SPLINE_CURVE_WITH_KNOTS((3,3),(0.,0.0709397118056799),.UNSPECIFIED.)
CURVE()
GEOMETRIC_REPRESENTATION_ITEM()
RATIONAL_B_SPLINE_CURVE((1.,1.00002245184959,1.))
REPRESENTATION_ITEM('')
);
#19240=(
BOUNDED_CURVE()
B_SPLINE_CURVE(2,(#77985,#77986,#77987),.UNSPECIFIED.,.F.,.F.)
B_SPLINE_CURVE_WITH_KNOTS((3,3),(0.,0.0709397118056798),.UNSPECIFIED.)
CURVE()
GEOMETRIC_REPRESENTATION_ITEM()
RATIONAL_B_SPLINE_CURVE((1.,1.00002245136635,1.))
REPRESENTATION_ITEM('')
);
#19241=(
BOUNDED_CURVE()
B_SPLINE_CURVE(2,(#77991,#77992,#77993),.UNSPECIFIED.,.F.,.F.)
B_SPLINE_CURVE_WITH_KNOTS((3,3),(0.,0.0424100231686042),.UNSPECIFIED.)
CURVE()
GEOMETRIC_REPRESENTATION_ITEM()
RATIONAL_B_SPLINE_CURVE((1.,1.00001338527369,1.00001075142031))
REPRESENTATION_ITEM('')
);
#19242=(
BOUNDED_CURVE()
B_SPLINE_CURVE(2,(#77995,#77996,#77997),.UNSPECIFIED.,.F.,.F.)
B_SPLINE_CURVE_WITH_KNOTS((3,3),(0.339146964126513,0.668418076018301),
 .UNSPECIFIED.)
CURVE()
GEOMETRIC_REPRESENTATION_ITEM()
RATIONAL_B_SPLINE_CURVE((1.00400190544534,1.00495889669788,1.00400190544534))
REPRESENTATION_ITEM('')
);
#19243=(
BOUNDED_CURVE()
B_SPLINE_CURVE(2,(#77999,#78000,#78001),.UNSPECIFIED.,.F.,.F.)
B_SPLINE_CURVE_WITH_KNOTS((3,3),(0.0284639717703716,0.0708739951602899),
 .UNSPECIFIED.)
CURVE()
GEOMETRIC_REPRESENTATION_ITEM()
RATIONAL_B_SPLINE_CURVE((1.00001075056076,1.00001338420368,1.))
REPRESENTATION_ITEM('')
);
#19244=(
BOUNDED_CURVE()
B_SPLINE_CURVE(2,(#78005,#78006,#78007),.UNSPECIFIED.,.F.,.F.)
B_SPLINE_CURVE_WITH_KNOTS((3,3),(0.,0.0424100236434718),.UNSPECIFIED.)
CURVE()
GEOMETRIC_REPRESENTATION_ITEM()
RATIONAL_B_SPLINE_CURVE((1.,1.0000133842216,1.00001075057506))
REPRESENTATION_ITEM('')
);
#19245=(
BOUNDED_CURVE()
B_SPLINE_CURVE(2,(#78009,#78010,#78011),.UNSPECIFIED.,.F.,.F.)
B_SPLINE_CURVE_WITH_KNOTS((3,3),(0.339146964126518,0.668418076018304),
 .UNSPECIFIED.)
CURVE()
GEOMETRIC_REPRESENTATION_ITEM()
RATIONAL_B_SPLINE_CURVE((1.00400190544534,1.00495889669787,1.00400190544534))
REPRESENTATION_ITEM('')
);
#19246=(
BOUNDED_CURVE()
B_SPLINE_CURVE(2,(#78013,#78014,#78015),.UNSPECIFIED.,.F.,.F.)
B_SPLINE_CURVE_WITH_KNOTS((3,3),(0.0284639718440856,0.0708739951602902),
 .UNSPECIFIED.)
CURVE()
GEOMETRIC_REPRESENTATION_ITEM()
RATIONAL_B_SPLINE_CURVE((1.00001075101626,1.00001338477073,1.))
REPRESENTATION_ITEM('')
);
#19247=(
BOUNDED_CURVE()
B_SPLINE_CURVE(2,(#78019,#78020,#78021),.UNSPECIFIED.,.F.,.F.)
B_SPLINE_CURVE_WITH_KNOTS((3,3),(0.,0.0424100231103199),.UNSPECIFIED.)
CURVE()
GEOMETRIC_REPRESENTATION_ITEM()
RATIONAL_B_SPLINE_CURVE((1.,1.00001338475467,1.00001075100344))
REPRESENTATION_ITEM('')
);
#19248=(
BOUNDED_CURVE()
B_SPLINE_CURVE(2,(#78023,#78024,#78025),.UNSPECIFIED.,.F.,.F.)
B_SPLINE_CURVE_WITH_KNOTS((3,3),(0.339146964126514,0.668418076018306),
 .UNSPECIFIED.)
CURVE()
GEOMETRIC_REPRESENTATION_ITEM()
RATIONAL_B_SPLINE_CURVE((1.00400190544536,1.0049588966979,1.00400190544536))
REPRESENTATION_ITEM('')
);
#19249=(
BOUNDED_CURVE()
B_SPLINE_CURVE(2,(#78027,#78028,#78029),.UNSPECIFIED.,.F.,.F.)
B_SPLINE_CURVE_WITH_KNOTS((3,3),(0.0284639723140838,0.0708739951602902),
 .UNSPECIFIED.)
CURVE()
GEOMETRIC_REPRESENTATION_ITEM()
RATIONAL_B_SPLINE_CURVE((1.00001075055174,1.00001338419219,1.))
REPRESENTATION_ITEM('')
);
#19250=(
BOUNDED_CURVE()
B_SPLINE_CURVE(2,(#78033,#78034,#78035),.UNSPECIFIED.,.F.,.F.)
B_SPLINE_CURVE_WITH_KNOTS((3,3),(0.,0.0424100235660184),.UNSPECIFIED.)
CURVE()
GEOMETRIC_REPRESENTATION_ITEM()
RATIONAL_B_SPLINE_CURVE((1.,1.0000133839457,1.00001075035348))
REPRESENTATION_ITEM('')
);
#19251=(
BOUNDED_CURVE()
B_SPLINE_CURVE(2,(#78037,#78038,#78039),.UNSPECIFIED.,.F.,.F.)
B_SPLINE_CURVE_WITH_KNOTS((3,3),(0.339146964126508,0.668418076018301),
 .UNSPECIFIED.)
CURVE()
GEOMETRIC_REPRESENTATION_ITEM()
RATIONAL_B_SPLINE_CURVE((1.00400190544536,1.0049588966979,1.00400190544536))
REPRESENTATION_ITEM('')
);
#19252=(
BOUNDED_CURVE()
B_SPLINE_CURVE(2,(#78041,#78042,#78043),.UNSPECIFIED.,.F.,.F.)
B_SPLINE_CURVE_WITH_KNOTS((3,3),(0.0284639720583302,0.0708739951602905),
 .UNSPECIFIED.)
CURVE()
GEOMETRIC_REPRESENTATION_ITEM()
RATIONAL_B_SPLINE_CURVE((1.00001075112448,1.00001338490536,1.))
REPRESENTATION_ITEM('')
);
#19253=(
BOUNDED_CURVE()
B_SPLINE_CURVE(2,(#78047,#78048,#78049),.UNSPECIFIED.,.F.,.F.)
B_SPLINE_CURVE_WITH_KNOTS((3,3),(0.,0.0424100220617497),.UNSPECIFIED.)
CURVE()
GEOMETRIC_REPRESENTATION_ITEM()
RATIONAL_B_SPLINE_CURVE((1.,1.00001338539763,1.00001075152027))
REPRESENTATION_ITEM('')
);
#19254=(
BOUNDED_CURVE()
B_SPLINE_CURVE(2,(#78051,#78052,#78053),.UNSPECIFIED.,.F.,.F.)
B_SPLINE_CURVE_WITH_KNOTS((3,3),(0.339146964126514,0.668418076018307),
 .UNSPECIFIED.)
CURVE()
GEOMETRIC_REPRESENTATION_ITEM()
RATIONAL_B_SPLINE_CURVE((1.00400190544536,1.0049588966979,1.00400190544536))
REPRESENTATION_ITEM('')
);
#19255=(
BOUNDED_CURVE()
B_SPLINE_CURVE(2,(#78055,#78056,#78057),.UNSPECIFIED.,.F.,.F.)
B_SPLINE_CURVE_WITH_KNOTS((3,3),(0.0284639715520864,0.07087399516029),
 .UNSPECIFIED.)
CURVE()
GEOMETRIC_REPRESENTATION_ITEM()
RATIONAL_B_SPLINE_CURVE((1.00001075068925,1.00001338436375,1.))
REPRESENTATION_ITEM('')
);
#19256=(
BOUNDED_CURVE()
B_SPLINE_CURVE(2,(#78061,#78062,#78063),.UNSPECIFIED.,.F.,.F.)
B_SPLINE_CURVE_WITH_KNOTS((3,3),(0.,0.04241002248244),.UNSPECIFIED.)
CURVE()
GEOMETRIC_REPRESENTATION_ITEM()
RATIONAL_B_SPLINE_CURVE((1.,1.00001338499034,1.00001075119297))
REPRESENTATION_ITEM('')
);
#19257=(
BOUNDED_CURVE()
B_SPLINE_CURVE(2,(#78065,#78066,#78067),.UNSPECIFIED.,.F.,.F.)
B_SPLINE_CURVE_WITH_KNOTS((3,3),(0.339146964126512,0.668418076018301),
 .UNSPECIFIED.)
CURVE()
GEOMETRIC_REPRESENTATION_ITEM()
RATIONAL_B_SPLINE_CURVE((1.00400190544534,1.00495889669788,1.00400190544534))
REPRESENTATION_ITEM('')
);
#19258=(
BOUNDED_CURVE()
B_SPLINE_CURVE(2,(#78069,#78070,#78071),.UNSPECIFIED.,.F.,.F.)
B_SPLINE_CURVE_WITH_KNOTS((3,3),(0.0284639721565262,0.0708739951602904),
 .UNSPECIFIED.)
CURVE()
GEOMETRIC_REPRESENTATION_ITEM()
RATIONAL_B_SPLINE_CURVE((1.0000107506802,1.00001338435219,1.))
REPRESENTATION_ITEM('')
);
#19259=(
BOUNDED_CURVE()
B_SPLINE_CURVE(2,(#78075,#78076,#78077),.UNSPECIFIED.,.F.,.F.)
B_SPLINE_CURVE_WITH_KNOTS((3,3),(0.,0.0424100240923756),.UNSPECIFIED.)
CURVE()
GEOMETRIC_REPRESENTATION_ITEM()
RATIONAL_B_SPLINE_CURVE((1.,1.0000133837799,1.00001075022011))
REPRESENTATION_ITEM('')
);
#19260=(
BOUNDED_CURVE()
B_SPLINE_CURVE(2,(#78079,#78080,#78081),.UNSPECIFIED.,.F.,.F.)
B_SPLINE_CURVE_WITH_KNOTS((3,3),(0.339146964126516,0.668418076018305),
 .UNSPECIFIED.)
CURVE()
GEOMETRIC_REPRESENTATION_ITEM()
RATIONAL_B_SPLINE_CURVE((1.00400190544534,1.00495889669788,1.00400190544534))
REPRESENTATION_ITEM('')
);
#19261=(
BOUNDED_CURVE()
B_SPLINE_CURVE(2,(#78083,#78084,#78085),.UNSPECIFIED.,.F.,.F.)
B_SPLINE_CURVE_WITH_KNOTS((3,3),(0.028463971978143,0.0708739951602902),
 .UNSPECIFIED.)
CURVE()
GEOMETRIC_REPRESENTATION_ITEM()
RATIONAL_B_SPLINE_CURVE((1.00001075215987,1.00001338619444,1.))
REPRESENTATION_ITEM('')
);
#19262=(
BOUNDED_CURVE()
B_SPLINE_CURVE(2,(#78089,#78090,#78091),.UNSPECIFIED.,.F.,.F.)
B_SPLINE_CURVE_WITH_KNOTS((3,3),(0.,0.0424100230241919),.UNSPECIFIED.)
CURVE()
GEOMETRIC_REPRESENTATION_ITEM()
RATIONAL_B_SPLINE_CURVE((1.,1.00001338577696,1.0000107518246))
REPRESENTATION_ITEM('')
);
#19263=(
BOUNDED_CURVE()
B_SPLINE_CURVE(2,(#78093,#78094,#78095),.UNSPECIFIED.,.F.,.F.)
B_SPLINE_CURVE_WITH_KNOTS((3,3),(0.339146964126515,0.668418076018303),
 .UNSPECIFIED.)
CURVE()
GEOMETRIC_REPRESENTATION_ITEM()
RATIONAL_B_SPLINE_CURVE((1.00400190544534,1.00495889669788,1.00400190544534))
REPRESENTATION_ITEM('')
);
#19264=(
BOUNDED_CURVE()
B_SPLINE_CURVE(2,(#78097,#78098,#78099),.UNSPECIFIED.,.F.,.F.)
B_SPLINE_CURVE_WITH_KNOTS((3,3),(0.0284639714085394,0.0708739951602901),
 .UNSPECIFIED.)
CURVE()
GEOMETRIC_REPRESENTATION_ITEM()
RATIONAL_B_SPLINE_CURVE((1.00001075029138,1.00001338386847,1.))
REPRESENTATION_ITEM('')
);
#19265=(
BOUNDED_CURVE()
B_SPLINE_CURVE(2,(#78103,#78104,#78105),.UNSPECIFIED.,.F.,.F.)
B_SPLINE_CURVE_WITH_KNOTS((3,3),(0.,0.0424100237528121),.UNSPECIFIED.)
CURVE()
GEOMETRIC_REPRESENTATION_ITEM()
RATIONAL_B_SPLINE_CURVE((1.,1.00001338452937,1.00001075082223))
REPRESENTATION_ITEM('')
);
#19266=(
BOUNDED_CURVE()
B_SPLINE_CURVE(2,(#78107,#78108,#78109),.UNSPECIFIED.,.F.,.F.)
B_SPLINE_CURVE_WITH_KNOTS((3,3),(0.33914696412652,0.668418076018306),
 .UNSPECIFIED.)
CURVE()
GEOMETRIC_REPRESENTATION_ITEM()
RATIONAL_B_SPLINE_CURVE((1.00400190544534,1.00495889669787,1.00400190544534))
REPRESENTATION_ITEM('')
);
#19267=(
BOUNDED_CURVE()
B_SPLINE_CURVE(2,(#78111,#78112,#78113),.UNSPECIFIED.,.F.,.F.)
B_SPLINE_CURVE_WITH_KNOTS((3,3),(0.0284639714357814,0.0708739951602905),
 .UNSPECIFIED.)
CURVE()
GEOMETRIC_REPRESENTATION_ITEM()
RATIONAL_B_SPLINE_CURVE((1.00001075147797,1.00001338534574,1.))
REPRESENTATION_ITEM('')
);
#19268=(
BOUNDED_CURVE()
B_SPLINE_CURVE(2,(#78117,#78118,#78119),.UNSPECIFIED.,.F.,.F.)
B_SPLINE_CURVE_WITH_KNOTS((3,3),(0.,0.0424100231755104),.UNSPECIFIED.)
CURVE()
GEOMETRIC_REPRESENTATION_ITEM()
RATIONAL_B_SPLINE_CURVE((1.,1.0000133853411,1.00001075147445))
REPRESENTATION_ITEM('')
);
#19269=(
BOUNDED_CURVE()
B_SPLINE_CURVE(2,(#78121,#78122,#78123),.UNSPECIFIED.,.F.,.F.)
B_SPLINE_CURVE_WITH_KNOTS((3,3),(0.339146964126517,0.668418076018305),
 .UNSPECIFIED.)
CURVE()
GEOMETRIC_REPRESENTATION_ITEM()
RATIONAL_B_SPLINE_CURVE((1.00400190544534,1.00495889669788,1.00400190544534))
REPRESENTATION_ITEM('')
);
#19270=(
BOUNDED_CURVE()
B_SPLINE_CURVE(2,(#78125,#78126,#78127),.UNSPECIFIED.,.F.,.F.)
B_SPLINE_CURVE_WITH_KNOTS((3,3),(0.0284639717634429,0.0708739951602899),
 .UNSPECIFIED.)
CURVE()
GEOMETRIC_REPRESENTATION_ITEM()
RATIONAL_B_SPLINE_CURVE((1.00001075157258,1.00001338546337,1.))
REPRESENTATION_ITEM('')
);
#19271=(
BOUNDED_CURVE()
B_SPLINE_CURVE(2,(#78131,#78132,#78133),.UNSPECIFIED.,.F.,.F.)
B_SPLINE_CURVE_WITH_KNOTS((3,3),(0.,0.0424100230054134),.UNSPECIFIED.)
CURVE()
GEOMETRIC_REPRESENTATION_ITEM()
RATIONAL_B_SPLINE_CURVE((1.,1.00001338465159,1.00001075092068))
REPRESENTATION_ITEM('')
);
#19272=(
BOUNDED_CURVE()
B_SPLINE_CURVE(2,(#78135,#78136,#78137),.UNSPECIFIED.,.F.,.F.)
B_SPLINE_CURVE_WITH_KNOTS((3,3),(0.339146964126518,0.668418076018304),
 .UNSPECIFIED.)
CURVE()
GEOMETRIC_REPRESENTATION_ITEM()
RATIONAL_B_SPLINE_CURVE((1.00400190544534,1.00495889669787,1.00400190544534))
REPRESENTATION_ITEM('')
);
#19273=(
BOUNDED_CURVE()
B_SPLINE_CURVE(2,(#78139,#78140,#78141),.UNSPECIFIED.,.F.,.F.)
B_SPLINE_CURVE_WITH_KNOTS((3,3),(0.0284639725451214,0.0708739951602902),
 .UNSPECIFIED.)
CURVE()
GEOMETRIC_REPRESENTATION_ITEM()
RATIONAL_B_SPLINE_CURVE((1.00001075152758,1.00001338540698,1.))
REPRESENTATION_ITEM('')
);
#19274=(
BOUNDED_CURVE()
B_SPLINE_CURVE(2,(#78145,#78146,#78147),.UNSPECIFIED.,.F.,.F.)
B_SPLINE_CURVE_WITH_KNOTS((3,3),(0.,0.042410022661541),.UNSPECIFIED.)
CURVE()
GEOMETRIC_REPRESENTATION_ITEM()
RATIONAL_B_SPLINE_CURVE((1.,1.00001338471694,1.0000107509733))
REPRESENTATION_ITEM('')
);
#19275=(
BOUNDED_CURVE()
B_SPLINE_CURVE(2,(#78149,#78150,#78151),.UNSPECIFIED.,.F.,.F.)
B_SPLINE_CURVE_WITH_KNOTS((3,3),(0.339146964126513,0.668418076018301),
 .UNSPECIFIED.)
CURVE()
GEOMETRIC_REPRESENTATION_ITEM()
RATIONAL_B_SPLINE_CURVE((1.00400190544534,1.00495889669788,1.00400190544534))
REPRESENTATION_ITEM('')
);
#19276=(
BOUNDED_CURVE()
B_SPLINE_CURVE(2,(#78153,#78154,#78155),.UNSPECIFIED.,.F.,.F.)
B_SPLINE_CURVE_WITH_KNOTS((3,3),(0.0284639712817304,0.0708739951602903),
 .UNSPECIFIED.)
CURVE()
GEOMETRIC_REPRESENTATION_ITEM()
RATIONAL_B_SPLINE_CURVE((1.00001075092078,1.00001338465212,1.))
REPRESENTATION_ITEM('')
);
#19277=(
BOUNDED_CURVE()
B_SPLINE_CURVE(2,(#78159,#78160,#78161),.UNSPECIFIED.,.F.,.F.)
B_SPLINE_CURVE_WITH_KNOTS((3,3),(0.,0.0424100230249418),.UNSPECIFIED.)
CURVE()
GEOMETRIC_REPRESENTATION_ITEM()
RATIONAL_B_SPLINE_CURVE((1.,1.00001338592286,1.0000107519418))
REPRESENTATION_ITEM('')
);
#19278=(
BOUNDED_CURVE()
B_SPLINE_CURVE(2,(#78163,#78164,#78165),.UNSPECIFIED.,.F.,.F.)
B_SPLINE_CURVE_WITH_KNOTS((3,3),(0.339146964126504,0.668418076018296),
 .UNSPECIFIED.)
CURVE()
GEOMETRIC_REPRESENTATION_ITEM()
RATIONAL_B_SPLINE_CURVE((1.00400190544536,1.0049588966979,1.00400190544536))
REPRESENTATION_ITEM('')
);
#19279=(
BOUNDED_CURVE()
B_SPLINE_CURVE(2,(#78167,#78168,#78169),.UNSPECIFIED.,.F.,.F.)
B_SPLINE_CURVE_WITH_KNOTS((3,3),(0.0284639714045715,0.0708739951602901),
 .UNSPECIFIED.)
CURVE()
GEOMETRIC_REPRESENTATION_ITEM()
RATIONAL_B_SPLINE_CURVE((1.00001075086984,1.00001338458864,1.))
REPRESENTATION_ITEM('')
);
#19280=(
BOUNDED_CURVE()
B_SPLINE_CURVE(2,(#78173,#78174,#78175),.UNSPECIFIED.,.F.,.F.)
B_SPLINE_CURVE_WITH_KNOTS((3,3),(0.,0.042410023759092),.UNSPECIFIED.)
CURVE()
GEOMETRIC_REPRESENTATION_ITEM()
RATIONAL_B_SPLINE_CURVE((1.,1.00001338518135,1.00001075134592))
REPRESENTATION_ITEM('')
);
#19281=(
BOUNDED_CURVE()
B_SPLINE_CURVE(2,(#78177,#78178,#78179),.UNSPECIFIED.,.F.,.F.)
B_SPLINE_CURVE_WITH_KNOTS((3,3),(0.339146964126521,0.668418076018308),
 .UNSPECIFIED.)
CURVE()
GEOMETRIC_REPRESENTATION_ITEM()
RATIONAL_B_SPLINE_CURVE((1.00400190544534,1.00495889669787,1.00400190544534))
REPRESENTATION_ITEM('')
);
#19282=(
BOUNDED_CURVE()
B_SPLINE_CURVE(2,(#78181,#78182,#78183),.UNSPECIFIED.,.F.,.F.)
B_SPLINE_CURVE_WITH_KNOTS((3,3),(0.0284639721328031,0.0708739951602905),
 .UNSPECIFIED.)
CURVE()
GEOMETRIC_REPRESENTATION_ITEM()
RATIONAL_B_SPLINE_CURVE((1.00001075159191,1.00001338548726,1.))
REPRESENTATION_ITEM('')
);
#19283=(
BOUNDED_CURVE()
B_SPLINE_CURVE(2,(#78187,#78188,#78189),.UNSPECIFIED.,.F.,.F.)
B_SPLINE_CURVE_WITH_KNOTS((3,3),(0.,0.0424100231470919),.UNSPECIFIED.)
CURVE()
GEOMETRIC_REPRESENTATION_ITEM()
RATIONAL_B_SPLINE_CURVE((1.,1.00001338447535,1.00001075077907))
REPRESENTATION_ITEM('')
);
#19284=(
BOUNDED_CURVE()
B_SPLINE_CURVE(2,(#78191,#78192,#78193),.UNSPECIFIED.,.F.,.F.)
B_SPLINE_CURVE_WITH_KNOTS((3,3),(0.339146964126509,0.668418076018305),
 .UNSPECIFIED.)
CURVE()
GEOMETRIC_REPRESENTATION_ITEM()
RATIONAL_B_SPLINE_CURVE((1.00400190544537,1.00495889669791,1.00400190544537))
REPRESENTATION_ITEM('')
);
#19285=(
BOUNDED_CURVE()
B_SPLINE_CURVE(2,(#78195,#78196,#78197),.UNSPECIFIED.,.F.,.F.)
B_SPLINE_CURVE_WITH_KNOTS((3,3),(0.0284639710994826,0.0708739951602903),
 .UNSPECIFIED.)
CURVE()
GEOMETRIC_REPRESENTATION_ITEM()
RATIONAL_B_SPLINE_CURVE((1.00001075063279,1.00001338429367,1.))
REPRESENTATION_ITEM('')
);
#19286=(
BOUNDED_CURVE()
B_SPLINE_CURVE(2,(#78201,#78202,#78203),.UNSPECIFIED.,.F.,.F.)
B_SPLINE_CURVE_WITH_KNOTS((3,3),(0.,0.0424100229366385),.UNSPECIFIED.)
CURVE()
GEOMETRIC_REPRESENTATION_ITEM()
RATIONAL_B_SPLINE_CURVE((1.,1.00001338458235,1.00001075086509))
REPRESENTATION_ITEM('')
);
#19287=(
BOUNDED_CURVE()
B_SPLINE_CURVE(2,(#78205,#78206,#78207),.UNSPECIFIED.,.F.,.F.)
B_SPLINE_CURVE_WITH_KNOTS((3,3),(0.339146964126511,0.668418076018304),
 .UNSPECIFIED.)
CURVE()
GEOMETRIC_REPRESENTATION_ITEM()
RATIONAL_B_SPLINE_CURVE((1.00400190544536,1.0049588966979,1.00400190544536))
REPRESENTATION_ITEM('')
);
#19288=(
BOUNDED_CURVE()
B_SPLINE_CURVE(2,(#78209,#78210,#78211),.UNSPECIFIED.,.F.,.F.)
B_SPLINE_CURVE_WITH_KNOTS((3,3),(0.0284639718437778,0.0708739951602902),
 .UNSPECIFIED.)
CURVE()
GEOMETRIC_REPRESENTATION_ITEM()
RATIONAL_B_SPLINE_CURVE((1.00001075112877,1.00001338491081,1.))
REPRESENTATION_ITEM('')
);
#19289=(
BOUNDED_CURVE()
B_SPLINE_CURVE(2,(#78215,#78216,#78217),.UNSPECIFIED.,.F.,.F.)
B_SPLINE_CURVE_WITH_KNOTS((3,3),(0.,0.0424100231273197),.UNSPECIFIED.)
CURVE()
GEOMETRIC_REPRESENTATION_ITEM()
RATIONAL_B_SPLINE_CURVE((1.,1.00001338514488,1.00001075131686))
REPRESENTATION_ITEM('')
);
#19290=(
BOUNDED_CURVE()
B_SPLINE_CURVE(2,(#78219,#78220,#78221),.UNSPECIFIED.,.F.,.F.)
B_SPLINE_CURVE_WITH_KNOTS((3,3),(0.339146964126517,0.668418076018305),
 .UNSPECIFIED.)
CURVE()
GEOMETRIC_REPRESENTATION_ITEM()
RATIONAL_B_SPLINE_CURVE((1.00400190544534,1.00495889669788,1.00400190544534))
REPRESENTATION_ITEM('')
);
#19291=(
BOUNDED_CURVE()
B_SPLINE_CURVE(2,(#78223,#78224,#78225),.UNSPECIFIED.,.F.,.F.)
B_SPLINE_CURVE_WITH_KNOTS((3,3),(0.028463971590667,0.0708739951602901),
 .UNSPECIFIED.)
CURVE()
GEOMETRIC_REPRESENTATION_ITEM()
RATIONAL_B_SPLINE_CURVE((1.00001075154508,1.00001338542922,1.))
REPRESENTATION_ITEM('')
);
#19292=(
BOUNDED_CURVE()
B_SPLINE_CURVE(2,(#78229,#78230,#78231),.UNSPECIFIED.,.F.,.F.)
B_SPLINE_CURVE_WITH_KNOTS((3,3),(0.,0.042410023865277),.UNSPECIFIED.)
CURVE()
GEOMETRIC_REPRESENTATION_ITEM()
RATIONAL_B_SPLINE_CURVE((1.,1.00001338530686,1.00001075144669))
REPRESENTATION_ITEM('')
);
#19293=(
BOUNDED_CURVE()
B_SPLINE_CURVE(2,(#78233,#78234,#78235),.UNSPECIFIED.,.F.,.F.)
B_SPLINE_CURVE_WITH_KNOTS((3,3),(0.339146964126508,0.668418076018304),
 .UNSPECIFIED.)
CURVE()
GEOMETRIC_REPRESENTATION_ITEM()
RATIONAL_B_SPLINE_CURVE((1.00400190544537,1.00495889669791,1.00400190544537))
REPRESENTATION_ITEM('')
);
#19294=(
BOUNDED_CURVE()
B_SPLINE_CURVE(2,(#78237,#78238,#78239),.UNSPECIFIED.,.F.,.F.)
B_SPLINE_CURVE_WITH_KNOTS((3,3),(0.0284639715344571,0.0708739951602902),
 .UNSPECIFIED.)
CURVE()
GEOMETRIC_REPRESENTATION_ITEM()
RATIONAL_B_SPLINE_CURVE((1.0000107510557,1.00001338481998,1.))
REPRESENTATION_ITEM('')
);
#19295=(
BOUNDED_CURVE()
B_SPLINE_CURVE(2,(#78243,#78244,#78245),.UNSPECIFIED.,.F.,.F.)
B_SPLINE_CURVE_WITH_KNOTS((3,3),(0.,0.0424100228518102),.UNSPECIFIED.)
CURVE()
GEOMETRIC_REPRESENTATION_ITEM()
RATIONAL_B_SPLINE_CURVE((1.,1.00001338581925,1.00001075185864))
REPRESENTATION_ITEM('')
);
#19296=(
BOUNDED_CURVE()
B_SPLINE_CURVE(2,(#78247,#78248,#78249),.UNSPECIFIED.,.F.,.F.)
B_SPLINE_CURVE_WITH_KNOTS((3,3),(0.339146964126521,0.668418076018307),
 .UNSPECIFIED.)
CURVE()
GEOMETRIC_REPRESENTATION_ITEM()
RATIONAL_B_SPLINE_CURVE((1.00400190544534,1.00495889669787,1.00400190544534))
REPRESENTATION_ITEM('')
);
#19297=(
BOUNDED_CURVE()
B_SPLINE_CURVE(2,(#78251,#78252,#78253),.UNSPECIFIED.,.F.,.F.)
B_SPLINE_CURVE_WITH_KNOTS((3,3),(0.0284639711204301,0.0708739951602906),
 .UNSPECIFIED.)
CURVE()
GEOMETRIC_REPRESENTATION_ITEM()
RATIONAL_B_SPLINE_CURVE((1.00001075034871,1.00001338393999,1.))
REPRESENTATION_ITEM('')
);
#19298=(
BOUNDED_CURVE()
B_SPLINE_CURVE(2,(#78257,#78258,#78259),.UNSPECIFIED.,.F.,.F.)
B_SPLINE_CURVE_WITH_KNOTS((3,3),(0.,0.0424100240197507),.UNSPECIFIED.)
CURVE()
GEOMETRIC_REPRESENTATION_ITEM()
RATIONAL_B_SPLINE_CURVE((1.,1.00001338509862,1.00001075127937))
REPRESENTATION_ITEM('')
);
#19299=(
BOUNDED_CURVE()
B_SPLINE_CURVE(2,(#78261,#78262,#78263),.UNSPECIFIED.,.F.,.F.)
B_SPLINE_CURVE_WITH_KNOTS((3,3),(0.339146964126524,0.668418076018308),
 .UNSPECIFIED.)
CURVE()
GEOMETRIC_REPRESENTATION_ITEM()
RATIONAL_B_SPLINE_CURVE((1.00400190544533,1.00495889669787,1.00400190544533))
REPRESENTATION_ITEM('')
);
#19300=(
BOUNDED_CURVE()
B_SPLINE_CURVE(2,(#78265,#78266,#78267),.UNSPECIFIED.,.F.,.F.)
B_SPLINE_CURVE_WITH_KNOTS((3,3),(0.0284639714437082,0.0708739951602905),
 .UNSPECIFIED.)
CURVE()
GEOMETRIC_REPRESENTATION_ITEM()
RATIONAL_B_SPLINE_CURVE((1.00001075074537,1.00001338443367,1.))
REPRESENTATION_ITEM('')
);
#19301=(
BOUNDED_CURVE()
B_SPLINE_CURVE(2,(#78271,#78272,#78273),.UNSPECIFIED.,.F.,.F.)
B_SPLINE_CURVE_WITH_KNOTS((3,3),(0.,0.0424100234119021),.UNSPECIFIED.)
CURVE()
GEOMETRIC_REPRESENTATION_ITEM()
RATIONAL_B_SPLINE_CURVE((1.,1.00001338567679,1.000010751744))
REPRESENTATION_ITEM('')
);
#19302=(
BOUNDED_CURVE()
B_SPLINE_CURVE(2,(#78275,#78276,#78277),.UNSPECIFIED.,.F.,.F.)
B_SPLINE_CURVE_WITH_KNOTS((3,3),(0.339146964126514,0.668418076018306),
 .UNSPECIFIED.)
CURVE()
GEOMETRIC_REPRESENTATION_ITEM()
RATIONAL_B_SPLINE_CURVE((1.00400190544536,1.0049588966979,1.00400190544536))
REPRESENTATION_ITEM('')
);
#19303=(
BOUNDED_CURVE()
B_SPLINE_CURVE(2,(#78279,#78280,#78281),.UNSPECIFIED.,.F.,.F.)
B_SPLINE_CURVE_WITH_KNOTS((3,3),(0.0284639720122614,0.0708739951602903),
 .UNSPECIFIED.)
CURVE()
GEOMETRIC_REPRESENTATION_ITEM()
RATIONAL_B_SPLINE_CURVE((1.00001075146677,1.00001338533152,1.))
REPRESENTATION_ITEM('')
);
#19304=(
BOUNDED_CURVE()
B_SPLINE_CURVE(2,(#78285,#78286,#78287),.UNSPECIFIED.,.F.,.F.)
B_SPLINE_CURVE_WITH_KNOTS((3,3),(0.,0.0424100244197339),.UNSPECIFIED.)
CURVE()
GEOMETRIC_REPRESENTATION_ITEM()
RATIONAL_B_SPLINE_CURVE((1.,1.00001338512157,1.00001075129765))
REPRESENTATION_ITEM('')
);
#19305=(
BOUNDED_CURVE()
B_SPLINE_CURVE(2,(#78289,#78290,#78291),.UNSPECIFIED.,.F.,.F.)
B_SPLINE_CURVE_WITH_KNOTS((3,3),(0.339146964126511,0.668418076018303),
 .UNSPECIFIED.)
CURVE()
GEOMETRIC_REPRESENTATION_ITEM()
RATIONAL_B_SPLINE_CURVE((1.00400190544536,1.0049588966979,1.00400190544536))
REPRESENTATION_ITEM('')
);
#19306=(
BOUNDED_CURVE()
B_SPLINE_CURVE(2,(#78293,#78294,#78295),.UNSPECIFIED.,.F.,.F.)
B_SPLINE_CURVE_WITH_KNOTS((3,3),(0.0284639714088168,0.0708739951602901),
 .UNSPECIFIED.)
CURVE()
GEOMETRIC_REPRESENTATION_ITEM()
RATIONAL_B_SPLINE_CURVE((1.00001075122115,1.00001338502601,1.))
REPRESENTATION_ITEM('')
);
#19307=(
BOUNDED_CURVE()
B_SPLINE_CURVE(2,(#78299,#78300,#78301),.UNSPECIFIED.,.F.,.F.)
B_SPLINE_CURVE_WITH_KNOTS((3,3),(0.,0.0709397118056798),.UNSPECIFIED.)
CURVE()
GEOMETRIC_REPRESENTATION_ITEM()
RATIONAL_B_SPLINE_CURVE((1.,1.0000224517311,1.))
REPRESENTATION_ITEM('')
);
#19308=(
BOUNDED_CURVE()
B_SPLINE_CURVE(2,(#78309,#78310,#78311),.UNSPECIFIED.,.F.,.F.)
B_SPLINE_CURVE_WITH_KNOTS((3,3),(0.,0.0424100231806302),.UNSPECIFIED.)
CURVE()
GEOMETRIC_REPRESENTATION_ITEM()
RATIONAL_B_SPLINE_CURVE((1.,1.00001338421203,1.00001075056755))
REPRESENTATION_ITEM('')
);
#19309=(
BOUNDED_CURVE()
B_SPLINE_CURVE(2,(#78313,#78314,#78315),.UNSPECIFIED.,.F.,.F.)
B_SPLINE_CURVE_WITH_KNOTS((3,3),(0.339146964126513,0.668418076018302),
 .UNSPECIFIED.)
CURVE()
GEOMETRIC_REPRESENTATION_ITEM()
RATIONAL_B_SPLINE_CURVE((1.00400190544535,1.00495889669789,1.00400190544535))
REPRESENTATION_ITEM('')
);
#19310=(
BOUNDED_CURVE()
B_SPLINE_CURVE(2,(#78317,#78318,#78319),.UNSPECIFIED.,.F.,.F.)
B_SPLINE_CURVE_WITH_KNOTS((3,3),(0.0284639714379858,0.0708739951602898),
 .UNSPECIFIED.)
CURVE()
GEOMETRIC_REPRESENTATION_ITEM()
RATIONAL_B_SPLINE_CURVE((1.00001075041393,1.00001338402103,1.))
REPRESENTATION_ITEM('')
);
#19311=(
BOUNDED_CURVE()
B_SPLINE_CURVE(2,(#78323,#78324,#78325),.UNSPECIFIED.,.F.,.F.)
B_SPLINE_CURVE_WITH_KNOTS((3,3),(0.,0.0424100233991719),.UNSPECIFIED.)
CURVE()
GEOMETRIC_REPRESENTATION_ITEM()
RATIONAL_B_SPLINE_CURVE((1.,1.00001338583662,1.00001075187238))
REPRESENTATION_ITEM('')
);
#19312=(
BOUNDED_CURVE()
B_SPLINE_CURVE(2,(#78327,#78328,#78329),.UNSPECIFIED.,.F.,.F.)
B_SPLINE_CURVE_WITH_KNOTS((3,3),(0.339146964126513,0.668418076018302),
 .UNSPECIFIED.)
CURVE()
GEOMETRIC_REPRESENTATION_ITEM()
RATIONAL_B_SPLINE_CURVE((1.00400190544535,1.00495889669789,1.00400190544535))
REPRESENTATION_ITEM('')
);
#19313=(
BOUNDED_CURVE()
B_SPLINE_CURVE(2,(#78331,#78332,#78333),.UNSPECIFIED.,.F.,.F.)
B_SPLINE_CURVE_WITH_KNOTS((3,3),(0.0284639720344373,0.0708739951602892),
 .UNSPECIFIED.)
CURVE()
GEOMETRIC_REPRESENTATION_ITEM()
RATIONAL_B_SPLINE_CURVE((1.00001075214126,1.00001338617124,1.))
REPRESENTATION_ITEM('')
);
#19314=(
BOUNDED_CURVE()
B_SPLINE_CURVE(2,(#78337,#78338,#78339),.UNSPECIFIED.,.F.,.F.)
B_SPLINE_CURVE_WITH_KNOTS((3,3),(0.,0.0424100237328626),.UNSPECIFIED.)
CURVE()
GEOMETRIC_REPRESENTATION_ITEM()
RATIONAL_B_SPLINE_CURVE((1.,1.00001338671567,1.00001075257833))
REPRESENTATION_ITEM('')
);
#19315=(
BOUNDED_CURVE()
B_SPLINE_CURVE(2,(#78341,#78342,#78343),.UNSPECIFIED.,.F.,.F.)
B_SPLINE_CURVE_WITH_KNOTS((3,3),(0.339146964126522,0.668418076018309),
 .UNSPECIFIED.)
CURVE()
GEOMETRIC_REPRESENTATION_ITEM()
RATIONAL_B_SPLINE_CURVE((1.00400190544534,1.00495889669788,1.00400190544534))
REPRESENTATION_ITEM('')
);
#19316=(
BOUNDED_CURVE()
B_SPLINE_CURVE(2,(#78345,#78346,#78347),.UNSPECIFIED.,.F.,.F.)
B_SPLINE_CURVE_WITH_KNOTS((3,3),(0.0284639721094118,0.0708739951602891),
 .UNSPECIFIED.)
CURVE()
GEOMETRIC_REPRESENTATION_ITEM()
RATIONAL_B_SPLINE_CURVE((1.00001075120572,1.00001338500648,1.))
REPRESENTATION_ITEM('')
);
#19317=(
BOUNDED_CURVE()
B_SPLINE_CURVE(2,(#78351,#78352,#78353),.UNSPECIFIED.,.F.,.F.)
B_SPLINE_CURVE_WITH_KNOTS((3,3),(0.,0.0424100230569424),.UNSPECIFIED.)
CURVE()
GEOMETRIC_REPRESENTATION_ITEM()
RATIONAL_B_SPLINE_CURVE((1.,1.00001338564898,1.00001075172179))
REPRESENTATION_ITEM('')
);
#19318=(
BOUNDED_CURVE()
B_SPLINE_CURVE(2,(#78355,#78356,#78357),.UNSPECIFIED.,.F.,.F.)
B_SPLINE_CURVE_WITH_KNOTS((3,3),(0.339146964126515,0.668418076018298),
 .UNSPECIFIED.)
CURVE()
GEOMETRIC_REPRESENTATION_ITEM()
RATIONAL_B_SPLINE_CURVE((1.00400190544533,1.00495889669786,1.00400190544533))
REPRESENTATION_ITEM('')
);
#19319=(
BOUNDED_CURVE()
B_SPLINE_CURVE(2,(#78359,#78360,#78361),.UNSPECIFIED.,.F.,.F.)
B_SPLINE_CURVE_WITH_KNOTS((3,3),(0.0284639721324363,0.0708739951602891),
 .UNSPECIFIED.)
CURVE()
GEOMETRIC_REPRESENTATION_ITEM()
RATIONAL_B_SPLINE_CURVE((1.00001075234275,1.00001338642205,1.))
REPRESENTATION_ITEM('')
);
#19320=(
BOUNDED_CURVE()
B_SPLINE_CURVE(2,(#78365,#78366,#78367),.UNSPECIFIED.,.F.,.F.)
B_SPLINE_CURVE_WITH_KNOTS((3,3),(0.,0.0424100231045523),.UNSPECIFIED.)
CURVE()
GEOMETRIC_REPRESENTATION_ITEM()
RATIONAL_B_SPLINE_CURVE((1.,1.00001338428089,1.00001075062289))
REPRESENTATION_ITEM('')
);
#19321=(
BOUNDED_CURVE()
B_SPLINE_CURVE(2,(#78369,#78370,#78371),.UNSPECIFIED.,.F.,.F.)
B_SPLINE_CURVE_WITH_KNOTS((3,3),(0.339146964126512,0.668418076018305),
 .UNSPECIFIED.)
CURVE()
GEOMETRIC_REPRESENTATION_ITEM()
RATIONAL_B_SPLINE_CURVE((1.00400190544536,1.0049588966979,1.00400190544536))
REPRESENTATION_ITEM('')
);
#19322=(
BOUNDED_CURVE()
B_SPLINE_CURVE(2,(#78373,#78374,#78375),.UNSPECIFIED.,.F.,.F.)
B_SPLINE_CURVE_WITH_KNOTS((3,3),(0.0284639718061504,0.0708739951602889),
 .UNSPECIFIED.)
CURVE()
GEOMETRIC_REPRESENTATION_ITEM()
RATIONAL_B_SPLINE_CURVE((1.0000107509097,1.00001338463808,1.))
REPRESENTATION_ITEM('')
);
#19323=(
BOUNDED_CURVE()
B_SPLINE_CURVE(2,(#78379,#78380,#78381),.UNSPECIFIED.,.F.,.F.)
B_SPLINE_CURVE_WITH_KNOTS((3,3),(0.,0.0424100237189079),.UNSPECIFIED.)
CURVE()
GEOMETRIC_REPRESENTATION_ITEM()
RATIONAL_B_SPLINE_CURVE((1.,1.00001338362396,1.00001075009499))
REPRESENTATION_ITEM('')
);
#19324=(
BOUNDED_CURVE()
B_SPLINE_CURVE(2,(#78383,#78384,#78385),.UNSPECIFIED.,.F.,.F.)
B_SPLINE_CURVE_WITH_KNOTS((3,3),(0.339146964126514,0.668418076018301),
 .UNSPECIFIED.)
CURVE()
GEOMETRIC_REPRESENTATION_ITEM()
RATIONAL_B_SPLINE_CURVE((1.00400190544534,1.00495889669788,1.00400190544534))
REPRESENTATION_ITEM('')
);
#19325=(
BOUNDED_CURVE()
B_SPLINE_CURVE(2,(#78387,#78388,#78389),.UNSPECIFIED.,.F.,.F.)
B_SPLINE_CURVE_WITH_KNOTS((3,3),(0.0284639710964825,0.0708739951602894),
 .UNSPECIFIED.)
CURVE()
GEOMETRIC_REPRESENTATION_ITEM()
RATIONAL_B_SPLINE_CURVE((1.00001075212803,1.00001338615521,1.))
REPRESENTATION_ITEM('')
);
#19326=(
BOUNDED_CURVE()
B_SPLINE_CURVE(2,(#78393,#78394,#78395),.UNSPECIFIED.,.F.,.F.)
B_SPLINE_CURVE_WITH_KNOTS((3,3),(0.,0.0424100233501915),.UNSPECIFIED.)
CURVE()
GEOMETRIC_REPRESENTATION_ITEM()
RATIONAL_B_SPLINE_CURVE((1.,1.00001338506266,1.00001075125073))
REPRESENTATION_ITEM('')
);
#19327=(
BOUNDED_CURVE()
B_SPLINE_CURVE(2,(#78397,#78398,#78399),.UNSPECIFIED.,.F.,.F.)
B_SPLINE_CURVE_WITH_KNOTS((3,3),(0.339146964126518,0.668418076018306),
 .UNSPECIFIED.)
CURVE()
GEOMETRIC_REPRESENTATION_ITEM()
RATIONAL_B_SPLINE_CURVE((1.00400190544534,1.00495889669788,1.00400190544534))
REPRESENTATION_ITEM('')
);
#19328=(
BOUNDED_CURVE()
B_SPLINE_CURVE(2,(#78401,#78402,#78403),.UNSPECIFIED.,.F.,.F.)
B_SPLINE_CURVE_WITH_KNOTS((3,3),(0.0284639717818257,0.0708739951602895),
 .UNSPECIFIED.)
CURVE()
GEOMETRIC_REPRESENTATION_ITEM()
RATIONAL_B_SPLINE_CURVE((1.00001075166044,1.00001338557275,1.))
REPRESENTATION_ITEM('')
);
#19329=(
BOUNDED_CURVE()
B_SPLINE_CURVE(2,(#78407,#78408,#78409),.UNSPECIFIED.,.F.,.F.)
B_SPLINE_CURVE_WITH_KNOTS((3,3),(0.,0.0424100231031821),.UNSPECIFIED.)
CURVE()
GEOMETRIC_REPRESENTATION_ITEM()
RATIONAL_B_SPLINE_CURVE((1.,1.00001338538099,1.00001075150652))
REPRESENTATION_ITEM('')
);
#19330=(
BOUNDED_CURVE()
B_SPLINE_CURVE(2,(#78411,#78412,#78413),.UNSPECIFIED.,.F.,.F.)
B_SPLINE_CURVE_WITH_KNOTS((3,3),(0.339146964126511,0.668418076018296),
 .UNSPECIFIED.)
CURVE()
GEOMETRIC_REPRESENTATION_ITEM()
RATIONAL_B_SPLINE_CURVE((1.00400190544533,1.00495889669787,1.00400190544533))
REPRESENTATION_ITEM('')
);
#19331=(
BOUNDED_CURVE()
B_SPLINE_CURVE(2,(#78415,#78416,#78417),.UNSPECIFIED.,.F.,.F.)
B_SPLINE_CURVE_WITH_KNOTS((3,3),(0.0284639708342344,0.0708739951602889),
 .UNSPECIFIED.)
CURVE()
GEOMETRIC_REPRESENTATION_ITEM()
RATIONAL_B_SPLINE_CURVE((1.00001075087742,1.00001338459835,1.))
REPRESENTATION_ITEM('')
);
#19332=(
BOUNDED_CURVE()
B_SPLINE_CURVE(2,(#78421,#78422,#78423),.UNSPECIFIED.,.F.,.F.)
B_SPLINE_CURVE_WITH_KNOTS((3,3),(0.,0.0424100228599136),.UNSPECIFIED.)
CURVE()
GEOMETRIC_REPRESENTATION_ITEM()
RATIONAL_B_SPLINE_CURVE((1.,1.00001338560217,1.00001075168427))
REPRESENTATION_ITEM('')
);
#19333=(
BOUNDED_CURVE()
B_SPLINE_CURVE(2,(#78425,#78426,#78427),.UNSPECIFIED.,.F.,.F.)
B_SPLINE_CURVE_WITH_KNOTS((3,3),(0.339146964126524,0.668418076018308),
 .UNSPECIFIED.)
CURVE()
GEOMETRIC_REPRESENTATION_ITEM()
RATIONAL_B_SPLINE_CURVE((1.00400190544533,1.00495889669787,1.00400190544533))
REPRESENTATION_ITEM('')
);
#19334=(
BOUNDED_CURVE()
B_SPLINE_CURVE(2,(#78429,#78430,#78431),.UNSPECIFIED.,.F.,.F.)
B_SPLINE_CURVE_WITH_KNOTS((3,3),(0.0284639720345148,0.0708739951602895),
 .UNSPECIFIED.)
CURVE()
GEOMETRIC_REPRESENTATION_ITEM()
RATIONAL_B_SPLINE_CURVE((1.00001075173436,1.00001338566466,1.))
REPRESENTATION_ITEM('')
);
#19335=(
BOUNDED_CURVE()
B_SPLINE_CURVE(2,(#78435,#78436,#78437),.UNSPECIFIED.,.F.,.F.)
B_SPLINE_CURVE_WITH_KNOTS((3,3),(0.,0.0424100233282264),.UNSPECIFIED.)
CURVE()
GEOMETRIC_REPRESENTATION_ITEM()
RATIONAL_B_SPLINE_CURVE((1.,1.00001338433303,1.00001075066468))
REPRESENTATION_ITEM('')
);
#19336=(
BOUNDED_CURVE()
B_SPLINE_CURVE(2,(#78439,#78440,#78441),.UNSPECIFIED.,.F.,.F.)
B_SPLINE_CURVE_WITH_KNOTS((3,3),(0.339146964126518,0.668418076018304),
 .UNSPECIFIED.)
CURVE()
GEOMETRIC_REPRESENTATION_ITEM()
RATIONAL_B_SPLINE_CURVE((1.00400190544534,1.00495889669788,1.00400190544534))
REPRESENTATION_ITEM('')
);
#19337=(
BOUNDED_CURVE()
B_SPLINE_CURVE(2,(#78443,#78444,#78445),.UNSPECIFIED.,.F.,.F.)
B_SPLINE_CURVE_WITH_KNOTS((3,3),(0.028463971433294,0.0708739951602898),
 .UNSPECIFIED.)
CURVE()
GEOMETRIC_REPRESENTATION_ITEM()
RATIONAL_B_SPLINE_CURVE((1.00001075098432,1.00001338473115,1.))
REPRESENTATION_ITEM('')
);
#19338=(
BOUNDED_CURVE()
B_SPLINE_CURVE(2,(#78449,#78450,#78451),.UNSPECIFIED.,.F.,.F.)
B_SPLINE_CURVE_WITH_KNOTS((3,3),(0.,0.042410024098998),.UNSPECIFIED.)
CURVE()
GEOMETRIC_REPRESENTATION_ITEM()
RATIONAL_B_SPLINE_CURVE((1.,1.00001338512572,1.0000107513011))
REPRESENTATION_ITEM('')
);
#19339=(
BOUNDED_CURVE()
B_SPLINE_CURVE(2,(#78453,#78454,#78455),.UNSPECIFIED.,.F.,.F.)
B_SPLINE_CURVE_WITH_KNOTS((3,3),(0.33914696412651,0.668418076018299),
 .UNSPECIFIED.)
CURVE()
GEOMETRIC_REPRESENTATION_ITEM()
RATIONAL_B_SPLINE_CURVE((1.00400190544535,1.00495889669788,1.00400190544535))
REPRESENTATION_ITEM('')
);
#19340=(
BOUNDED_CURVE()
B_SPLINE_CURVE(2,(#78457,#78458,#78459),.UNSPECIFIED.,.F.,.F.)
B_SPLINE_CURVE_WITH_KNOTS((3,3),(0.0284639719730562,0.0708739951602891),
 .UNSPECIFIED.)
CURVE()
GEOMETRIC_REPRESENTATION_ITEM()
RATIONAL_B_SPLINE_CURVE((1.00001075041269,1.00001338401924,1.))
REPRESENTATION_ITEM('')
);
#19341=(
BOUNDED_CURVE()
B_SPLINE_CURVE(2,(#78462,#78463,#78464),.UNSPECIFIED.,.F.,.F.)
B_SPLINE_CURVE_WITH_KNOTS((3,3),(0.,0.0709397118056796),.UNSPECIFIED.)
CURVE()
GEOMETRIC_REPRESENTATION_ITEM()
RATIONAL_B_SPLINE_CURVE((1.,1.00002245188718,1.))
REPRESENTATION_ITEM('')
);
#19342=(
BOUNDED_CURVE()
B_SPLINE_CURVE(2,(#78482,#78483,#78484),.UNSPECIFIED.,.F.,.F.)
B_SPLINE_CURVE_WITH_KNOTS((3,3),(0.072859873218516,0.164428174992087),
 .UNSPECIFIED.)
CURVE()
GEOMETRIC_REPRESENTATION_ITEM()
RATIONAL_B_SPLINE_CURVE((1.00004422028548,1.00004989756719,1.))
REPRESENTATION_ITEM('')
);
#19343=(
BOUNDED_CURVE()
B_SPLINE_CURVE(2,(#78486,#78487,#78488),.UNSPECIFIED.,.F.,.F.)
B_SPLINE_CURVE_WITH_KNOTS((3,3),(0.526544758504317,0.808610241550327),
 .UNSPECIFIED.)
CURVE()
GEOMETRIC_REPRESENTATION_ITEM()
RATIONAL_B_SPLINE_CURVE((1.00594694470058,1.00650257927329,1.00594694470058))
REPRESENTATION_ITEM('')
);
#19344=(
BOUNDED_CURVE()
B_SPLINE_CURVE(2,(#78490,#78491,#78492),.UNSPECIFIED.,.F.,.F.)
B_SPLINE_CURVE_WITH_KNOTS((3,3),(0.,0.0915683011616728),.UNSPECIFIED.)
CURVE()
GEOMETRIC_REPRESENTATION_ITEM()
RATIONAL_B_SPLINE_CURVE((1.,1.00004989745095,1.00004422018284))
REPRESENTATION_ITEM('')
);
#19345=(
BOUNDED_CURVE()
B_SPLINE_CURVE(2,(#78497,#78498,#78499),.UNSPECIFIED.,.F.,.F.)
B_SPLINE_CURVE_WITH_KNOTS((3,3),(0.0728598736698146,0.164428174992088),
 .UNSPECIFIED.)
CURVE()
GEOMETRIC_REPRESENTATION_ITEM()
RATIONAL_B_SPLINE_CURVE((1.00004421982567,1.00004989704804,1.))
REPRESENTATION_ITEM('')
);
#19346=(
BOUNDED_CURVE()
B_SPLINE_CURVE(2,(#78501,#78502,#78503),.UNSPECIFIED.,.F.,.F.)
B_SPLINE_CURVE_WITH_KNOTS((3,3),(0.526544758504314,0.808610241550329),
 .UNSPECIFIED.)
CURVE()
GEOMETRIC_REPRESENTATION_ITEM()
RATIONAL_B_SPLINE_CURVE((1.00594694470059,1.00650257927331,1.00594694470059))
REPRESENTATION_ITEM('')
);
#19347=(
BOUNDED_CURVE()
B_SPLINE_CURVE(2,(#78505,#78506,#78507),.UNSPECIFIED.,.F.,.F.)
B_SPLINE_CURVE_WITH_KNOTS((3,3),(0.,0.09156830116281),.UNSPECIFIED.)
CURVE()
GEOMETRIC_REPRESENTATION_ITEM()
RATIONAL_B_SPLINE_CURVE((1.,1.00004989701499,1.00004421979647))
REPRESENTATION_ITEM('')
);
#19348=(
BOUNDED_CURVE()
B_SPLINE_CURVE(2,(#78512,#78513,#78514),.UNSPECIFIED.,.F.,.F.)
B_SPLINE_CURVE_WITH_KNOTS((3,3),(0.0728598735675412,0.164428174992088),
 .UNSPECIFIED.)
CURVE()
GEOMETRIC_REPRESENTATION_ITEM()
RATIONAL_B_SPLINE_CURVE((1.00004422027197,1.00004989755171,1.))
REPRESENTATION_ITEM('')
);
#19349=(
BOUNDED_CURVE()
B_SPLINE_CURVE(2,(#78516,#78517,#78518),.UNSPECIFIED.,.F.,.F.)
B_SPLINE_CURVE_WITH_KNOTS((3,3),(0.526544758504315,0.808610241550327),
 .UNSPECIFIED.)
CURVE()
GEOMETRIC_REPRESENTATION_ITEM()
RATIONAL_B_SPLINE_CURVE((1.00594694470059,1.0065025792733,1.00594694470059))
REPRESENTATION_ITEM('')
);
#19350=(
BOUNDED_CURVE()
B_SPLINE_CURVE(2,(#78520,#78521,#78522),.UNSPECIFIED.,.F.,.F.)
B_SPLINE_CURVE_WITH_KNOTS((3,3),(0.,0.0915683022545724),.UNSPECIFIED.)
CURVE()
GEOMETRIC_REPRESENTATION_ITEM()
RATIONAL_B_SPLINE_CURVE((1.,1.00004989734545,1.00004422008868))
REPRESENTATION_ITEM('')
);
#19351=(
BOUNDED_CURVE()
B_SPLINE_CURVE(2,(#78527,#78528,#78529),.UNSPECIFIED.,.F.,.F.)
B_SPLINE_CURVE_WITH_KNOTS((3,3),(0.0728598733693843,0.164428174992087),
 .UNSPECIFIED.)
CURVE()
GEOMETRIC_REPRESENTATION_ITEM()
RATIONAL_B_SPLINE_CURVE((1.0000442202851,1.00004989756666,1.))
REPRESENTATION_ITEM('')
);
#19352=(
BOUNDED_CURVE()
B_SPLINE_CURVE(2,(#78531,#78532,#78533),.UNSPECIFIED.,.F.,.F.)
B_SPLINE_CURVE_WITH_KNOTS((3,3),(0.526544758504307,0.808610241550322),
 .UNSPECIFIED.)
CURVE()
GEOMETRIC_REPRESENTATION_ITEM()
RATIONAL_B_SPLINE_CURVE((1.00594694470059,1.00650257927331,1.00594694470059))
REPRESENTATION_ITEM('')
);
#19353=(
BOUNDED_CURVE()
B_SPLINE_CURVE(2,(#78535,#78536,#78537),.UNSPECIFIED.,.F.,.F.)
B_SPLINE_CURVE_WITH_KNOTS((3,3),(0.,0.091568301844154),.UNSPECIFIED.)
CURVE()
GEOMETRIC_REPRESENTATION_ITEM()
RATIONAL_B_SPLINE_CURVE((1.,1.00004989738211,1.00004422012141))
REPRESENTATION_ITEM('')
);
#19354=(
BOUNDED_CURVE()
B_SPLINE_CURVE(2,(#78542,#78543,#78544),.UNSPECIFIED.,.F.,.F.)
B_SPLINE_CURVE_WITH_KNOTS((3,3),(0.0728598727493186,0.164428174992087),
 .UNSPECIFIED.)
CURVE()
GEOMETRIC_REPRESENTATION_ITEM()
RATIONAL_B_SPLINE_CURVE((1.00004422024106,1.00004989751739,1.))
REPRESENTATION_ITEM('')
);
#19355=(
BOUNDED_CURVE()
B_SPLINE_CURVE(2,(#78546,#78547,#78548),.UNSPECIFIED.,.F.,.F.)
B_SPLINE_CURVE_WITH_KNOTS((3,3),(0.526544758504317,0.808610241550328),
 .UNSPECIFIED.)
CURVE()
GEOMETRIC_REPRESENTATION_ITEM()
RATIONAL_B_SPLINE_CURVE((1.00594694470058,1.0065025792733,1.00594694470058))
REPRESENTATION_ITEM('')
);
#19356=(
BOUNDED_CURVE()
B_SPLINE_CURVE(2,(#78550,#78551,#78552),.UNSPECIFIED.,.F.,.F.)
B_SPLINE_CURVE_WITH_KNOTS((3,3),(0.,0.0915683005636383),.UNSPECIFIED.)
CURVE()
GEOMETRIC_REPRESENTATION_ITEM()
RATIONAL_B_SPLINE_CURVE((1.,1.00004989687733,1.00004421967485))
REPRESENTATION_ITEM('')
);
#19357=(
BOUNDED_CURVE()
B_SPLINE_CURVE(2,(#78557,#78558,#78559),.UNSPECIFIED.,.F.,.F.)
B_SPLINE_CURVE_WITH_KNOTS((3,3),(0.0728598739393654,0.164428174992088),
 .UNSPECIFIED.)
CURVE()
GEOMETRIC_REPRESENTATION_ITEM()
RATIONAL_B_SPLINE_CURVE((1.00004421961259,1.00004989680742,1.))
REPRESENTATION_ITEM('')
);
#19358=(
BOUNDED_CURVE()
B_SPLINE_CURVE(2,(#78561,#78562,#78563),.UNSPECIFIED.,.F.,.F.)
B_SPLINE_CURVE_WITH_KNOTS((3,3),(0.526544758504316,0.808610241550329),
 .UNSPECIFIED.)
CURVE()
GEOMETRIC_REPRESENTATION_ITEM()
RATIONAL_B_SPLINE_CURVE((1.00594694470059,1.0065025792733,1.00594694470059))
REPRESENTATION_ITEM('')
);
#19359=(
BOUNDED_CURVE()
B_SPLINE_CURVE(2,(#78565,#78566,#78567),.UNSPECIFIED.,.F.,.F.)
B_SPLINE_CURVE_WITH_KNOTS((3,3),(0.,0.0915683013365669),.UNSPECIFIED.)
CURVE()
GEOMETRIC_REPRESENTATION_ITEM()
RATIONAL_B_SPLINE_CURVE((1.,1.00004989717223,1.00004421993572))
REPRESENTATION_ITEM('')
);
#19360=(
BOUNDED_CURVE()
B_SPLINE_CURVE(2,(#78572,#78573,#78574),.UNSPECIFIED.,.F.,.F.)
B_SPLINE_CURVE_WITH_KNOTS((3,3),(0.0728598751585041,0.164428174992087),
 .UNSPECIFIED.)
CURVE()
GEOMETRIC_REPRESENTATION_ITEM()
RATIONAL_B_SPLINE_CURVE((1.00004421967368,1.00004989687551,1.))
REPRESENTATION_ITEM('')
);
#19361=(
BOUNDED_CURVE()
B_SPLINE_CURVE(2,(#78576,#78577,#78578),.UNSPECIFIED.,.F.,.F.)
B_SPLINE_CURVE_WITH_KNOTS((3,3),(0.526544758504317,0.808610241550327),
 .UNSPECIFIED.)
CURVE()
GEOMETRIC_REPRESENTATION_ITEM()
RATIONAL_B_SPLINE_CURVE((1.00594694470058,1.00650257927329,1.00594694470058))
REPRESENTATION_ITEM('')
);
#19362=(
BOUNDED_CURVE()
B_SPLINE_CURVE(2,(#78580,#78581,#78582),.UNSPECIFIED.,.F.,.F.)
B_SPLINE_CURVE_WITH_KNOTS((3,3),(0.,0.0915683017593413),.UNSPECIFIED.)
CURVE()
GEOMETRIC_REPRESENTATION_ITEM()
RATIONAL_B_SPLINE_CURVE((1.,1.00004989738203,1.00004422012139))
REPRESENTATION_ITEM('')
);
#19363=(
BOUNDED_CURVE()
B_SPLINE_CURVE(2,(#78587,#78588,#78589),.UNSPECIFIED.,.F.,.F.)
B_SPLINE_CURVE_WITH_KNOTS((3,3),(0.0728598743955349,0.164428174992088),
 .UNSPECIFIED.)
CURVE()
GEOMETRIC_REPRESENTATION_ITEM()
RATIONAL_B_SPLINE_CURVE((1.00004422007075,1.00004989732408,1.))
REPRESENTATION_ITEM('')
);
#19364=(
BOUNDED_CURVE()
B_SPLINE_CURVE(2,(#78591,#78592,#78593),.UNSPECIFIED.,.F.,.F.)
B_SPLINE_CURVE_WITH_KNOTS((3,3),(0.526544758504317,0.808610241550327),
 .UNSPECIFIED.)
CURVE()
GEOMETRIC_REPRESENTATION_ITEM()
RATIONAL_B_SPLINE_CURVE((1.00594694470058,1.00650257927329,1.00594694470058))
REPRESENTATION_ITEM('')
);
#19365=(
BOUNDED_CURVE()
B_SPLINE_CURVE(2,(#78595,#78596,#78597),.UNSPECIFIED.,.F.,.F.)
B_SPLINE_CURVE_WITH_KNOTS((3,3),(0.,0.0915683011593544),.UNSPECIFIED.)
CURVE()
GEOMETRIC_REPRESENTATION_ITEM()
RATIONAL_B_SPLINE_CURVE((1.,1.00004989717994,1.00004421994266))
REPRESENTATION_ITEM('')
);
#19366=(
BOUNDED_CURVE()
B_SPLINE_CURVE(2,(#78602,#78603,#78604),.UNSPECIFIED.,.F.,.F.)
B_SPLINE_CURVE_WITH_KNOTS((3,3),(0.0728598745472918,0.164428174992087),
 .UNSPECIFIED.)
CURVE()
GEOMETRIC_REPRESENTATION_ITEM()
RATIONAL_B_SPLINE_CURVE((1.00004422005424,1.00004989730536,1.))
REPRESENTATION_ITEM('')
);
#19367=(
BOUNDED_CURVE()
B_SPLINE_CURVE(2,(#78606,#78607,#78608),.UNSPECIFIED.,.F.,.F.)
B_SPLINE_CURVE_WITH_KNOTS((3,3),(0.526544758504319,0.808610241550335),
 .UNSPECIFIED.)
CURVE()
GEOMETRIC_REPRESENTATION_ITEM()
RATIONAL_B_SPLINE_CURVE((1.0059469447006,1.00650257927331,1.0059469447006))
REPRESENTATION_ITEM('')
);
#19368=(
BOUNDED_CURVE()
B_SPLINE_CURVE(2,(#78610,#78611,#78612),.UNSPECIFIED.,.F.,.F.)
B_SPLINE_CURVE_WITH_KNOTS((3,3),(0.,0.0915683006206516),.UNSPECIFIED.)
CURVE()
GEOMETRIC_REPRESENTATION_ITEM()
RATIONAL_B_SPLINE_CURVE((1.,1.00004989694253,1.00004421973259))
REPRESENTATION_ITEM('')
);
#19369=(
BOUNDED_CURVE()
B_SPLINE_CURVE(2,(#78617,#78618,#78619),.UNSPECIFIED.,.F.,.F.)
B_SPLINE_CURVE_WITH_KNOTS((3,3),(0.0728598732187887,0.164428174992087),
 .UNSPECIFIED.)
CURVE()
GEOMETRIC_REPRESENTATION_ITEM()
RATIONAL_B_SPLINE_CURVE((1.00004422023233,1.00004989750722,1.))
REPRESENTATION_ITEM('')
);
#19370=(
BOUNDED_CURVE()
B_SPLINE_CURVE(2,(#78621,#78622,#78623),.UNSPECIFIED.,.F.,.F.)
B_SPLINE_CURVE_WITH_KNOTS((3,3),(0.526544758504317,0.808610241550327),
 .UNSPECIFIED.)
CURVE()
GEOMETRIC_REPRESENTATION_ITEM()
RATIONAL_B_SPLINE_CURVE((1.00594694470058,1.00650257927329,1.00594694470058))
REPRESENTATION_ITEM('')
);
#19371=(
BOUNDED_CURVE()
B_SPLINE_CURVE(2,(#78625,#78626,#78627),.UNSPECIFIED.,.F.,.F.)
B_SPLINE_CURVE_WITH_KNOTS((3,3),(0.,0.0915683011622659),.UNSPECIFIED.)
CURVE()
GEOMETRIC_REPRESENTATION_ITEM()
RATIONAL_B_SPLINE_CURVE((1.,1.00004989751462,1.00004422023926))
REPRESENTATION_ITEM('')
);
#19372=(
BOUNDED_CURVE()
B_SPLINE_CURVE(2,(#78632,#78633,#78634),.UNSPECIFIED.,.F.,.F.)
B_SPLINE_CURVE_WITH_KNOTS((3,3),(0.0728598743613769,0.164428174992088),
 .UNSPECIFIED.)
CURVE()
GEOMETRIC_REPRESENTATION_ITEM()
RATIONAL_B_SPLINE_CURVE((1.00004421988312,1.0000498971124,1.))
REPRESENTATION_ITEM('')
);
#19373=(
BOUNDED_CURVE()
B_SPLINE_CURVE(2,(#78636,#78637,#78638),.UNSPECIFIED.,.F.,.F.)
B_SPLINE_CURVE_WITH_KNOTS((3,3),(0.526544758504314,0.808610241550329),
 .UNSPECIFIED.)
CURVE()
GEOMETRIC_REPRESENTATION_ITEM()
RATIONAL_B_SPLINE_CURVE((1.00594694470059,1.00650257927331,1.00594694470059))
REPRESENTATION_ITEM('')
);
#19374=(
BOUNDED_CURVE()
B_SPLINE_CURVE(2,(#78640,#78641,#78642),.UNSPECIFIED.,.F.,.F.)
B_SPLINE_CURVE_WITH_KNOTS((3,3),(0.,0.0915683004683977),.UNSPECIFIED.)
CURVE()
GEOMETRIC_REPRESENTATION_ITEM()
RATIONAL_B_SPLINE_CURVE((1.,1.00004989675431,1.00004421956588))
REPRESENTATION_ITEM('')
);
#19375=(
BOUNDED_CURVE()
B_SPLINE_CURVE(2,(#78647,#78648,#78649),.UNSPECIFIED.,.F.,.F.)
B_SPLINE_CURVE_WITH_KNOTS((3,3),(0.0728598726718109,0.164428174992088),
 .UNSPECIFIED.)
CURVE()
GEOMETRIC_REPRESENTATION_ITEM()
RATIONAL_B_SPLINE_CURVE((1.00004422040501,1.00004989770244,1.))
REPRESENTATION_ITEM('')
);
#19376=(
BOUNDED_CURVE()
B_SPLINE_CURVE(2,(#78651,#78652,#78653),.UNSPECIFIED.,.F.,.F.)
B_SPLINE_CURVE_WITH_KNOTS((3,3),(0.526544758504306,0.808610241550323),
 .UNSPECIFIED.)
CURVE()
GEOMETRIC_REPRESENTATION_ITEM()
RATIONAL_B_SPLINE_CURVE((1.0059469447006,1.00650257927332,1.0059469447006))
REPRESENTATION_ITEM('')
);
#19377=(
BOUNDED_CURVE()
B_SPLINE_CURVE(2,(#78655,#78656,#78657),.UNSPECIFIED.,.F.,.F.)
B_SPLINE_CURVE_WITH_KNOTS((3,3),(0.,0.0915683018343069),.UNSPECIFIED.)
CURVE()
GEOMETRIC_REPRESENTATION_ITEM()
RATIONAL_B_SPLINE_CURVE((1.,1.00004989767869,1.00004422038426))
REPRESENTATION_ITEM('')
);
#19378=(
BOUNDED_CURVE()
B_SPLINE_CURVE(2,(#78662,#78663,#78664),.UNSPECIFIED.,.F.,.F.)
B_SPLINE_CURVE_WITH_KNOTS((3,3),(0.0728598734298788,0.164428174992087),
 .UNSPECIFIED.)
CURVE()
GEOMETRIC_REPRESENTATION_ITEM()
RATIONAL_B_SPLINE_CURVE((1.00004422015244,1.00004989741692,1.))
REPRESENTATION_ITEM('')
);
#19379=(
BOUNDED_CURVE()
B_SPLINE_CURVE(2,(#78666,#78667,#78668),.UNSPECIFIED.,.F.,.F.)
B_SPLINE_CURVE_WITH_KNOTS((3,3),(0.526544758504322,0.808610241550332),
 .UNSPECIFIED.)
CURVE()
GEOMETRIC_REPRESENTATION_ITEM()
RATIONAL_B_SPLINE_CURVE((1.00594694470058,1.00650257927329,1.00594694470058))
REPRESENTATION_ITEM('')
);
#19380=(
BOUNDED_CURVE()
B_SPLINE_CURVE(2,(#78670,#78671,#78672),.UNSPECIFIED.,.F.,.F.)
B_SPLINE_CURVE_WITH_KNOTS((3,3),(0.,0.0915683005750663),.UNSPECIFIED.)
CURVE()
GEOMETRIC_REPRESENTATION_ITEM()
RATIONAL_B_SPLINE_CURVE((1.,1.0000498970517,1.00004421982937))
REPRESENTATION_ITEM('')
);
#19381=(
BOUNDED_CURVE()
B_SPLINE_CURVE(2,(#78677,#78678,#78679),.UNSPECIFIED.,.F.,.F.)
B_SPLINE_CURVE_WITH_KNOTS((3,3),(0.0728598737528459,0.164428174992088),
 .UNSPECIFIED.)
CURVE()
GEOMETRIC_REPRESENTATION_ITEM()
RATIONAL_B_SPLINE_CURVE((1.00004421990677,1.0000498971395,1.))
REPRESENTATION_ITEM('')
);
#19382=(
BOUNDED_CURVE()
B_SPLINE_CURVE(2,(#78681,#78682,#78683),.UNSPECIFIED.,.F.,.F.)
B_SPLINE_CURVE_WITH_KNOTS((3,3),(0.526544758504314,0.808610241550329),
 .UNSPECIFIED.)
CURVE()
GEOMETRIC_REPRESENTATION_ITEM()
RATIONAL_B_SPLINE_CURVE((1.00594694470059,1.00650257927331,1.00594694470059))
REPRESENTATION_ITEM('')
);
#19383=(
BOUNDED_CURVE()
B_SPLINE_CURVE(2,(#78685,#78686,#78687),.UNSPECIFIED.,.F.,.F.)
B_SPLINE_CURVE_WITH_KNOTS((3,3),(0.,0.0915683018875454),.UNSPECIFIED.)
CURVE()
GEOMETRIC_REPRESENTATION_ITEM()
RATIONAL_B_SPLINE_CURVE((1.,1.00004989719222,1.0000442199531))
REPRESENTATION_ITEM('')
);
#19384=(
BOUNDED_CURVE()
B_SPLINE_CURVE(2,(#78692,#78693,#78694),.UNSPECIFIED.,.F.,.F.)
B_SPLINE_CURVE_WITH_KNOTS((3,3),(0.0728598745151923,0.164428174992087),
 .UNSPECIFIED.)
CURVE()
GEOMETRIC_REPRESENTATION_ITEM()
RATIONAL_B_SPLINE_CURVE((1.00004421966589,1.00004989686717,1.))
REPRESENTATION_ITEM('')
);
#19385=(
BOUNDED_CURVE()
B_SPLINE_CURVE(2,(#78696,#78697,#78698),.UNSPECIFIED.,.F.,.F.)
B_SPLINE_CURVE_WITH_KNOTS((3,3),(0.526544758504313,0.808610241550331),
 .UNSPECIFIED.)
CURVE()
GEOMETRIC_REPRESENTATION_ITEM()
RATIONAL_B_SPLINE_CURVE((1.0059469447006,1.00650257927332,1.0059469447006))
REPRESENTATION_ITEM('')
);
#19386=(
BOUNDED_CURVE()
B_SPLINE_CURVE(2,(#78700,#78701,#78702),.UNSPECIFIED.,.F.,.F.)
B_SPLINE_CURVE_WITH_KNOTS((3,3),(0.,0.0915683010779811),.UNSPECIFIED.)
CURVE()
GEOMETRIC_REPRESENTATION_ITEM()
RATIONAL_B_SPLINE_CURVE((1.,1.00004989711025,1.00004421988095))
REPRESENTATION_ITEM('')
);
#19387=(
BOUNDED_CURVE()
B_SPLINE_CURVE(2,(#78707,#78708,#78709),.UNSPECIFIED.,.F.,.F.)
B_SPLINE_CURVE_WITH_KNOTS((3,3),(0.0728598743365227,0.164428174992087),
 .UNSPECIFIED.)
CURVE()
GEOMETRIC_REPRESENTATION_ITEM()
RATIONAL_B_SPLINE_CURVE((1.00004422013591,1.00004989739766,1.))
REPRESENTATION_ITEM('')
);
#19388=(
BOUNDED_CURVE()
B_SPLINE_CURVE(2,(#78711,#78712,#78713),.UNSPECIFIED.,.F.,.F.)
B_SPLINE_CURVE_WITH_KNOTS((3,3),(0.526544758504318,0.808610241550326),
 .UNSPECIFIED.)
CURVE()
GEOMETRIC_REPRESENTATION_ITEM()
RATIONAL_B_SPLINE_CURVE((1.00594694470057,1.00650257927328,1.00594694470057))
REPRESENTATION_ITEM('')
);
#19389=(
BOUNDED_CURVE()
B_SPLINE_CURVE(2,(#78715,#78716,#78717),.UNSPECIFIED.,.F.,.F.)
B_SPLINE_CURVE_WITH_KNOTS((3,3),(0.,0.0915682998237193),.UNSPECIFIED.)
CURVE()
GEOMETRIC_REPRESENTATION_ITEM()
RATIONAL_B_SPLINE_CURVE((1.,1.00004989671321,1.00004421952985))
REPRESENTATION_ITEM('')
);
#19390=(
BOUNDED_CURVE()
B_SPLINE_CURVE(2,(#78722,#78723,#78724),.UNSPECIFIED.,.F.,.F.)
B_SPLINE_CURVE_WITH_KNOTS((3,3),(0.0728598745249184,0.164428174992087),
 .UNSPECIFIED.)
CURVE()
GEOMETRIC_REPRESENTATION_ITEM()
RATIONAL_B_SPLINE_CURVE((1.00004421993429,1.00004989717003,1.))
REPRESENTATION_ITEM('')
);
#19391=(
BOUNDED_CURVE()
B_SPLINE_CURVE(2,(#78726,#78727,#78728),.UNSPECIFIED.,.F.,.F.)
B_SPLINE_CURVE_WITH_KNOTS((3,3),(0.52654475850432,0.808610241550335),
 .UNSPECIFIED.)
CURVE()
GEOMETRIC_REPRESENTATION_ITEM()
RATIONAL_B_SPLINE_CURVE((1.0059469447006,1.00650257927331,1.0059469447006))
REPRESENTATION_ITEM('')
);
#19392=(
BOUNDED_CURVE()
B_SPLINE_CURVE(2,(#78730,#78731,#78732),.UNSPECIFIED.,.F.,.F.)
B_SPLINE_CURVE_WITH_KNOTS((3,3),(0.,0.0915683006102755),.UNSPECIFIED.)
CURVE()
GEOMETRIC_REPRESENTATION_ITEM()
RATIONAL_B_SPLINE_CURVE((1.,1.000049897179,1.00004421994216))
REPRESENTATION_ITEM('')
);
#19393=(
BOUNDED_CURVE()
B_SPLINE_CURVE(2,(#78737,#78738,#78739),.UNSPECIFIED.,.F.,.F.)
B_SPLINE_CURVE_WITH_KNOTS((3,3),(0.0728598745442839,0.164428174992087),
 .UNSPECIFIED.)
CURVE()
GEOMETRIC_REPRESENTATION_ITEM()
RATIONAL_B_SPLINE_CURVE((1.0000442198851,1.00004989711451,1.))
REPRESENTATION_ITEM('')
);
#19394=(
BOUNDED_CURVE()
B_SPLINE_CURVE(2,(#78741,#78742,#78743),.UNSPECIFIED.,.F.,.F.)
B_SPLINE_CURVE_WITH_KNOTS((3,3),(0.526544758504317,0.808610241550327),
 .UNSPECIFIED.)
CURVE()
GEOMETRIC_REPRESENTATION_ITEM()
RATIONAL_B_SPLINE_CURVE((1.00594694470058,1.00650257927329,1.00594694470058))
REPRESENTATION_ITEM('')
);
#19395=(
BOUNDED_CURVE()
B_SPLINE_CURVE(2,(#78745,#78746,#78747),.UNSPECIFIED.,.F.,.F.)
B_SPLINE_CURVE_WITH_KNOTS((3,3),(0.,0.0915683018203568),.UNSPECIFIED.)
CURVE()
GEOMETRIC_REPRESENTATION_ITEM()
RATIONAL_B_SPLINE_CURVE((1.,1.00004989789332,1.00004422057448))
REPRESENTATION_ITEM('')
);
#19396=(
BOUNDED_CURVE()
B_SPLINE_CURVE(2,(#78752,#78753,#78754),.UNSPECIFIED.,.F.,.F.)
B_SPLINE_CURVE_WITH_KNOTS((3,3),(0.0728598737856223,0.164428174992088),
 .UNSPECIFIED.)
CURVE()
GEOMETRIC_REPRESENTATION_ITEM()
RATIONAL_B_SPLINE_CURVE((1.00004421995822,1.00004989719753,1.))
REPRESENTATION_ITEM('')
);
#19397=(
BOUNDED_CURVE()
B_SPLINE_CURVE(2,(#78756,#78757,#78758),.UNSPECIFIED.,.F.,.F.)
B_SPLINE_CURVE_WITH_KNOTS((3,3),(0.52654475850432,0.808610241550332),
 .UNSPECIFIED.)
CURVE()
GEOMETRIC_REPRESENTATION_ITEM()
RATIONAL_B_SPLINE_CURVE((1.00594694470059,1.0065025792733,1.00594694470059))
REPRESENTATION_ITEM('')
);
#19398=(
BOUNDED_CURVE()
B_SPLINE_CURVE(2,(#78760,#78761,#78762),.UNSPECIFIED.,.F.,.F.)
B_SPLINE_CURVE_WITH_KNOTS((3,3),(0.,0.0915683018433535),.UNSPECIFIED.)
CURVE()
GEOMETRIC_REPRESENTATION_ITEM()
RATIONAL_B_SPLINE_CURVE((1.,1.00004989711595,1.00004421988554))
REPRESENTATION_ITEM('')
);
#19399=(
BOUNDED_CURVE()
B_SPLINE_CURVE(2,(#78767,#78768,#78769),.UNSPECIFIED.,.F.,.F.)
B_SPLINE_CURVE_WITH_KNOTS((3,3),(0.0728598735563218,0.164428174992087),
 .UNSPECIFIED.)
CURVE()
GEOMETRIC_REPRESENTATION_ITEM()
RATIONAL_B_SPLINE_CURVE((1.00004422001458,1.00004989726128,1.))
REPRESENTATION_ITEM('')
);
#19400=(
BOUNDED_CURVE()
B_SPLINE_CURVE(2,(#78771,#78772,#78773),.UNSPECIFIED.,.F.,.F.)
B_SPLINE_CURVE_WITH_KNOTS((3,3),(0.526544758504322,0.808610241550332),
 .UNSPECIFIED.)
CURVE()
GEOMETRIC_REPRESENTATION_ITEM()
RATIONAL_B_SPLINE_CURVE((1.00594694470058,1.00650257927329,1.00594694470058))
REPRESENTATION_ITEM('')
);
#19401=(
BOUNDED_CURVE()
B_SPLINE_CURVE(2,(#78775,#78776,#78777),.UNSPECIFIED.,.F.,.F.)
B_SPLINE_CURVE_WITH_KNOTS((3,3),(0.,0.0915682994549458),.UNSPECIFIED.)
CURVE()
GEOMETRIC_REPRESENTATION_ITEM()
RATIONAL_B_SPLINE_CURVE((1.,1.00004989645929,1.00004421930504))
REPRESENTATION_ITEM('')
);
#19402=(
BOUNDED_CURVE()
B_SPLINE_CURVE(2,(#78782,#78783,#78784),.UNSPECIFIED.,.F.,.F.)
B_SPLINE_CURVE_WITH_KNOTS((3,3),(0.0728598733693843,0.164428174992087),
 .UNSPECIFIED.)
CURVE()
GEOMETRIC_REPRESENTATION_ITEM()
RATIONAL_B_SPLINE_CURVE((1.0000442202851,1.00004989756666,1.))
REPRESENTATION_ITEM('')
);
#19403=(
BOUNDED_CURVE()
B_SPLINE_CURVE(2,(#78786,#78787,#78788),.UNSPECIFIED.,.F.,.F.)
B_SPLINE_CURVE_WITH_KNOTS((3,3),(0.526544758504307,0.808610241550322),
 .UNSPECIFIED.)
CURVE()
GEOMETRIC_REPRESENTATION_ITEM()
RATIONAL_B_SPLINE_CURVE((1.00594694470059,1.00650257927331,1.00594694470059))
REPRESENTATION_ITEM('')
);
#19404=(
BOUNDED_CURVE()
B_SPLINE_CURVE(2,(#78790,#78791,#78792),.UNSPECIFIED.,.F.,.F.)
B_SPLINE_CURVE_WITH_KNOTS((3,3),(0.,0.091568301844154),.UNSPECIFIED.)
CURVE()
GEOMETRIC_REPRESENTATION_ITEM()
RATIONAL_B_SPLINE_CURVE((1.,1.00004989738211,1.00004422012141))
REPRESENTATION_ITEM('')
);
#19405=(
BOUNDED_CURVE()
B_SPLINE_CURVE(2,(#78797,#78798,#78799),.UNSPECIFIED.,.F.,.F.)
B_SPLINE_CURVE_WITH_KNOTS((3,3),(0.0728598732916255,0.164428174992087),
 .UNSPECIFIED.)
CURVE()
GEOMETRIC_REPRESENTATION_ITEM()
RATIONAL_B_SPLINE_CURVE((1.00004422000312,1.00004989724853,1.))
REPRESENTATION_ITEM('')
);
#19406=(
BOUNDED_CURVE()
B_SPLINE_CURVE(2,(#78801,#78802,#78803),.UNSPECIFIED.,.F.,.F.)
B_SPLINE_CURVE_WITH_KNOTS((3,3),(0.526544758504322,0.808610241550332),
 .UNSPECIFIED.)
CURVE()
GEOMETRIC_REPRESENTATION_ITEM()
RATIONAL_B_SPLINE_CURVE((1.00594694470058,1.00650257927329,1.00594694470058))
REPRESENTATION_ITEM('')
);
#19407=(
BOUNDED_CURVE()
B_SPLINE_CURVE(2,(#78805,#78806,#78807),.UNSPECIFIED.,.F.,.F.)
B_SPLINE_CURVE_WITH_KNOTS((3,3),(0.,0.0915683005619487),.UNSPECIFIED.)
CURVE()
GEOMETRIC_REPRESENTATION_ITEM()
RATIONAL_B_SPLINE_CURVE((1.,1.00004989697534,1.0000442197617))
REPRESENTATION_ITEM('')
);
#19408=(
BOUNDED_CURVE()
B_SPLINE_CURVE(2,(#78812,#78813,#78814),.UNSPECIFIED.,.F.,.F.)
B_SPLINE_CURVE_WITH_KNOTS((3,3),(0.0728598731686667,0.164428174992087),
 .UNSPECIFIED.)
CURVE()
GEOMETRIC_REPRESENTATION_ITEM()
RATIONAL_B_SPLINE_CURVE((1.00004421982523,1.00004989704789,1.))
REPRESENTATION_ITEM('')
);
#19409=(
BOUNDED_CURVE()
B_SPLINE_CURVE(2,(#78816,#78817,#78818),.UNSPECIFIED.,.F.,.F.)
B_SPLINE_CURVE_WITH_KNOTS((3,3),(0.526544758504316,0.808610241550328),
 .UNSPECIFIED.)
CURVE()
GEOMETRIC_REPRESENTATION_ITEM()
RATIONAL_B_SPLINE_CURVE((1.00594694470059,1.0065025792733,1.00594694470059))
REPRESENTATION_ITEM('')
);
#19410=(
BOUNDED_CURVE()
B_SPLINE_CURVE(2,(#78820,#78821,#78822),.UNSPECIFIED.,.F.,.F.)
B_SPLINE_CURVE_WITH_KNOTS((3,3),(0.,0.0915683024294117),.UNSPECIFIED.)
CURVE()
GEOMETRIC_REPRESENTATION_ITEM()
RATIONAL_B_SPLINE_CURVE((1.,1.00004989771985,1.00004422042037))
REPRESENTATION_ITEM('')
);
#19411=(
BOUNDED_CURVE()
B_SPLINE_CURVE(2,(#78827,#78828,#78829),.UNSPECIFIED.,.F.,.F.)
B_SPLINE_CURVE_WITH_KNOTS((3,3),(0.0728598730627314,0.164428174992087),
 .UNSPECIFIED.)
CURVE()
GEOMETRIC_REPRESENTATION_ITEM()
RATIONAL_B_SPLINE_CURVE((1.00004422011343,1.00004989737316,1.))
REPRESENTATION_ITEM('')
);
#19412=(
BOUNDED_CURVE()
B_SPLINE_CURVE(2,(#78831,#78832,#78833),.UNSPECIFIED.,.F.,.F.)
B_SPLINE_CURVE_WITH_KNOTS((3,3),(0.526544758504317,0.808610241550327),
 .UNSPECIFIED.)
CURVE()
GEOMETRIC_REPRESENTATION_ITEM()
RATIONAL_B_SPLINE_CURVE((1.00594694470058,1.00650257927329,1.00594694470058))
REPRESENTATION_ITEM('')
);
#19413=(
BOUNDED_CURVE()
B_SPLINE_CURVE(2,(#78835,#78836,#78837),.UNSPECIFIED.,.F.,.F.)
B_SPLINE_CURVE_WITH_KNOTS((3,3),(0.,0.0915683011593819),.UNSPECIFIED.)
CURVE()
GEOMETRIC_REPRESENTATION_ITEM()
RATIONAL_B_SPLINE_CURVE((1.,1.00004989718316,1.00004421994552))
REPRESENTATION_ITEM('')
);
#19414=(
BOUNDED_CURVE()
B_SPLINE_CURVE(2,(#78842,#78843,#78844),.UNSPECIFIED.,.F.,.F.)
B_SPLINE_CURVE_WITH_KNOTS((3,3),(0.0728598745376772,0.164428174992087),
 .UNSPECIFIED.)
CURVE()
GEOMETRIC_REPRESENTATION_ITEM()
RATIONAL_B_SPLINE_CURVE((1.00004421990789,1.00004989714022,1.))
REPRESENTATION_ITEM('')
);
#19415=(
BOUNDED_CURVE()
B_SPLINE_CURVE(2,(#78846,#78847,#78848),.UNSPECIFIED.,.F.,.F.)
B_SPLINE_CURVE_WITH_KNOTS((3,3),(0.526544758504319,0.808610241550335),
 .UNSPECIFIED.)
CURVE()
GEOMETRIC_REPRESENTATION_ITEM()
RATIONAL_B_SPLINE_CURVE((1.0059469447006,1.00650257927331,1.0059469447006))
REPRESENTATION_ITEM('')
);
#19416=(
BOUNDED_CURVE()
B_SPLINE_CURVE(2,(#78850,#78851,#78852),.UNSPECIFIED.,.F.,.F.)
B_SPLINE_CURVE_WITH_KNOTS((3,3),(0.,0.0915683006214894),.UNSPECIFIED.)
CURVE()
GEOMETRIC_REPRESENTATION_ITEM()
RATIONAL_B_SPLINE_CURVE((1.,1.00004989740271,1.00004422014041))
REPRESENTATION_ITEM('')
);
#19417=(
BOUNDED_CURVE()
B_SPLINE_CURVE(2,(#78857,#78858,#78859),.UNSPECIFIED.,.F.,.F.)
B_SPLINE_CURVE_WITH_KNOTS((3,3),(0.0728598745473656,0.164428174992088),
 .UNSPECIFIED.)
CURVE()
GEOMETRIC_REPRESENTATION_ITEM()
RATIONAL_B_SPLINE_CURVE((1.00004421990015,1.00004989713148,1.))
REPRESENTATION_ITEM('')
);
#19418=(
BOUNDED_CURVE()
B_SPLINE_CURVE(2,(#78861,#78862,#78863),.UNSPECIFIED.,.F.,.F.)
B_SPLINE_CURVE_WITH_KNOTS((3,3),(0.526544758504317,0.808610241550327),
 .UNSPECIFIED.)
CURVE()
GEOMETRIC_REPRESENTATION_ITEM()
RATIONAL_B_SPLINE_CURVE((1.00594694470058,1.00650257927329,1.00594694470058))
REPRESENTATION_ITEM('')
);
#19419=(
BOUNDED_CURVE()
B_SPLINE_CURVE(2,(#78865,#78866,#78867),.UNSPECIFIED.,.F.,.F.)
B_SPLINE_CURVE_WITH_KNOTS((3,3),(0.,0.0915683004967461),.UNSPECIFIED.)
CURVE()
GEOMETRIC_REPRESENTATION_ITEM()
RATIONAL_B_SPLINE_CURVE((1.,1.00004989676149,1.00004421957222))
REPRESENTATION_ITEM('')
);
#19420=(
BOUNDED_CURVE()
B_SPLINE_CURVE(2,(#78872,#78873,#78874),.UNSPECIFIED.,.F.,.F.)
B_SPLINE_CURVE_WITH_KNOTS((3,3),(0.0728598736647092,0.164428174992087),
 .UNSPECIFIED.)
CURVE()
GEOMETRIC_REPRESENTATION_ITEM()
RATIONAL_B_SPLINE_CURVE((1.00004422012316,1.00004989738373,1.))
REPRESENTATION_ITEM('')
);
#19421=(
BOUNDED_CURVE()
B_SPLINE_CURVE(2,(#78876,#78877,#78878),.UNSPECIFIED.,.F.,.F.)
B_SPLINE_CURVE_WITH_KNOTS((3,3),(0.526544758504317,0.808610241550327),
 .UNSPECIFIED.)
CURVE()
GEOMETRIC_REPRESENTATION_ITEM()
RATIONAL_B_SPLINE_CURVE((1.00594694470058,1.00650257927329,1.00594694470058))
REPRESENTATION_ITEM('')
);
#19422=(
BOUNDED_CURVE()
B_SPLINE_CURVE(2,(#78880,#78881,#78882),.UNSPECIFIED.,.F.,.F.)
B_SPLINE_CURVE_WITH_KNOTS((3,3),(0.,0.0915683012539948),.UNSPECIFIED.)
CURVE()
GEOMETRIC_REPRESENTATION_ITEM()
RATIONAL_B_SPLINE_CURVE((1.,1.0000498973998,1.00004422013745))
REPRESENTATION_ITEM('')
);
#19423=(
BOUNDED_CURVE()
B_SPLINE_CURVE(2,(#78887,#78888,#78889),.UNSPECIFIED.,.F.,.F.)
B_SPLINE_CURVE_WITH_KNOTS((3,3),(0.0728598742416343,0.164428174992088),
 .UNSPECIFIED.)
CURVE()
GEOMETRIC_REPRESENTATION_ITEM()
RATIONAL_B_SPLINE_CURVE((1.00004421960735,1.0000498968013,1.))
REPRESENTATION_ITEM('')
);
#19424=(
BOUNDED_CURVE()
B_SPLINE_CURVE(2,(#78891,#78892,#78893),.UNSPECIFIED.,.F.,.F.)
B_SPLINE_CURVE_WITH_KNOTS((3,3),(0.526544758504316,0.808610241550327),
 .UNSPECIFIED.)
CURVE()
GEOMETRIC_REPRESENTATION_ITEM()
RATIONAL_B_SPLINE_CURVE((1.00594694470059,1.0065025792733,1.00594694470059))
REPRESENTATION_ITEM('')
);
#19425=(
BOUNDED_CURVE()
B_SPLINE_CURVE(2,(#78895,#78896,#78897),.UNSPECIFIED.,.F.,.F.)
B_SPLINE_CURVE_WITH_KNOTS((3,3),(0.,0.0915683010196277),.UNSPECIFIED.)
CURVE()
GEOMETRIC_REPRESENTATION_ITEM()
RATIONAL_B_SPLINE_CURVE((1.,1.00004989727193,1.00004422002427))
REPRESENTATION_ITEM('')
);
#19426=(
BOUNDED_CURVE()
B_SPLINE_CURVE(2,(#78902,#78903,#78904),.UNSPECIFIED.,.F.,.F.)
B_SPLINE_CURVE_WITH_KNOTS((3,3),(0.0728598731345689,0.164428174992088),
 .UNSPECIFIED.)
CURVE()
GEOMETRIC_REPRESENTATION_ITEM()
RATIONAL_B_SPLINE_CURVE((1.00004422008966,1.00004989734629,1.))
REPRESENTATION_ITEM('')
);
#19427=(
BOUNDED_CURVE()
B_SPLINE_CURVE(2,(#78906,#78907,#78908),.UNSPECIFIED.,.F.,.F.)
B_SPLINE_CURVE_WITH_KNOTS((3,3),(0.526544758504308,0.80861024155032),
 .UNSPECIFIED.)
CURVE()
GEOMETRIC_REPRESENTATION_ITEM()
RATIONAL_B_SPLINE_CURVE((1.00594694470059,1.0065025792733,1.00594694470059))
REPRESENTATION_ITEM('')
);
#19428=(
BOUNDED_CURVE()
B_SPLINE_CURVE(2,(#78910,#78911,#78912),.UNSPECIFIED.,.F.,.F.)
B_SPLINE_CURVE_WITH_KNOTS((3,3),(0.,0.0915683023201614),.UNSPECIFIED.)
CURVE()
GEOMETRIC_REPRESENTATION_ITEM()
RATIONAL_B_SPLINE_CURVE((1.,1.00004989756362,1.00004422028198))
REPRESENTATION_ITEM('')
);
#19429=(
BOUNDED_CURVE()
B_SPLINE_CURVE(2,(#78917,#78918,#78919),.UNSPECIFIED.,.F.,.F.)
B_SPLINE_CURVE_WITH_KNOTS((3,3),(0.0728598741432394,0.164428174992087),
 .UNSPECIFIED.)
CURVE()
GEOMETRIC_REPRESENTATION_ITEM()
RATIONAL_B_SPLINE_CURVE((1.0000442198169,1.00004989703782,1.))
REPRESENTATION_ITEM('')
);
#19430=(
BOUNDED_CURVE()
B_SPLINE_CURVE(2,(#78921,#78922,#78923),.UNSPECIFIED.,.F.,.F.)
B_SPLINE_CURVE_WITH_KNOTS((3,3),(0.526544758504322,0.808610241550331),
 .UNSPECIFIED.)
CURVE()
GEOMETRIC_REPRESENTATION_ITEM()
RATIONAL_B_SPLINE_CURVE((1.00594694470057,1.00650257927328,1.00594694470057))
REPRESENTATION_ITEM('')
);
#19431=(
BOUNDED_CURVE()
B_SPLINE_CURVE(2,(#78925,#78926,#78927),.UNSPECIFIED.,.F.,.F.)
B_SPLINE_CURVE_WITH_KNOTS((3,3),(0.,0.091568300071012),.UNSPECIFIED.)
CURVE()
GEOMETRIC_REPRESENTATION_ITEM()
RATIONAL_B_SPLINE_CURVE((1.,1.00004989671001,1.00004421952686))
REPRESENTATION_ITEM('')
);
#19432=(
BOUNDED_CURVE()
B_SPLINE_CURVE(2,(#78932,#78933,#78934),.UNSPECIFIED.,.F.,.F.)
B_SPLINE_CURVE_WITH_KNOTS((3,3),(0.072859874431626,0.164428174992088),
 .UNSPECIFIED.)
CURVE()
GEOMETRIC_REPRESENTATION_ITEM()
RATIONAL_B_SPLINE_CURVE((1.00004421999585,1.00004989723955,1.))
REPRESENTATION_ITEM('')
);
#19433=(
BOUNDED_CURVE()
B_SPLINE_CURVE(2,(#78936,#78937,#78938),.UNSPECIFIED.,.F.,.F.)
B_SPLINE_CURVE_WITH_KNOTS((3,3),(0.526544758504315,0.80861024155033),
 .UNSPECIFIED.)
CURVE()
GEOMETRIC_REPRESENTATION_ITEM()
RATIONAL_B_SPLINE_CURVE((1.00594694470059,1.00650257927331,1.00594694470059))
REPRESENTATION_ITEM('')
);
#19434=(
BOUNDED_CURVE()
B_SPLINE_CURVE(2,(#78940,#78941,#78942),.UNSPECIFIED.,.F.,.F.)
B_SPLINE_CURVE_WITH_KNOTS((3,3),(0.,0.0915683013824899),.UNSPECIFIED.)
CURVE()
GEOMETRIC_REPRESENTATION_ITEM()
RATIONAL_B_SPLINE_CURVE((1.,1.00004989718276,1.00004421994503))
REPRESENTATION_ITEM('')
);
#19435=(
BOUNDED_CURVE()
B_SPLINE_CURVE(2,(#78947,#78948,#78949),.UNSPECIFIED.,.F.,.F.)
B_SPLINE_CURVE_WITH_KNOTS((3,3),(0.0728598738602229,0.164428174992088),
 .UNSPECIFIED.)
CURVE()
GEOMETRIC_REPRESENTATION_ITEM()
RATIONAL_B_SPLINE_CURVE((1.00004421989654,1.00004989712788,1.))
REPRESENTATION_ITEM('')
);
#19436=(
BOUNDED_CURVE()
B_SPLINE_CURVE(2,(#78951,#78952,#78953),.UNSPECIFIED.,.F.,.F.)
B_SPLINE_CURVE_WITH_KNOTS((3,3),(0.526544758504319,0.808610241550335),
 .UNSPECIFIED.)
CURVE()
GEOMETRIC_REPRESENTATION_ITEM()
RATIONAL_B_SPLINE_CURVE((1.0059469447006,1.00650257927331,1.0059469447006))
REPRESENTATION_ITEM('')
);
#19437=(
BOUNDED_CURVE()
B_SPLINE_CURVE(2,(#78955,#78956,#78957),.UNSPECIFIED.,.F.,.F.)
B_SPLINE_CURVE_WITH_KNOTS((3,3),(0.,0.0915683010770035),.UNSPECIFIED.)
CURVE()
GEOMETRIC_REPRESENTATION_ITEM()
RATIONAL_B_SPLINE_CURVE((1.,1.00004989738745,1.00004422012661))
REPRESENTATION_ITEM('')
);
#19438=(
BOUNDED_CURVE()
B_SPLINE_CURVE(2,(#78962,#78963,#78964),.UNSPECIFIED.,.F.,.F.)
B_SPLINE_CURVE_WITH_KNOTS((3,3),(0.0728598737013136,0.164428174992087),
 .UNSPECIFIED.)
CURVE()
GEOMETRIC_REPRESENTATION_ITEM()
RATIONAL_B_SPLINE_CURVE((1.00004421995655,1.0000498971957,1.))
REPRESENTATION_ITEM('')
);
#19439=(
BOUNDED_CURVE()
B_SPLINE_CURVE(2,(#78966,#78967,#78968),.UNSPECIFIED.,.F.,.F.)
B_SPLINE_CURVE_WITH_KNOTS((3,3),(0.526544758504317,0.808610241550327),
 .UNSPECIFIED.)
CURVE()
GEOMETRIC_REPRESENTATION_ITEM()
RATIONAL_B_SPLINE_CURVE((1.00594694470058,1.00650257927329,1.00594694470058))
REPRESENTATION_ITEM('')
);
#19440=(
BOUNDED_CURVE()
B_SPLINE_CURVE(2,(#78970,#78971,#78972),.UNSPECIFIED.,.F.,.F.)
B_SPLINE_CURVE_WITH_KNOTS((3,3),(0.,0.0915683004544683),.UNSPECIFIED.)
CURVE()
GEOMETRIC_REPRESENTATION_ITEM()
RATIONAL_B_SPLINE_CURVE((1.,1.00004989698968,1.00004421977447))
REPRESENTATION_ITEM('')
);
#19441=(
BOUNDED_CURVE()
B_SPLINE_CURVE(2,(#78978,#78979,#78980),.UNSPECIFIED.,.F.,.F.)
B_SPLINE_CURVE_WITH_KNOTS((3,3),(0.0728598745393818,0.164428174992087),
 .UNSPECIFIED.)
CURVE()
GEOMETRIC_REPRESENTATION_ITEM()
RATIONAL_B_SPLINE_CURVE((1.00004421963559,1.00004989683296,1.))
REPRESENTATION_ITEM('')
);
#19442=(
BOUNDED_CURVE()
B_SPLINE_CURVE(2,(#78991,#78992,#78993),.UNSPECIFIED.,.F.,.F.)
B_SPLINE_CURVE_WITH_KNOTS((3,3),(0.526544758504312,0.808610241550332),
 .UNSPECIFIED.)
CURVE()
GEOMETRIC_REPRESENTATION_ITEM()
RATIONAL_B_SPLINE_CURVE((1.00594694470061,1.00650257927333,1.00594694470061))
REPRESENTATION_ITEM('')
);
#19443=(
BOUNDED_CURVE()
B_SPLINE_CURVE(2,(#78998,#78999,#79000),.UNSPECIFIED.,.F.,.F.)
B_SPLINE_CURVE_WITH_KNOTS((3,3),(0.0728598752332843,0.164428174992088),
 .UNSPECIFIED.)
CURVE()
GEOMETRIC_REPRESENTATION_ITEM()
RATIONAL_B_SPLINE_CURVE((1.00004421930454,1.00004989645893,1.))
REPRESENTATION_ITEM('')
);
#19444=(
BOUNDED_CURVE()
B_SPLINE_CURVE(2,(#79011,#79012,#79013),.UNSPECIFIED.,.F.,.F.)
B_SPLINE_CURVE_WITH_KNOTS((3,3),(0.52654475850433,0.808610241550344),
 .UNSPECIFIED.)
CURVE()
GEOMETRIC_REPRESENTATION_ITEM()
RATIONAL_B_SPLINE_CURVE((1.00594694470059,1.00650257927331,1.00594694470059))
REPRESENTATION_ITEM('')
);
#19445=(
BOUNDED_CURVE()
B_SPLINE_CURVE(2,(#79018,#79019,#79020),.UNSPECIFIED.,.F.,.F.)
B_SPLINE_CURVE_WITH_KNOTS((3,3),(0.072859875072559,0.164428174992087),
 .UNSPECIFIED.)
CURVE()
GEOMETRIC_REPRESENTATION_ITEM()
RATIONAL_B_SPLINE_CURVE((1.00004421966611,1.00004989686704,1.))
REPRESENTATION_ITEM('')
);
#19446=(
BOUNDED_CURVE()
B_SPLINE_CURVE(2,(#79031,#79032,#79033),.UNSPECIFIED.,.F.,.F.)
B_SPLINE_CURVE_WITH_KNOTS((3,3),(0.526544758504327,0.808610241550334),
 .UNSPECIFIED.)
CURVE()
GEOMETRIC_REPRESENTATION_ITEM()
RATIONAL_B_SPLINE_CURVE((1.00594694470057,1.00650257927328,1.00594694470057))
REPRESENTATION_ITEM('')
);
#19447=(
BOUNDED_CURVE()
B_SPLINE_CURVE(2,(#79038,#79039,#79040),.UNSPECIFIED.,.F.,.F.)
B_SPLINE_CURVE_WITH_KNOTS((3,3),(0.0728598742504614,0.164428174992087),
 .UNSPECIFIED.)
CURVE()
GEOMETRIC_REPRESENTATION_ITEM()
RATIONAL_B_SPLINE_CURVE((1.0000442198312,1.00004989705388,1.))
REPRESENTATION_ITEM('')
);
#19448=(
BOUNDED_CURVE()
B_SPLINE_CURVE(2,(#79051,#79052,#79053),.UNSPECIFIED.,.F.,.F.)
B_SPLINE_CURVE_WITH_KNOTS((3,3),(0.526544758504325,0.808610241550338),
 .UNSPECIFIED.)
CURVE()
GEOMETRIC_REPRESENTATION_ITEM()
RATIONAL_B_SPLINE_CURVE((1.00594694470059,1.0065025792733,1.00594694470059))
REPRESENTATION_ITEM('')
);
#19449=(
BOUNDED_CURVE()
B_SPLINE_CURVE(2,(#79058,#79059,#79060),.UNSPECIFIED.,.F.,.F.)
B_SPLINE_CURVE_WITH_KNOTS((3,3),(0.0728598740519051,0.164428174992087),
 .UNSPECIFIED.)
CURVE()
GEOMETRIC_REPRESENTATION_ITEM()
RATIONAL_B_SPLINE_CURVE((1.00004421980835,1.00004989702823,1.))
REPRESENTATION_ITEM('')
);
#19450=(
BOUNDED_CURVE()
B_SPLINE_CURVE(2,(#79071,#79072,#79073),.UNSPECIFIED.,.F.,.F.)
B_SPLINE_CURVE_WITH_KNOTS((3,3),(0.526544758504316,0.808610241550331),
 .UNSPECIFIED.)
CURVE()
GEOMETRIC_REPRESENTATION_ITEM()
RATIONAL_B_SPLINE_CURVE((1.0059469447006,1.00650257927331,1.0059469447006))
REPRESENTATION_ITEM('')
);
#19451=(
BOUNDED_CURVE()
B_SPLINE_CURVE(2,(#79078,#79079,#79080),.UNSPECIFIED.,.F.,.F.)
B_SPLINE_CURVE_WITH_KNOTS((3,3),(0.0728598732895676,0.164428174992087),
 .UNSPECIFIED.)
CURVE()
GEOMETRIC_REPRESENTATION_ITEM()
RATIONAL_B_SPLINE_CURVE((1.00004422030706,1.0000498975915,1.))
REPRESENTATION_ITEM('')
);
#19452=(
BOUNDED_CURVE()
B_SPLINE_CURVE(2,(#79091,#79092,#79093),.UNSPECIFIED.,.F.,.F.)
B_SPLINE_CURVE_WITH_KNOTS((3,3),(0.526544758504325,0.808610241550338),
 .UNSPECIFIED.)
CURVE()
GEOMETRIC_REPRESENTATION_ITEM()
RATIONAL_B_SPLINE_CURVE((1.00594694470059,1.0065025792733,1.00594694470059))
REPRESENTATION_ITEM('')
);
#19453=(
BOUNDED_CURVE()
B_SPLINE_CURVE(2,(#79098,#79099,#79100),.UNSPECIFIED.,.F.,.F.)
B_SPLINE_CURVE_WITH_KNOTS((3,3),(0.0728598732782704,0.164428174992087),
 .UNSPECIFIED.)
CURVE()
GEOMETRIC_REPRESENTATION_ITEM()
RATIONAL_B_SPLINE_CURVE((1.00004422011247,1.00004989737192,1.))
REPRESENTATION_ITEM('')
);
#19454=(
BOUNDED_CURVE()
B_SPLINE_CURVE(2,(#79111,#79112,#79113),.UNSPECIFIED.,.F.,.F.)
B_SPLINE_CURVE_WITH_KNOTS((3,3),(0.526544758504328,0.808610241550337),
 .UNSPECIFIED.)
CURVE()
GEOMETRIC_REPRESENTATION_ITEM()
RATIONAL_B_SPLINE_CURVE((1.00594694470057,1.00650257927329,1.00594694470057))
REPRESENTATION_ITEM('')
);
#19455=(
BOUNDED_CURVE()
B_SPLINE_CURVE(2,(#79118,#79119,#79120),.UNSPECIFIED.,.F.,.F.)
B_SPLINE_CURVE_WITH_KNOTS((3,3),(0.0728598738456803,0.164428174992088),
 .UNSPECIFIED.)
CURVE()
GEOMETRIC_REPRESENTATION_ITEM()
RATIONAL_B_SPLINE_CURVE((1.0000442203771,1.00004989767014,1.))
REPRESENTATION_ITEM('')
);
#19456=(
BOUNDED_CURVE()
B_SPLINE_CURVE(2,(#79131,#79132,#79133),.UNSPECIFIED.,.F.,.F.)
B_SPLINE_CURVE_WITH_KNOTS((3,3),(0.526544758504326,0.808610241550336),
 .UNSPECIFIED.)
CURVE()
GEOMETRIC_REPRESENTATION_ITEM()
RATIONAL_B_SPLINE_CURVE((1.00594694470058,1.00650257927329,1.00594694470058))
REPRESENTATION_ITEM('')
);
#19457=(
BOUNDED_CURVE()
B_SPLINE_CURVE(2,(#79138,#79139,#79140),.UNSPECIFIED.,.F.,.F.)
B_SPLINE_CURVE_WITH_KNOTS((3,3),(0.0728598743728024,0.164428174992087),
 .UNSPECIFIED.)
CURVE()
GEOMETRIC_REPRESENTATION_ITEM()
RATIONAL_B_SPLINE_CURVE((1.00004421963814,1.00004989683596,1.))
REPRESENTATION_ITEM('')
);
#19458=(
BOUNDED_CURVE()
B_SPLINE_CURVE(2,(#79151,#79152,#79153),.UNSPECIFIED.,.F.,.F.)
B_SPLINE_CURVE_WITH_KNOTS((3,3),(0.526544758504329,0.808610241550345),
 .UNSPECIFIED.)
CURVE()
GEOMETRIC_REPRESENTATION_ITEM()
RATIONAL_B_SPLINE_CURVE((1.0059469447006,1.00650257927331,1.0059469447006))
REPRESENTATION_ITEM('')
);
#19459=(
BOUNDED_CURVE()
B_SPLINE_CURVE(2,(#79158,#79159,#79160),.UNSPECIFIED.,.F.,.F.)
B_SPLINE_CURVE_WITH_KNOTS((3,3),(0.0728598738250905,0.164428174992087),
 .UNSPECIFIED.)
CURVE()
GEOMETRIC_REPRESENTATION_ITEM()
RATIONAL_B_SPLINE_CURVE((1.00004422075857,1.0000498981006,1.))
REPRESENTATION_ITEM('')
);
#19460=(
BOUNDED_CURVE()
B_SPLINE_CURVE(2,(#79171,#79172,#79173),.UNSPECIFIED.,.F.,.F.)
B_SPLINE_CURVE_WITH_KNOTS((3,3),(0.526544758504326,0.808610241550335),
 .UNSPECIFIED.)
CURVE()
GEOMETRIC_REPRESENTATION_ITEM()
RATIONAL_B_SPLINE_CURVE((1.00594694470058,1.00650257927329,1.00594694470058))
REPRESENTATION_ITEM('')
);
#19461=(
BOUNDED_CURVE()
B_SPLINE_CURVE(2,(#79178,#79179,#79180),.UNSPECIFIED.,.F.,.F.)
B_SPLINE_CURVE_WITH_KNOTS((3,3),(0.0728598725540691,0.164428174992087),
 .UNSPECIFIED.)
CURVE()
GEOMETRIC_REPRESENTATION_ITEM()
RATIONAL_B_SPLINE_CURVE((1.00004422004749,1.00004989729911,1.))
REPRESENTATION_ITEM('')
);
#19462=(
BOUNDED_CURVE()
B_SPLINE_CURVE(2,(#79191,#79192,#79193),.UNSPECIFIED.,.F.,.F.)
B_SPLINE_CURVE_WITH_KNOTS((3,3),(0.526544758504315,0.808610241550331),
 .UNSPECIFIED.)
CURVE()
GEOMETRIC_REPRESENTATION_ITEM()
RATIONAL_B_SPLINE_CURVE((1.0059469447006,1.00650257927331,1.0059469447006))
REPRESENTATION_ITEM('')
);
#19463=(
BOUNDED_CURVE()
B_SPLINE_CURVE(2,(#79198,#79199,#79200),.UNSPECIFIED.,.F.,.F.)
B_SPLINE_CURVE_WITH_KNOTS((3,3),(0.0728598737482156,0.164428174992087),
 .UNSPECIFIED.)
CURVE()
GEOMETRIC_REPRESENTATION_ITEM()
RATIONAL_B_SPLINE_CURVE((1.00004421992039,1.00004989715487,1.))
REPRESENTATION_ITEM('')
);
#19464=(
BOUNDED_CURVE()
B_SPLINE_CURVE(2,(#79211,#79212,#79213),.UNSPECIFIED.,.F.,.F.)
B_SPLINE_CURVE_WITH_KNOTS((3,3),(0.52654475850433,0.808610241550342),
 .UNSPECIFIED.)
CURVE()
GEOMETRIC_REPRESENTATION_ITEM()
RATIONAL_B_SPLINE_CURVE((1.00594694470058,1.0065025792733,1.00594694470058))
REPRESENTATION_ITEM('')
);
#19465=(
BOUNDED_CURVE()
B_SPLINE_CURVE(2,(#79218,#79219,#79220),.UNSPECIFIED.,.F.,.F.)
B_SPLINE_CURVE_WITH_KNOTS((3,3),(0.07285987336842,0.164428174992087),
 .UNSPECIFIED.)
CURVE()
GEOMETRIC_REPRESENTATION_ITEM()
RATIONAL_B_SPLINE_CURVE((1.00004422018813,1.00004989745724,1.))
REPRESENTATION_ITEM('')
);
#19466=(
BOUNDED_CURVE()
B_SPLINE_CURVE(2,(#79231,#79232,#79233),.UNSPECIFIED.,.F.,.F.)
B_SPLINE_CURVE_WITH_KNOTS((3,3),(0.526544758504316,0.808610241550331),
 .UNSPECIFIED.)
CURVE()
GEOMETRIC_REPRESENTATION_ITEM()
RATIONAL_B_SPLINE_CURVE((1.0059469447006,1.00650257927331,1.0059469447006))
REPRESENTATION_ITEM('')
);
#19467=(
BOUNDED_CURVE()
B_SPLINE_CURVE(2,(#79238,#79239,#79240),.UNSPECIFIED.,.F.,.F.)
B_SPLINE_CURVE_WITH_KNOTS((3,3),(0.0728598727455658,0.164428174992087),
 .UNSPECIFIED.)
CURVE()
GEOMETRIC_REPRESENTATION_ITEM()
RATIONAL_B_SPLINE_CURVE((1.00004422062249,1.00004989794779,1.))
REPRESENTATION_ITEM('')
);
#19468=(
BOUNDED_CURVE()
B_SPLINE_CURVE(2,(#79251,#79252,#79253),.UNSPECIFIED.,.F.,.F.)
B_SPLINE_CURVE_WITH_KNOTS((3,3),(0.526544758504326,0.808610241550338),
 .UNSPECIFIED.)
CURVE()
GEOMETRIC_REPRESENTATION_ITEM()
RATIONAL_B_SPLINE_CURVE((1.00594694470059,1.0065025792733,1.00594694470059))
REPRESENTATION_ITEM('')
);
#19469=(
BOUNDED_CURVE()
B_SPLINE_CURVE(2,(#79258,#79259,#79260),.UNSPECIFIED.,.F.,.F.)
B_SPLINE_CURVE_WITH_KNOTS((3,3),(0.0728598739743273,0.164428174992087),
 .UNSPECIFIED.)
CURVE()
GEOMETRIC_REPRESENTATION_ITEM()
RATIONAL_B_SPLINE_CURVE((1.00004421975389,1.00004989696683,1.))
REPRESENTATION_ITEM('')
);
#19470=(
BOUNDED_CURVE()
B_SPLINE_CURVE(2,(#79271,#79272,#79273),.UNSPECIFIED.,.F.,.F.)
B_SPLINE_CURVE_WITH_KNOTS((3,3),(0.52654475850433,0.808610241550343),
 .UNSPECIFIED.)
CURVE()
GEOMETRIC_REPRESENTATION_ITEM()
RATIONAL_B_SPLINE_CURVE((1.00594694470059,1.0065025792733,1.00594694470059))
REPRESENTATION_ITEM('')
);
#19471=(
BOUNDED_CURVE()
B_SPLINE_CURVE(2,(#79278,#79279,#79280),.UNSPECIFIED.,.F.,.F.)
B_SPLINE_CURVE_WITH_KNOTS((3,3),(0.0728598738465884,0.164428174992087),
 .UNSPECIFIED.)
CURVE()
GEOMETRIC_REPRESENTATION_ITEM()
RATIONAL_B_SPLINE_CURVE((1.0000442201497,1.00004989741356,1.))
REPRESENTATION_ITEM('')
);
#19472=(
BOUNDED_CURVE()
B_SPLINE_CURVE(2,(#79291,#79292,#79293),.UNSPECIFIED.,.F.,.F.)
B_SPLINE_CURVE_WITH_KNOTS((3,3),(0.526544758504314,0.80861024155033),
 .UNSPECIFIED.)
CURVE()
GEOMETRIC_REPRESENTATION_ITEM()
RATIONAL_B_SPLINE_CURVE((1.0059469447006,1.00650257927332,1.0059469447006))
REPRESENTATION_ITEM('')
);
#19473=(
BOUNDED_CURVE()
B_SPLINE_CURVE(2,(#79298,#79299,#79300),.UNSPECIFIED.,.F.,.F.)
B_SPLINE_CURVE_WITH_KNOTS((3,3),(0.0728598743812492,0.164428174992087),
 .UNSPECIFIED.)
CURVE()
GEOMETRIC_REPRESENTATION_ITEM()
RATIONAL_B_SPLINE_CURVE((1.00004422004264,1.00004989729238,1.))
REPRESENTATION_ITEM('')
);
#19474=(
BOUNDED_CURVE()
B_SPLINE_CURVE(2,(#79311,#79312,#79313),.UNSPECIFIED.,.F.,.F.)
B_SPLINE_CURVE_WITH_KNOTS((3,3),(0.526544758504329,0.808610241550345),
 .UNSPECIFIED.)
CURVE()
GEOMETRIC_REPRESENTATION_ITEM()
RATIONAL_B_SPLINE_CURVE((1.0059469447006,1.00650257927331,1.0059469447006))
REPRESENTATION_ITEM('')
);
#19475=(
BOUNDED_CURVE()
B_SPLINE_CURVE(2,(#79318,#79319,#79320),.UNSPECIFIED.,.F.,.F.)
B_SPLINE_CURVE_WITH_KNOTS((3,3),(0.0728598751562594,0.164428174992087),
 .UNSPECIFIED.)
CURVE()
GEOMETRIC_REPRESENTATION_ITEM()
RATIONAL_B_SPLINE_CURVE((1.00004421953408,1.000049896718,1.))
REPRESENTATION_ITEM('')
);
#19476=(
BOUNDED_CURVE()
B_SPLINE_CURVE(2,(#79331,#79332,#79333),.UNSPECIFIED.,.F.,.F.)
B_SPLINE_CURVE_WITH_KNOTS((3,3),(0.526544758504326,0.808610241550335),
 .UNSPECIFIED.)
CURVE()
GEOMETRIC_REPRESENTATION_ITEM()
RATIONAL_B_SPLINE_CURVE((1.00594694470057,1.00650257927328,1.00594694470057))
REPRESENTATION_ITEM('')
);
#19477=(
BOUNDED_CURVE()
B_SPLINE_CURVE(2,(#79338,#79339,#79340),.UNSPECIFIED.,.F.,.F.)
B_SPLINE_CURVE_WITH_KNOTS((3,3),(0.0728598745734469,0.164428174992087),
 .UNSPECIFIED.)
CURVE()
GEOMETRIC_REPRESENTATION_ITEM()
RATIONAL_B_SPLINE_CURVE((1.00004421949713,1.0000498966767,1.))
REPRESENTATION_ITEM('')
);
#19478=(
BOUNDED_CURVE()
B_SPLINE_CURVE(2,(#79351,#79352,#79353),.UNSPECIFIED.,.F.,.F.)
B_SPLINE_CURVE_WITH_KNOTS((3,3),(0.526544758504326,0.808610241550333),
 .UNSPECIFIED.)
CURVE()
GEOMETRIC_REPRESENTATION_ITEM()
RATIONAL_B_SPLINE_CURVE((1.00594694470057,1.00650257927328,1.00594694470057))
REPRESENTATION_ITEM('')
);
#19479=(
BOUNDED_CURVE()
B_SPLINE_CURVE(2,(#79358,#79359,#79360),.UNSPECIFIED.,.F.,.F.)
B_SPLINE_CURVE_WITH_KNOTS((3,3),(0.0728598743491898,0.164428174992087),
 .UNSPECIFIED.)
CURVE()
GEOMETRIC_REPRESENTATION_ITEM()
RATIONAL_B_SPLINE_CURVE((1.00004421963837,1.00004989683623,1.))
REPRESENTATION_ITEM('')
);
#19480=(
BOUNDED_CURVE()
B_SPLINE_CURVE(2,(#79371,#79372,#79373),.UNSPECIFIED.,.F.,.F.)
B_SPLINE_CURVE_WITH_KNOTS((3,3),(0.526544758504326,0.808610241550337),
 .UNSPECIFIED.)
CURVE()
GEOMETRIC_REPRESENTATION_ITEM()
RATIONAL_B_SPLINE_CURVE((1.00594694470058,1.0065025792733,1.00594694470058))
REPRESENTATION_ITEM('')
);
#19481=(
BOUNDED_CURVE()
B_SPLINE_CURVE(2,(#79378,#79379,#79380),.UNSPECIFIED.,.F.,.F.)
B_SPLINE_CURVE_WITH_KNOTS((3,3),(0.0728598737483212,0.164428174992087),
 .UNSPECIFIED.)
CURVE()
GEOMETRIC_REPRESENTATION_ITEM()
RATIONAL_B_SPLINE_CURVE((1.00004421992501,1.00004989716008,1.))
REPRESENTATION_ITEM('')
);
#19482=(
BOUNDED_CURVE()
B_SPLINE_CURVE(2,(#79391,#79392,#79393),.UNSPECIFIED.,.F.,.F.)
B_SPLINE_CURVE_WITH_KNOTS((3,3),(0.526544758504331,0.808610241550341),
 .UNSPECIFIED.)
CURVE()
GEOMETRIC_REPRESENTATION_ITEM()
RATIONAL_B_SPLINE_CURVE((1.00594694470057,1.00650257927329,1.00594694470057))
REPRESENTATION_ITEM('')
);
#19483=(
BOUNDED_CURVE()
B_SPLINE_CURVE(2,(#79398,#79399,#79400),.UNSPECIFIED.,.F.,.F.)
B_SPLINE_CURVE_WITH_KNOTS((3,3),(0.0728598731298684,0.164428174992087),
 .UNSPECIFIED.)
CURVE()
GEOMETRIC_REPRESENTATION_ITEM()
RATIONAL_B_SPLINE_CURVE((1.00004422024797,1.00004989752493,1.))
REPRESENTATION_ITEM('')
);
#19484=(
BOUNDED_CURVE()
B_SPLINE_CURVE(2,(#79411,#79412,#79413),.UNSPECIFIED.,.F.,.F.)
B_SPLINE_CURVE_WITH_KNOTS((3,3),(0.526544758504314,0.80861024155033),
 .UNSPECIFIED.)
CURVE()
GEOMETRIC_REPRESENTATION_ITEM()
RATIONAL_B_SPLINE_CURVE((1.0059469447006,1.00650257927331,1.0059469447006))
REPRESENTATION_ITEM('')
);
#19485=(
BOUNDED_CURVE()
B_SPLINE_CURVE(2,(#79418,#79419,#79420),.UNSPECIFIED.,.F.,.F.)
B_SPLINE_CURVE_WITH_KNOTS((3,3),(0.0728598731596,0.164428174992087),
 .UNSPECIFIED.)
CURVE()
GEOMETRIC_REPRESENTATION_ITEM()
RATIONAL_B_SPLINE_CURVE((1.00004421993844,1.00004989717563,1.))
REPRESENTATION_ITEM('')
);
#19486=(
BOUNDED_CURVE()
B_SPLINE_CURVE(2,(#79431,#79432,#79433),.UNSPECIFIED.,.F.,.F.)
B_SPLINE_CURVE_WITH_KNOTS((3,3),(0.526544758504325,0.808610241550336),
 .UNSPECIFIED.)
CURVE()
GEOMETRIC_REPRESENTATION_ITEM()
RATIONAL_B_SPLINE_CURVE((1.00594694470058,1.00650257927329,1.00594694470058))
REPRESENTATION_ITEM('')
);
#19487=(
BOUNDED_CURVE()
B_SPLINE_CURVE(2,(#79438,#79439,#79440),.UNSPECIFIED.,.F.,.F.)
B_SPLINE_CURVE_WITH_KNOTS((3,3),(0.0728598731840463,0.164428174992087),
 .UNSPECIFIED.)
CURVE()
GEOMETRIC_REPRESENTATION_ITEM()
RATIONAL_B_SPLINE_CURVE((1.00004422050293,1.00004989781259,1.))
REPRESENTATION_ITEM('')
);
#19488=(
BOUNDED_CURVE()
B_SPLINE_CURVE(2,(#79451,#79452,#79453),.UNSPECIFIED.,.F.,.F.)
B_SPLINE_CURVE_WITH_KNOTS((3,3),(0.526544758504328,0.808610241550335),
 .UNSPECIFIED.)
CURVE()
GEOMETRIC_REPRESENTATION_ITEM()
RATIONAL_B_SPLINE_CURVE((1.00594694470057,1.00650257927328,1.00594694470057))
REPRESENTATION_ITEM('')
);
#19489=(
BOUNDED_CURVE()
B_SPLINE_CURVE(2,(#79458,#79459,#79460),.UNSPECIFIED.,.F.,.F.)
B_SPLINE_CURVE_WITH_KNOTS((3,3),(0.0728598743730364,0.164428174992087),
 .UNSPECIFIED.)
CURVE()
GEOMETRIC_REPRESENTATION_ITEM()
RATIONAL_B_SPLINE_CURVE((1.00004421961452,1.0000498968093,1.))
REPRESENTATION_ITEM('')
);
#19490=(
BOUNDED_CURVE()
B_SPLINE_CURVE(2,(#79471,#79472,#79473),.UNSPECIFIED.,.F.,.F.)
B_SPLINE_CURVE_WITH_KNOTS((3,3),(0.526544758504321,0.80861024155034),
 .UNSPECIFIED.)
CURVE()
GEOMETRIC_REPRESENTATION_ITEM()
RATIONAL_B_SPLINE_CURVE((1.00594694470061,1.00650257927332,1.00594694470061))
REPRESENTATION_ITEM('')
);
#19491=(
BOUNDED_CURVE()
B_SPLINE_CURVE(2,(#79478,#79479,#79480),.UNSPECIFIED.,.F.,.F.)
B_SPLINE_CURVE_WITH_KNOTS((3,3),(0.0728598738321962,0.164428174992087),
 .UNSPECIFIED.)
CURVE()
GEOMETRIC_REPRESENTATION_ITEM()
RATIONAL_B_SPLINE_CURVE((1.00004422004048,1.00004989729031,1.))
REPRESENTATION_ITEM('')
);
#19492=(
BOUNDED_CURVE()
B_SPLINE_CURVE(2,(#79491,#79492,#79493),.UNSPECIFIED.,.F.,.F.)
B_SPLINE_CURVE_WITH_KNOTS((3,3),(0.526544758504326,0.808610241550336),
 .UNSPECIFIED.)
CURVE()
GEOMETRIC_REPRESENTATION_ITEM()
RATIONAL_B_SPLINE_CURVE((1.00594694470058,1.00650257927329,1.00594694470058))
REPRESENTATION_ITEM('')
);
#19493=(
BOUNDED_CURVE()
B_SPLINE_CURVE(2,(#79498,#79499,#79500),.UNSPECIFIED.,.F.,.F.)
B_SPLINE_CURVE_WITH_KNOTS((3,3),(0.0728598739247914,0.164428174992087),
 .UNSPECIFIED.)
CURVE()
GEOMETRIC_REPRESENTATION_ITEM()
RATIONAL_B_SPLINE_CURVE((1.00004422012998,1.00004989739124,1.))
REPRESENTATION_ITEM('')
);
#19494=(
BOUNDED_CURVE()
B_SPLINE_CURVE(2,(#79511,#79512,#79513),.UNSPECIFIED.,.F.,.F.)
B_SPLINE_CURVE_WITH_KNOTS((3,3),(0.526544758504326,0.808610241550334),
 .UNSPECIFIED.)
CURVE()
GEOMETRIC_REPRESENTATION_ITEM()
RATIONAL_B_SPLINE_CURVE((1.00594694470057,1.00650257927328,1.00594694470057))
REPRESENTATION_ITEM('')
);
#19495=(
BOUNDED_CURVE()
B_SPLINE_CURVE(2,(#79518,#79519,#79520),.UNSPECIFIED.,.F.,.F.)
B_SPLINE_CURVE_WITH_KNOTS((3,3),(0.0728598736288243,0.164428174992087),
 .UNSPECIFIED.)
CURVE()
GEOMETRIC_REPRESENTATION_ITEM()
RATIONAL_B_SPLINE_CURVE((1.00004422053539,1.00004989784891,1.))
REPRESENTATION_ITEM('')
);
#19496=(
BOUNDED_CURVE()
B_SPLINE_CURVE(2,(#79531,#79532,#79533),.UNSPECIFIED.,.F.,.F.)
B_SPLINE_CURVE_WITH_KNOTS((3,3),(0.526544758504324,0.808610241550337),
 .UNSPECIFIED.)
CURVE()
GEOMETRIC_REPRESENTATION_ITEM()
RATIONAL_B_SPLINE_CURVE((1.00594694470059,1.0065025792733,1.00594694470059))
REPRESENTATION_ITEM('')
);
#19497=(
BOUNDED_CURVE()
B_SPLINE_CURVE(2,(#79538,#79539,#79540),.UNSPECIFIED.,.F.,.F.)
B_SPLINE_CURVE_WITH_KNOTS((3,3),(0.0728598730615147,0.164428174992087),
 .UNSPECIFIED.)
CURVE()
GEOMETRIC_REPRESENTATION_ITEM()
RATIONAL_B_SPLINE_CURVE((1.00004422030862,1.00004989759341,1.))
REPRESENTATION_ITEM('')
);
#19498=(
BOUNDED_CURVE()
B_SPLINE_CURVE(2,(#79551,#79552,#79553),.UNSPECIFIED.,.F.,.F.)
B_SPLINE_CURVE_WITH_KNOTS((3,3),(0.526544758504332,0.808610241550341),
 .UNSPECIFIED.)
CURVE()
GEOMETRIC_REPRESENTATION_ITEM()
RATIONAL_B_SPLINE_CURVE((1.00594694470057,1.00650257927329,1.00594694470057))
REPRESENTATION_ITEM('')
);
#19499=(
BOUNDED_CURVE()
B_SPLINE_CURVE(2,(#79558,#79559,#79560),.UNSPECIFIED.,.F.,.F.)
B_SPLINE_CURVE_WITH_KNOTS((3,3),(0.07285987336842,0.164428174992087),
 .UNSPECIFIED.)
CURVE()
GEOMETRIC_REPRESENTATION_ITEM()
RATIONAL_B_SPLINE_CURVE((1.00004422018813,1.00004989745724,1.))
REPRESENTATION_ITEM('')
);
#19500=(
BOUNDED_CURVE()
B_SPLINE_CURVE(2,(#79571,#79572,#79573),.UNSPECIFIED.,.F.,.F.)
B_SPLINE_CURVE_WITH_KNOTS((3,3),(0.526544758504316,0.808610241550331),
 .UNSPECIFIED.)
CURVE()
GEOMETRIC_REPRESENTATION_ITEM()
RATIONAL_B_SPLINE_CURVE((1.0059469447006,1.00650257927331,1.0059469447006))
REPRESENTATION_ITEM('')
);
#19501=(
BOUNDED_CURVE()
B_SPLINE_CURVE(2,(#79578,#79579,#79580),.UNSPECIFIED.,.F.,.F.)
B_SPLINE_CURVE_WITH_KNOTS((3,3),(0.0728598741162188,0.164428174992087),
 .UNSPECIFIED.)
CURVE()
GEOMETRIC_REPRESENTATION_ITEM()
RATIONAL_B_SPLINE_CURVE((1.00004421986125,1.00004989708788,1.))
REPRESENTATION_ITEM('')
);
#19502=(
BOUNDED_CURVE()
B_SPLINE_CURVE(2,(#79591,#79592,#79593),.UNSPECIFIED.,.F.,.F.)
B_SPLINE_CURVE_WITH_KNOTS((3,3),(0.526544758504326,0.808610241550337),
 .UNSPECIFIED.)
CURVE()
GEOMETRIC_REPRESENTATION_ITEM()
RATIONAL_B_SPLINE_CURVE((1.00594694470058,1.00650257927329,1.00594694470058))
REPRESENTATION_ITEM('')
);
#19503=(
BOUNDED_CURVE()
B_SPLINE_CURVE(2,(#79598,#79599,#79600),.UNSPECIFIED.,.F.,.F.)
B_SPLINE_CURVE_WITH_KNOTS((3,3),(0.0728598752298607,0.164428174992087),
 .UNSPECIFIED.)
CURVE()
GEOMETRIC_REPRESENTATION_ITEM()
RATIONAL_B_SPLINE_CURVE((1.00004421980288,1.00004989702126,1.))
REPRESENTATION_ITEM('')
);
#19504=(
BOUNDED_CURVE()
B_SPLINE_CURVE(2,(#79611,#79612,#79613),.UNSPECIFIED.,.F.,.F.)
B_SPLINE_CURVE_WITH_KNOTS((3,3),(0.526544758504327,0.808610241550334),
 .UNSPECIFIED.)
CURVE()
GEOMETRIC_REPRESENTATION_ITEM()
RATIONAL_B_SPLINE_CURVE((1.00594694470057,1.00650257927328,1.00594694470057))
REPRESENTATION_ITEM('')
);
#19505=(
BOUNDED_CURVE()
B_SPLINE_CURVE(2,(#79618,#79619,#79620),.UNSPECIFIED.,.F.,.F.)
B_SPLINE_CURVE_WITH_KNOTS((3,3),(0.0728598738446078,0.164428174992087),
 .UNSPECIFIED.)
CURVE()
GEOMETRIC_REPRESENTATION_ITEM()
RATIONAL_B_SPLINE_CURVE((1.00004422018383,1.00004989745207,1.))
REPRESENTATION_ITEM('')
);
#19506=(
BOUNDED_CURVE()
B_SPLINE_CURVE(2,(#79631,#79632,#79633),.UNSPECIFIED.,.F.,.F.)
B_SPLINE_CURVE_WITH_KNOTS((3,3),(0.526544758504328,0.808610241550334),
 .UNSPECIFIED.)
CURVE()
GEOMETRIC_REPRESENTATION_ITEM()
RATIONAL_B_SPLINE_CURVE((1.00594694470057,1.00650257927328,1.00594694470057))
REPRESENTATION_ITEM('')
);
#19507=(
BOUNDED_CURVE()
B_SPLINE_CURVE(2,(#79636,#79637,#79638),.UNSPECIFIED.,.F.,.F.)
B_SPLINE_CURVE_WITH_KNOTS((3,3),(0.,0.0915683004209703),.UNSPECIFIED.)
CURVE()
GEOMETRIC_REPRESENTATION_ITEM()
RATIONAL_B_SPLINE_CURVE((1.,1.00004989694773,1.00004421973732))
REPRESENTATION_ITEM('')
);
#19508=(
BOUNDED_CURVE()
B_SPLINE_CURVE(2,(#79642,#79643,#79644),.UNSPECIFIED.,.F.,.F.)
B_SPLINE_CURVE_WITH_KNOTS((3,3),(0.,0.0915683013231767),.UNSPECIFIED.)
CURVE()
GEOMETRIC_REPRESENTATION_ITEM()
RATIONAL_B_SPLINE_CURVE((1.,1.00004989713748,1.00004421990493))
REPRESENTATION_ITEM('')
);
#19509=(
BOUNDED_CURVE()
B_SPLINE_CURVE(2,(#79648,#79649,#79650),.UNSPECIFIED.,.F.,.F.)
B_SPLINE_CURVE_WITH_KNOTS((3,3),(0.,0.0915683016069819),.UNSPECIFIED.)
CURVE()
GEOMETRIC_REPRESENTATION_ITEM()
RATIONAL_B_SPLINE_CURVE((1.,1.00004989745717,1.00004422018807))
REPRESENTATION_ITEM('')
);
#19510=(
BOUNDED_CURVE()
B_SPLINE_CURVE(2,(#79654,#79655,#79656),.UNSPECIFIED.,.F.,.F.)
B_SPLINE_CURVE_WITH_KNOTS((3,3),(0.,0.0915683018592699),.UNSPECIFIED.)
CURVE()
GEOMETRIC_REPRESENTATION_ITEM()
RATIONAL_B_SPLINE_CURVE((1.,1.00004989730699,1.00004422005483))
REPRESENTATION_ITEM('')
);
#19511=(
BOUNDED_CURVE()
B_SPLINE_CURVE(2,(#79660,#79661,#79662),.UNSPECIFIED.,.F.,.F.)
B_SPLINE_CURVE_WITH_KNOTS((3,3),(0.,0.0915683015335247),.UNSPECIFIED.)
CURVE()
GEOMETRIC_REPRESENTATION_ITEM()
RATIONAL_B_SPLINE_CURVE((1.,1.00004989745986,1.00004422019051))
REPRESENTATION_ITEM('')
);
#19512=(
BOUNDED_CURVE()
B_SPLINE_CURVE(2,(#79666,#79667,#79668),.UNSPECIFIED.,.F.,.F.)
B_SPLINE_CURVE_WITH_KNOTS((3,3),(0.,0.0915683019494071),.UNSPECIFIED.)
CURVE()
GEOMETRIC_REPRESENTATION_ITEM()
RATIONAL_B_SPLINE_CURVE((1.,1.00004989707043,1.00004421984513))
REPRESENTATION_ITEM('')
);
#19513=(
BOUNDED_CURVE()
B_SPLINE_CURVE(2,(#79672,#79673,#79674),.UNSPECIFIED.,.F.,.F.)
B_SPLINE_CURVE_WITH_KNOTS((3,3),(0.,0.0915683011311358),.UNSPECIFIED.)
CURVE()
GEOMETRIC_REPRESENTATION_ITEM()
RATIONAL_B_SPLINE_CURVE((1.,1.00004989683837,1.00004421963997))
REPRESENTATION_ITEM('')
);
#19514=(
BOUNDED_CURVE()
B_SPLINE_CURVE(2,(#79678,#79679,#79680),.UNSPECIFIED.,.F.,.F.)
B_SPLINE_CURVE_WITH_KNOTS((3,3),(0.,0.091568300610644),.UNSPECIFIED.)
CURVE()
GEOMETRIC_REPRESENTATION_ITEM()
RATIONAL_B_SPLINE_CURVE((1.,1.0000498971937,1.00004421995519))
REPRESENTATION_ITEM('')
);
#19515=(
BOUNDED_CURVE()
B_SPLINE_CURVE(2,(#79684,#79685,#79686),.UNSPECIFIED.,.F.,.F.)
B_SPLINE_CURVE_WITH_KNOTS((3,3),(0.,0.0915683011636906),.UNSPECIFIED.)
CURVE()
GEOMETRIC_REPRESENTATION_ITEM()
RATIONAL_B_SPLINE_CURVE((1.,1.00004989770404,1.00004422040713))
REPRESENTATION_ITEM('')
);
#19516=(
BOUNDED_CURVE()
B_SPLINE_CURVE(2,(#79690,#79691,#79692),.UNSPECIFIED.,.F.,.F.)
B_SPLINE_CURVE_WITH_KNOTS((3,3),(0.,0.09156830042059),.UNSPECIFIED.)
CURVE()
GEOMETRIC_REPRESENTATION_ITEM()
RATIONAL_B_SPLINE_CURVE((1.,1.00004989687363,1.00004421967165))
REPRESENTATION_ITEM('')
);
#19517=(
BOUNDED_CURVE()
B_SPLINE_CURVE(2,(#79696,#79697,#79698),.UNSPECIFIED.,.F.,.F.)
B_SPLINE_CURVE_WITH_KNOTS((3,3),(0.,0.0915683014739308),.UNSPECIFIED.)
CURVE()
GEOMETRIC_REPRESENTATION_ITEM()
RATIONAL_B_SPLINE_CURVE((1.,1.00004989729695,1.00004422004617))
REPRESENTATION_ITEM('')
);
#19518=(
BOUNDED_CURVE()
B_SPLINE_CURVE(2,(#79702,#79703,#79704),.UNSPECIFIED.,.F.,.F.)
B_SPLINE_CURVE_WITH_KNOTS((3,3),(0.,0.0915683011482813),.UNSPECIFIED.)
CURVE()
GEOMETRIC_REPRESENTATION_ITEM()
RATIONAL_B_SPLINE_CURVE((1.,1.00004989719406,1.00004421995518))
REPRESENTATION_ITEM('')
);
#19519=(
BOUNDED_CURVE()
B_SPLINE_CURVE(2,(#79708,#79709,#79710),.UNSPECIFIED.,.F.,.F.)
B_SPLINE_CURVE_WITH_KNOTS((3,3),(0.,0.0915683008241534),.UNSPECIFIED.)
CURVE()
GEOMETRIC_REPRESENTATION_ITEM()
RATIONAL_B_SPLINE_CURVE((1.,1.00004989687854,1.00004421967576))
REPRESENTATION_ITEM('')
);
#19520=(
BOUNDED_CURVE()
B_SPLINE_CURVE(2,(#79714,#79715,#79716),.UNSPECIFIED.,.F.,.F.)
B_SPLINE_CURVE_WITH_KNOTS((3,3),(0.,0.0915683018469464),.UNSPECIFIED.)
CURVE()
GEOMETRIC_REPRESENTATION_ITEM()
RATIONAL_B_SPLINE_CURVE((1.,1.00004989759971,1.00004422031425))
REPRESENTATION_ITEM('')
);
#19521=(
BOUNDED_CURVE()
B_SPLINE_CURVE(2,(#79720,#79721,#79722),.UNSPECIFIED.,.F.,.F.)
B_SPLINE_CURVE_WITH_KNOTS((3,3),(0.,0.0915683017817766),.UNSPECIFIED.)
CURVE()
GEOMETRIC_REPRESENTATION_ITEM()
RATIONAL_B_SPLINE_CURVE((1.,1.0000498971653,1.00004421992931))
REPRESENTATION_ITEM('')
);
#19522=(
BOUNDED_CURVE()
B_SPLINE_CURVE(2,(#79726,#79727,#79728),.UNSPECIFIED.,.F.,.F.)
B_SPLINE_CURVE_WITH_KNOTS((3,3),(0.,0.0915683006548595),.UNSPECIFIED.)
CURVE()
GEOMETRIC_REPRESENTATION_ITEM()
RATIONAL_B_SPLINE_CURVE((1.,1.0000498974359,1.0000442201698))
REPRESENTATION_ITEM('')
);
#19523=(
BOUNDED_CURVE()
B_SPLINE_CURVE(2,(#79732,#79733,#79734),.UNSPECIFIED.,.F.,.F.)
B_SPLINE_CURVE_WITH_KNOTS((3,3),(0.,0.0915683004665198),.UNSPECIFIED.)
CURVE()
GEOMETRIC_REPRESENTATION_ITEM()
RATIONAL_B_SPLINE_CURVE((1.,1.00004989714855,1.00004421991526))
REPRESENTATION_ITEM('')
);
#19524=(
BOUNDED_CURVE()
B_SPLINE_CURVE(2,(#79738,#79739,#79740),.UNSPECIFIED.,.F.,.F.)
B_SPLINE_CURVE_WITH_KNOTS((3,3),(0.,0.0915683004318276),.UNSPECIFIED.)
CURVE()
GEOMETRIC_REPRESENTATION_ITEM()
RATIONAL_B_SPLINE_CURVE((1.,1.00004989712855,1.00004421989756))
REPRESENTATION_ITEM('')
);
#19525=(
BOUNDED_CURVE()
B_SPLINE_CURVE(2,(#79744,#79745,#79746),.UNSPECIFIED.,.F.,.F.)
B_SPLINE_CURVE_WITH_KNOTS((3,3),(0.,0.0915683013234486),.UNSPECIFIED.)
CURVE()
GEOMETRIC_REPRESENTATION_ITEM()
RATIONAL_B_SPLINE_CURVE((1.,1.00004989715502,1.00004421992048))
REPRESENTATION_ITEM('')
);
#19526=(
BOUNDED_CURVE()
B_SPLINE_CURVE(2,(#79750,#79751,#79752),.UNSPECIFIED.,.F.,.F.)
B_SPLINE_CURVE_WITH_KNOTS((3,3),(0.,0.0915683014442284),.UNSPECIFIED.)
CURVE()
GEOMETRIC_REPRESENTATION_ITEM()
RATIONAL_B_SPLINE_CURVE((1.,1.00004989755638,1.00004422027609))
REPRESENTATION_ITEM('')
);
#19527=(
BOUNDED_CURVE()
B_SPLINE_CURVE(2,(#79756,#79757,#79758),.UNSPECIFIED.,.F.,.F.)
B_SPLINE_CURVE_WITH_KNOTS((3,3),(0.,0.0915683018592699),.UNSPECIFIED.)
CURVE()
GEOMETRIC_REPRESENTATION_ITEM()
RATIONAL_B_SPLINE_CURVE((1.,1.00004989730699,1.00004422005483))
REPRESENTATION_ITEM('')
);
#19528=(
BOUNDED_CURVE()
B_SPLINE_CURVE(2,(#79762,#79763,#79764),.UNSPECIFIED.,.F.,.F.)
B_SPLINE_CURVE_WITH_KNOTS((3,3),(0.,0.0915683008497595),.UNSPECIFIED.)
CURVE()
GEOMETRIC_REPRESENTATION_ITEM()
RATIONAL_B_SPLINE_CURVE((1.,1.00004989695215,1.00004421974097))
REPRESENTATION_ITEM('')
);
#19529=(
BOUNDED_CURVE()
B_SPLINE_CURVE(2,(#79768,#79769,#79770),.UNSPECIFIED.,.F.,.F.)
B_SPLINE_CURVE_WITH_KNOTS((3,3),(0.,0.0915683018022691),.UNSPECIFIED.)
CURVE()
GEOMETRIC_REPRESENTATION_ITEM()
RATIONAL_B_SPLINE_CURVE((1.,1.00004989750928,1.00004422023414))
REPRESENTATION_ITEM('')
);
#19530=(
BOUNDED_CURVE()
B_SPLINE_CURVE(2,(#79774,#79775,#79776),.UNSPECIFIED.,.F.,.F.)
B_SPLINE_CURVE_WITH_KNOTS((3,3),(0.,0.0915683019430039),.UNSPECIFIED.)
CURVE()
GEOMETRIC_REPRESENTATION_ITEM()
RATIONAL_B_SPLINE_CURVE((1.,1.00004989754698,1.00004422026747))
REPRESENTATION_ITEM('')
);
#19531=(
BOUNDED_CURVE()
B_SPLINE_CURVE(2,(#79780,#79781,#79782),.UNSPECIFIED.,.F.,.F.)
B_SPLINE_CURVE_WITH_KNOTS((3,3),(0.,0.0915683004685661),.UNSPECIFIED.)
CURVE()
GEOMETRIC_REPRESENTATION_ITEM()
RATIONAL_B_SPLINE_CURVE((1.,1.00004989737201,1.0000442201133))
REPRESENTATION_ITEM('')
);
#19532=(
BOUNDED_CURVE()
B_SPLINE_CURVE(2,(#79786,#79787,#79788),.UNSPECIFIED.,.F.,.F.)
B_SPLINE_CURVE_WITH_KNOTS((3,3),(0.,0.0915683004311751),.UNSPECIFIED.)
CURVE()
GEOMETRIC_REPRESENTATION_ITEM()
RATIONAL_B_SPLINE_CURVE((1.,1.00004989703817,1.00004421981746))
REPRESENTATION_ITEM('')
);
#19533=(
BOUNDED_CURVE()
B_SPLINE_CURVE(2,(#79792,#79793,#79794),.UNSPECIFIED.,.F.,.F.)
B_SPLINE_CURVE_WITH_KNOTS((3,3),(0.,0.0915683015082938),.UNSPECIFIED.)
CURVE()
GEOMETRIC_REPRESENTATION_ITEM()
RATIONAL_B_SPLINE_CURVE((1.,1.00004989736684,1.00004422010808))
REPRESENTATION_ITEM('')
);
#19534=(
BOUNDED_CURVE()
B_SPLINE_CURVE(2,(#79798,#79799,#79800),.UNSPECIFIED.,.F.,.F.)
B_SPLINE_CURVE_WITH_KNOTS((3,3),(0.,0.0915683021230445),.UNSPECIFIED.)
CURVE()
GEOMETRIC_REPRESENTATION_ITEM()
RATIONAL_B_SPLINE_CURVE((1.,1.0000498975049,1.00004422023007))
REPRESENTATION_ITEM('')
);
#19535=(
BOUNDED_CURVE()
B_SPLINE_CURVE(2,(#79804,#79805,#79806),.UNSPECIFIED.,.F.,.F.)
B_SPLINE_CURVE_WITH_KNOTS((3,3),(0.,0.0915683025371453),.UNSPECIFIED.)
CURVE()
GEOMETRIC_REPRESENTATION_ITEM()
RATIONAL_B_SPLINE_CURVE((1.,1.00004989764124,1.00004422035064))
REPRESENTATION_ITEM('')
);
#19536=(
BOUNDED_CURVE()
B_SPLINE_CURVE(2,(#79810,#79811,#79812),.UNSPECIFIED.,.F.,.F.)
B_SPLINE_CURVE_WITH_KNOTS((3,3),(0.,0.0915683008645893),.UNSPECIFIED.)
CURVE()
GEOMETRIC_REPRESENTATION_ITEM()
RATIONAL_B_SPLINE_CURVE((1.,1.00004989751924,1.00004422024354))
REPRESENTATION_ITEM('')
);
#19537=(
BOUNDED_CURVE()
B_SPLINE_CURVE(2,(#79816,#79817,#79818),.UNSPECIFIED.,.F.,.F.)
B_SPLINE_CURVE_WITH_KNOTS((3,3),(0.,0.0915683010569264),.UNSPECIFIED.)
CURVE()
GEOMETRIC_REPRESENTATION_ITEM()
RATIONAL_B_SPLINE_CURVE((1.,1.00004989699498,1.00004421977881))
REPRESENTATION_ITEM('')
);
#19538=(
BOUNDED_CURVE()
B_SPLINE_CURVE(2,(#79822,#79823,#79824),.UNSPECIFIED.,.F.,.F.)
B_SPLINE_CURVE_WITH_KNOTS((3,3),(0.,0.0915683011449946),.UNSPECIFIED.)
CURVE()
GEOMETRIC_REPRESENTATION_ITEM()
RATIONAL_B_SPLINE_CURVE((1.,1.00004989725244,1.00004422000692))
REPRESENTATION_ITEM('')
);
#19539=(
BOUNDED_CURVE()
B_SPLINE_CURVE(2,(#79828,#79829,#79830),.UNSPECIFIED.,.F.,.F.)
B_SPLINE_CURVE_WITH_KNOTS((3,3),(0.,0.0915683013065163),.UNSPECIFIED.)
CURVE()
GEOMETRIC_REPRESENTATION_ITEM()
RATIONAL_B_SPLINE_CURVE((1.,1.00004989753082,1.00004422025353))
REPRESENTATION_ITEM('')
);
#19743=CIRCLE('',#53613,37.8);
#19744=CIRCLE('',#53614,37.8);
#19745=CIRCLE('',#53616,37.3);
#19746=CIRCLE('',#53617,37.8);
#19747=CIRCLE('',#53618,37.8);
#19748=CIRCLE('',#53619,37.8);
#19749=CIRCLE('',#53620,37.8);
#19750=CIRCLE('',#53621,37.8);
#19751=CIRCLE('',#53622,37.8);
#19752=CIRCLE('',#53623,37.8);
#19753=CIRCLE('',#53624,37.8);
#19754=CIRCLE('',#53625,37.8);
#19755=CIRCLE('',#53626,37.8);
#19756=CIRCLE('',#53627,37.8);
#19757=CIRCLE('',#53628,37.8);
#19758=CIRCLE('',#53630,37.3);
#19759=CIRCLE('',#53631,37.3);
#19760=CIRCLE('',#53632,37.3);
#19761=CIRCLE('',#53633,34.);
#19762=CIRCLE('',#53635,37.8);
#19763=CIRCLE('',#53636,37.8);
#19764=CIRCLE('',#53637,37.8);
#19765=CIRCLE('',#53638,37.8);
#19766=CIRCLE('',#53639,37.8);
#19767=CIRCLE('',#53640,37.8);
#19768=CIRCLE('',#53641,37.8);
#19769=CIRCLE('',#53642,37.8);
#19770=CIRCLE('',#53643,37.8);
#19771=CIRCLE('',#53644,37.8);
#19772=CIRCLE('',#53645,37.8);
#19773=CIRCLE('',#53646,37.8);
#19774=CIRCLE('',#53648,37.8);
#19775=CIRCLE('',#53649,37.8);
#19776=CIRCLE('',#53650,37.8);
#19777=CIRCLE('',#53651,37.8);
#19778=CIRCLE('',#53652,37.8);
#19779=CIRCLE('',#53653,37.8);
#19780=CIRCLE('',#53654,37.8);
#19781=CIRCLE('',#53655,37.8);
#19782=CIRCLE('',#53656,37.8);
#19783=CIRCLE('',#53657,37.8);
#19784=CIRCLE('',#53658,37.8);
#19785=CIRCLE('',#53663,37.3);
#19786=CIRCLE('',#53664,37.8);
#19787=CIRCLE('',#53665,37.8);
#19788=CIRCLE('',#53666,37.8);
#19789=CIRCLE('',#53667,37.8);
#19790=CIRCLE('',#53668,37.8);
#19791=CIRCLE('',#53669,37.8);
#19792=CIRCLE('',#53670,37.8);
#19793=CIRCLE('',#53671,37.8);
#19794=CIRCLE('',#53672,37.8);
#19795=CIRCLE('',#53673,37.8);
#19796=CIRCLE('',#53674,37.8);
#19797=CIRCLE('',#53675,37.8);
#19798=CIRCLE('',#53677,37.8);
#19799=CIRCLE('',#53678,37.8);
#19800=CIRCLE('',#53679,37.8);
#19801=CIRCLE('',#53680,37.8);
#19802=CIRCLE('',#53681,37.8);
#19803=CIRCLE('',#53682,37.8);
#19804=CIRCLE('',#53683,37.8);
#19805=CIRCLE('',#53684,37.8);
#19806=CIRCLE('',#53685,37.8);
#19807=CIRCLE('',#53686,37.8);
#19808=CIRCLE('',#53687,37.8);
#19809=CIRCLE('',#53688,37.3);
#19810=CIRCLE('',#53691,37.8);
#19811=CIRCLE('',#53692,37.8);
#19812=CIRCLE('',#53693,37.8);
#19813=CIRCLE('',#53694,37.8);
#19814=CIRCLE('',#53695,37.8);
#19815=CIRCLE('',#53696,37.8);
#19816=CIRCLE('',#53697,37.8);
#19817=CIRCLE('',#53698,37.8);
#19818=CIRCLE('',#53699,37.8);
#19819=CIRCLE('',#53700,37.8);
#19820=CIRCLE('',#53701,37.8);
#19821=CIRCLE('',#53702,37.8);
#19822=CIRCLE('',#53708,41.43);
#19823=CIRCLE('',#53710,41.43);
#19824=CIRCLE('',#53712,41.43);
#19825=CIRCLE('',#53714,41.43);
#19826=CIRCLE('',#53716,41.43);
#19827=CIRCLE('',#53718,41.43);
#19828=CIRCLE('',#53720,41.43);
#19829=CIRCLE('',#53722,41.43);
#19830=CIRCLE('',#53724,41.43);
#19831=CIRCLE('',#53726,41.43);
#19832=CIRCLE('',#53728,41.43);
#19833=CIRCLE('',#53730,41.43);
#19834=CIRCLE('',#53732,41.43);
#19835=CIRCLE('',#53734,41.43);
#19836=CIRCLE('',#53736,41.43);
#19837=CIRCLE('',#53738,41.43);
#19838=CIRCLE('',#53740,41.43);
#19839=CIRCLE('',#53742,41.43);
#19840=CIRCLE('',#53744,41.43);
#19841=CIRCLE('',#53746,41.43);
#19842=CIRCLE('',#53748,41.43);
#19843=CIRCLE('',#53750,41.43);
#19844=CIRCLE('',#53752,41.43);
#19845=CIRCLE('',#53754,41.43);
#19846=CIRCLE('',#53756,41.43);
#19847=CIRCLE('',#53758,41.43);
#19848=CIRCLE('',#53760,41.43);
#19849=CIRCLE('',#53762,41.43);
#19850=CIRCLE('',#53764,41.43);
#19851=CIRCLE('',#53766,41.43);
#19852=CIRCLE('',#53768,41.43);
#19853=CIRCLE('',#53770,41.43);
#19854=CIRCLE('',#53772,41.43);
#19855=CIRCLE('',#53840,41.43);
#19856=CIRCLE('',#53842,41.43);
#19857=CIRCLE('',#53844,41.43);
#19858=CIRCLE('',#53846,41.43);
#19859=CIRCLE('',#53848,41.43);
#19860=CIRCLE('',#53850,41.43);
#19861=CIRCLE('',#53852,41.43);
#19862=CIRCLE('',#53854,41.43);
#19863=CIRCLE('',#53856,41.43);
#19864=CIRCLE('',#53858,41.43);
#19865=CIRCLE('',#53860,41.43);
#19866=CIRCLE('',#53862,41.43);
#19867=CIRCLE('',#53864,41.43);
#19868=CIRCLE('',#53866,41.43);
#19869=CIRCLE('',#53868,41.43);
#19870=CIRCLE('',#53870,41.43);
#19871=CIRCLE('',#53872,41.43);
#19872=CIRCLE('',#53874,41.43);
#19873=CIRCLE('',#53876,41.43);
#19874=CIRCLE('',#53878,41.43);
#19875=CIRCLE('',#53880,41.43);
#19876=CIRCLE('',#53882,41.43);
#19877=CIRCLE('',#53884,41.43);
#19878=CIRCLE('',#53886,41.43);
#19879=CIRCLE('',#53888,41.43);
#19880=CIRCLE('',#53890,41.43);
#19881=CIRCLE('',#53892,41.43);
#19882=CIRCLE('',#53894,41.43);
#19883=CIRCLE('',#53896,41.43);
#19884=CIRCLE('',#53898,41.43);
#19885=CIRCLE('',#53900,41.43);
#19886=CIRCLE('',#53902,41.43);
#19887=CIRCLE('',#53904,41.43);
#19888=CIRCLE('',#54104,34.);
#19889=CIRCLE('',#54105,1.);
#19890=CIRCLE('',#54106,33.);
#19891=CIRCLE('',#54107,34.);
#19892=CIRCLE('',#54109,25.);
#19893=CIRCLE('',#54111,34.);
#19894=CIRCLE('',#54113,33.);
#19895=CIRCLE('',#54114,1.);
#19896=CIRCLE('',#54115,34.);
#19897=CIRCLE('',#54116,34.);
#19898=CIRCLE('',#54118,25.);
#19899=CIRCLE('',#54121,1.);
#19900=CIRCLE('',#54122,24.);
#19901=CIRCLE('',#54123,24.);
#19902=CIRCLE('',#54125,24.);
#19903=CIRCLE('',#54127,24.);
#19904=CIRCLE('',#54128,1.);
#19905=CIRCLE('',#54129,24.);
#19906=CIRCLE('',#54131,24.);
#19907=CIRCLE('',#54133,15.01);
#19908=CIRCLE('',#54134,15.01);
#19909=CIRCLE('',#54136,15.81);
#19910=CIRCLE('',#54140,15.81);
#23084=VERTEX_POINT('',#77418);
#23085=VERTEX_POINT('',#77419);
#23086=VERTEX_POINT('',#77423);
#23087=VERTEX_POINT('',#77425);
#23088=VERTEX_POINT('',#77427);
#23089=VERTEX_POINT('',#77429);
#23090=VERTEX_POINT('',#77435);
#23091=VERTEX_POINT('',#77436);
#23092=VERTEX_POINT('',#77440);
#23093=VERTEX_POINT('',#77442);
#23094=VERTEX_POINT('',#77446);
#23095=VERTEX_POINT('',#77448);
#23096=VERTEX_POINT('',#77455);
#23097=VERTEX_POINT('',#77457);
#23098=VERTEX_POINT('',#77461);
#23099=VERTEX_POINT('',#77463);
#23100=VERTEX_POINT('',#77467);
#23101=VERTEX_POINT('',#77469);
#23102=VERTEX_POINT('',#77473);
#23103=VERTEX_POINT('',#77477);
#23104=VERTEX_POINT('',#77481);
#23105=VERTEX_POINT('',#77483);
#23106=VERTEX_POINT('',#77487);
#23107=VERTEX_POINT('',#77491);
#23108=VERTEX_POINT('',#77495);
#23109=VERTEX_POINT('',#77497);
#23110=VERTEX_POINT('',#77501);
#23111=VERTEX_POINT('',#77505);
#23112=VERTEX_POINT('',#77509);
#23113=VERTEX_POINT('',#77511);
#23114=VERTEX_POINT('',#77515);
#23115=VERTEX_POINT('',#77519);
#23116=VERTEX_POINT('',#77523);
#23117=VERTEX_POINT('',#77525);
#23118=VERTEX_POINT('',#77529);
#23119=VERTEX_POINT('',#77533);
#23120=VERTEX_POINT('',#77537);
#23121=VERTEX_POINT('',#77539);
#23122=VERTEX_POINT('',#77543);
#23123=VERTEX_POINT('',#77547);
#23124=VERTEX_POINT('',#77551);
#23125=VERTEX_POINT('',#77553);
#23126=VERTEX_POINT('',#77557);
#23127=VERTEX_POINT('',#77561);
#23128=VERTEX_POINT('',#77565);
#23129=VERTEX_POINT('',#77567);
#23130=VERTEX_POINT('',#77571);
#23131=VERTEX_POINT('',#77575);
#23132=VERTEX_POINT('',#77579);
#23133=VERTEX_POINT('',#77581);
#23134=VERTEX_POINT('',#77585);
#23135=VERTEX_POINT('',#77589);
#23136=VERTEX_POINT('',#77593);
#23137=VERTEX_POINT('',#77595);
#23138=VERTEX_POINT('',#77599);
#23139=VERTEX_POINT('',#77603);
#23140=VERTEX_POINT('',#77607);
#23141=VERTEX_POINT('',#77609);
#23142=VERTEX_POINT('',#77613);
#23143=VERTEX_POINT('',#77617);
#23144=VERTEX_POINT('',#77623);
#23145=VERTEX_POINT('',#77625);
#23146=VERTEX_POINT('',#77627);
#23147=VERTEX_POINT('',#77629);
#23148=VERTEX_POINT('',#77631);
#23149=VERTEX_POINT('',#77633);
#23150=VERTEX_POINT('',#77635);
#23151=VERTEX_POINT('',#77637);
#23152=VERTEX_POINT('',#77640);
#23153=VERTEX_POINT('',#77643);
#23154=VERTEX_POINT('',#77645);
#23155=VERTEX_POINT('',#77649);
#23156=VERTEX_POINT('',#77653);
#23157=VERTEX_POINT('',#77657);
#23158=VERTEX_POINT('',#77659);
#23159=VERTEX_POINT('',#77663);
#23160=VERTEX_POINT('',#77667);
#23161=VERTEX_POINT('',#77671);
#23162=VERTEX_POINT('',#77673);
#23163=VERTEX_POINT('',#77677);
#23164=VERTEX_POINT('',#77681);
#23165=VERTEX_POINT('',#77685);
#23166=VERTEX_POINT('',#77687);
#23167=VERTEX_POINT('',#77691);
#23168=VERTEX_POINT('',#77695);
#23169=VERTEX_POINT('',#77699);
#23170=VERTEX_POINT('',#77701);
#23171=VERTEX_POINT('',#77705);
#23172=VERTEX_POINT('',#77709);
#23173=VERTEX_POINT('',#77713);
#23174=VERTEX_POINT('',#77715);
#23175=VERTEX_POINT('',#77719);
#23176=VERTEX_POINT('',#77723);
#23177=VERTEX_POINT('',#77727);
#23178=VERTEX_POINT('',#77729);
#23179=VERTEX_POINT('',#77733);
#23180=VERTEX_POINT('',#77737);
#23181=VERTEX_POINT('',#77741);
#23182=VERTEX_POINT('',#77743);
#23183=VERTEX_POINT('',#77747);
#23184=VERTEX_POINT('',#77751);
#23185=VERTEX_POINT('',#77755);
#23186=VERTEX_POINT('',#77757);
#23187=VERTEX_POINT('',#77761);
#23188=VERTEX_POINT('',#77765);
#23189=VERTEX_POINT('',#77769);
#23190=VERTEX_POINT('',#77771);
#23191=VERTEX_POINT('',#77775);
#23192=VERTEX_POINT('',#77779);
#23193=VERTEX_POINT('',#77783);
#23194=VERTEX_POINT('',#77785);
#23195=VERTEX_POINT('',#77789);
#23196=VERTEX_POINT('',#77793);
#23197=VERTEX_POINT('',#77797);
#23198=VERTEX_POINT('',#77803);
#23199=VERTEX_POINT('',#77807);
#23200=VERTEX_POINT('',#77809);
#23201=VERTEX_POINT('',#77813);
#23202=VERTEX_POINT('',#77817);
#23203=VERTEX_POINT('',#77821);
#23204=VERTEX_POINT('',#77823);
#23205=VERTEX_POINT('',#77827);
#23206=VERTEX_POINT('',#77831);
#23207=VERTEX_POINT('',#77835);
#23208=VERTEX_POINT('',#77837);
#23209=VERTEX_POINT('',#77841);
#23210=VERTEX_POINT('',#77845);
#23211=VERTEX_POINT('',#77849);
#23212=VERTEX_POINT('',#77851);
#23213=VERTEX_POINT('',#77855);
#23214=VERTEX_POINT('',#77859);
#23215=VERTEX_POINT('',#77863);
#23216=VERTEX_POINT('',#77865);
#23217=VERTEX_POINT('',#77869);
#23218=VERTEX_POINT('',#77873);
#23219=VERTEX_POINT('',#77877);
#23220=VERTEX_POINT('',#77879);
#23221=VERTEX_POINT('',#77883);
#23222=VERTEX_POINT('',#77887);
#23223=VERTEX_POINT('',#77891);
#23224=VERTEX_POINT('',#77893);
#23225=VERTEX_POINT('',#77897);
#23226=VERTEX_POINT('',#77901);
#23227=VERTEX_POINT('',#77905);
#23228=VERTEX_POINT('',#77907);
#23229=VERTEX_POINT('',#77911);
#23230=VERTEX_POINT('',#77915);
#23231=VERTEX_POINT('',#77919);
#23232=VERTEX_POINT('',#77921);
#23233=VERTEX_POINT('',#77925);
#23234=VERTEX_POINT('',#77929);
#23235=VERTEX_POINT('',#77933);
#23236=VERTEX_POINT('',#77935);
#23237=VERTEX_POINT('',#77939);
#23238=VERTEX_POINT('',#77943);
#23239=VERTEX_POINT('',#77947);
#23240=VERTEX_POINT('',#77949);
#23241=VERTEX_POINT('',#77953);
#23242=VERTEX_POINT('',#77961);
#23243=VERTEX_POINT('',#77966);
#23244=VERTEX_POINT('',#77967);
#23245=VERTEX_POINT('',#77971);
#23246=VERTEX_POINT('',#77976);
#23247=VERTEX_POINT('',#77982);
#23248=VERTEX_POINT('',#77984);
#23249=VERTEX_POINT('',#77988);
#23250=VERTEX_POINT('',#77990);
#23251=VERTEX_POINT('',#77994);
#23252=VERTEX_POINT('',#77998);
#23253=VERTEX_POINT('',#78002);
#23254=VERTEX_POINT('',#78004);
#23255=VERTEX_POINT('',#78008);
#23256=VERTEX_POINT('',#78012);
#23257=VERTEX_POINT('',#78016);
#23258=VERTEX_POINT('',#78018);
#23259=VERTEX_POINT('',#78022);
#23260=VERTEX_POINT('',#78026);
#23261=VERTEX_POINT('',#78030);
#23262=VERTEX_POINT('',#78032);
#23263=VERTEX_POINT('',#78036);
#23264=VERTEX_POINT('',#78040);
#23265=VERTEX_POINT('',#78044);
#23266=VERTEX_POINT('',#78046);
#23267=VERTEX_POINT('',#78050);
#23268=VERTEX_POINT('',#78054);
#23269=VERTEX_POINT('',#78058);
#23270=VERTEX_POINT('',#78060);
#23271=VERTEX_POINT('',#78064);
#23272=VERTEX_POINT('',#78068);
#23273=VERTEX_POINT('',#78072);
#23274=VERTEX_POINT('',#78074);
#23275=VERTEX_POINT('',#78078);
#23276=VERTEX_POINT('',#78082);
#23277=VERTEX_POINT('',#78086);
#23278=VERTEX_POINT('',#78088);
#23279=VERTEX_POINT('',#78092);
#23280=VERTEX_POINT('',#78096);
#23281=VERTEX_POINT('',#78100);
#23282=VERTEX_POINT('',#78102);
#23283=VERTEX_POINT('',#78106);
#23284=VERTEX_POINT('',#78110);
#23285=VERTEX_POINT('',#78114);
#23286=VERTEX_POINT('',#78116);
#23287=VERTEX_POINT('',#78120);
#23288=VERTEX_POINT('',#78124);
#23289=VERTEX_POINT('',#78128);
#23290=VERTEX_POINT('',#78130);
#23291=VERTEX_POINT('',#78134);
#23292=VERTEX_POINT('',#78138);
#23293=VERTEX_POINT('',#78144);
#23294=VERTEX_POINT('',#78148);
#23295=VERTEX_POINT('',#78152);
#23296=VERTEX_POINT('',#78156);
#23297=VERTEX_POINT('',#78158);
#23298=VERTEX_POINT('',#78162);
#23299=VERTEX_POINT('',#78166);
#23300=VERTEX_POINT('',#78170);
#23301=VERTEX_POINT('',#78172);
#23302=VERTEX_POINT('',#78176);
#23303=VERTEX_POINT('',#78180);
#23304=VERTEX_POINT('',#78184);
#23305=VERTEX_POINT('',#78186);
#23306=VERTEX_POINT('',#78190);
#23307=VERTEX_POINT('',#78194);
#23308=VERTEX_POINT('',#78198);
#23309=VERTEX_POINT('',#78200);
#23310=VERTEX_POINT('',#78204);
#23311=VERTEX_POINT('',#78208);
#23312=VERTEX_POINT('',#78212);
#23313=VERTEX_POINT('',#78214);
#23314=VERTEX_POINT('',#78218);
#23315=VERTEX_POINT('',#78222);
#23316=VERTEX_POINT('',#78226);
#23317=VERTEX_POINT('',#78228);
#23318=VERTEX_POINT('',#78232);
#23319=VERTEX_POINT('',#78236);
#23320=VERTEX_POINT('',#78240);
#23321=VERTEX_POINT('',#78242);
#23322=VERTEX_POINT('',#78246);
#23323=VERTEX_POINT('',#78250);
#23324=VERTEX_POINT('',#78254);
#23325=VERTEX_POINT('',#78256);
#23326=VERTEX_POINT('',#78260);
#23327=VERTEX_POINT('',#78264);
#23328=VERTEX_POINT('',#78268);
#23329=VERTEX_POINT('',#78270);
#23330=VERTEX_POINT('',#78274);
#23331=VERTEX_POINT('',#78278);
#23332=VERTEX_POINT('',#78282);
#23333=VERTEX_POINT('',#78284);
#23334=VERTEX_POINT('',#78288);
#23335=VERTEX_POINT('',#78292);
#23336=VERTEX_POINT('',#78296);
#23337=VERTEX_POINT('',#78298);
#23338=VERTEX_POINT('',#78306);
#23339=VERTEX_POINT('',#78308);
#23340=VERTEX_POINT('',#78312);
#23341=VERTEX_POINT('',#78316);
#23342=VERTEX_POINT('',#78320);
#23343=VERTEX_POINT('',#78322);
#23344=VERTEX_POINT('',#78326);
#23345=VERTEX_POINT('',#78330);
#23346=VERTEX_POINT('',#78334);
#23347=VERTEX_POINT('',#78336);
#23348=VERTEX_POINT('',#78340);
#23349=VERTEX_POINT('',#78344);
#23350=VERTEX_POINT('',#78348);
#23351=VERTEX_POINT('',#78350);
#23352=VERTEX_POINT('',#78354);
#23353=VERTEX_POINT('',#78358);
#23354=VERTEX_POINT('',#78362);
#23355=VERTEX_POINT('',#78364);
#23356=VERTEX_POINT('',#78368);
#23357=VERTEX_POINT('',#78372);
#23358=VERTEX_POINT('',#78376);
#23359=VERTEX_POINT('',#78378);
#23360=VERTEX_POINT('',#78382);
#23361=VERTEX_POINT('',#78386);
#23362=VERTEX_POINT('',#78390);
#23363=VERTEX_POINT('',#78392);
#23364=VERTEX_POINT('',#78396);
#23365=VERTEX_POINT('',#78400);
#23366=VERTEX_POINT('',#78404);
#23367=VERTEX_POINT('',#78406);
#23368=VERTEX_POINT('',#78410);
#23369=VERTEX_POINT('',#78414);
#23370=VERTEX_POINT('',#78418);
#23371=VERTEX_POINT('',#78420);
#23372=VERTEX_POINT('',#78424);
#23373=VERTEX_POINT('',#78428);
#23374=VERTEX_POINT('',#78432);
#23375=VERTEX_POINT('',#78434);
#23376=VERTEX_POINT('',#78438);
#23377=VERTEX_POINT('',#78442);
#23378=VERTEX_POINT('',#78446);
#23379=VERTEX_POINT('',#78448);
#23380=VERTEX_POINT('',#78452);
#23381=VERTEX_POINT('',#78456);
#23382=VERTEX_POINT('',#78460);
#23383=VERTEX_POINT('',#78466);
#23384=VERTEX_POINT('',#78472);
#23385=VERTEX_POINT('',#78480);
#23386=VERTEX_POINT('',#78481);
#23387=VERTEX_POINT('',#78485);
#23388=VERTEX_POINT('',#78489);
#23389=VERTEX_POINT('',#78495);
#23390=VERTEX_POINT('',#78496);
#23391=VERTEX_POINT('',#78500);
#23392=VERTEX_POINT('',#78504);
#23393=VERTEX_POINT('',#78510);
#23394=VERTEX_POINT('',#78511);
#23395=VERTEX_POINT('',#78515);
#23396=VERTEX_POINT('',#78519);
#23397=VERTEX_POINT('',#78525);
#23398=VERTEX_POINT('',#78526);
#23399=VERTEX_POINT('',#78530);
#23400=VERTEX_POINT('',#78534);
#23401=VERTEX_POINT('',#78540);
#23402=VERTEX_POINT('',#78541);
#23403=VERTEX_POINT('',#78545);
#23404=VERTEX_POINT('',#78549);
#23405=VERTEX_POINT('',#78555);
#23406=VERTEX_POINT('',#78556);
#23407=VERTEX_POINT('',#78560);
#23408=VERTEX_POINT('',#78564);
#23409=VERTEX_POINT('',#78570);
#23410=VERTEX_POINT('',#78571);
#23411=VERTEX_POINT('',#78575);
#23412=VERTEX_POINT('',#78579);
#23413=VERTEX_POINT('',#78585);
#23414=VERTEX_POINT('',#78586);
#23415=VERTEX_POINT('',#78590);
#23416=VERTEX_POINT('',#78594);
#23417=VERTEX_POINT('',#78600);
#23418=VERTEX_POINT('',#78601);
#23419=VERTEX_POINT('',#78605);
#23420=VERTEX_POINT('',#78609);
#23421=VERTEX_POINT('',#78615);
#23422=VERTEX_POINT('',#78616);
#23423=VERTEX_POINT('',#78620);
#23424=VERTEX_POINT('',#78624);
#23425=VERTEX_POINT('',#78630);
#23426=VERTEX_POINT('',#78631);
#23427=VERTEX_POINT('',#78635);
#23428=VERTEX_POINT('',#78639);
#23429=VERTEX_POINT('',#78645);
#23430=VERTEX_POINT('',#78646);
#23431=VERTEX_POINT('',#78650);
#23432=VERTEX_POINT('',#78654);
#23433=VERTEX_POINT('',#78660);
#23434=VERTEX_POINT('',#78661);
#23435=VERTEX_POINT('',#78665);
#23436=VERTEX_POINT('',#78669);
#23437=VERTEX_POINT('',#78675);
#23438=VERTEX_POINT('',#78676);
#23439=VERTEX_POINT('',#78680);
#23440=VERTEX_POINT('',#78684);
#23441=VERTEX_POINT('',#78690);
#23442=VERTEX_POINT('',#78691);
#23443=VERTEX_POINT('',#78695);
#23444=VERTEX_POINT('',#78699);
#23445=VERTEX_POINT('',#78705);
#23446=VERTEX_POINT('',#78706);
#23447=VERTEX_POINT('',#78710);
#23448=VERTEX_POINT('',#78714);
#23449=VERTEX_POINT('',#78720);
#23450=VERTEX_POINT('',#78721);
#23451=VERTEX_POINT('',#78725);
#23452=VERTEX_POINT('',#78729);
#23453=VERTEX_POINT('',#78735);
#23454=VERTEX_POINT('',#78736);
#23455=VERTEX_POINT('',#78740);
#23456=VERTEX_POINT('',#78744);
#23457=VERTEX_POINT('',#78750);
#23458=VERTEX_POINT('',#78751);
#23459=VERTEX_POINT('',#78755);
#23460=VERTEX_POINT('',#78759);
#23461=VERTEX_POINT('',#78765);
#23462=VERTEX_POINT('',#78766);
#23463=VERTEX_POINT('',#78770);
#23464=VERTEX_POINT('',#78774);
#23465=VERTEX_POINT('',#78780);
#23466=VERTEX_POINT('',#78781);
#23467=VERTEX_POINT('',#78785);
#23468=VERTEX_POINT('',#78789);
#23469=VERTEX_POINT('',#78795);
#23470=VERTEX_POINT('',#78796);
#23471=VERTEX_POINT('',#78800);
#23472=VERTEX_POINT('',#78804);
#23473=VERTEX_POINT('',#78810);
#23474=VERTEX_POINT('',#78811);
#23475=VERTEX_POINT('',#78815);
#23476=VERTEX_POINT('',#78819);
#23477=VERTEX_POINT('',#78825);
#23478=VERTEX_POINT('',#78826);
#23479=VERTEX_POINT('',#78830);
#23480=VERTEX_POINT('',#78834);
#23481=VERTEX_POINT('',#78840);
#23482=VERTEX_POINT('',#78841);
#23483=VERTEX_POINT('',#78845);
#23484=VERTEX_POINT('',#78849);
#23485=VERTEX_POINT('',#78855);
#23486=VERTEX_POINT('',#78856);
#23487=VERTEX_POINT('',#78860);
#23488=VERTEX_POINT('',#78864);
#23489=VERTEX_POINT('',#78870);
#23490=VERTEX_POINT('',#78871);
#23491=VERTEX_POINT('',#78875);
#23492=VERTEX_POINT('',#78879);
#23493=VERTEX_POINT('',#78885);
#23494=VERTEX_POINT('',#78886);
#23495=VERTEX_POINT('',#78890);
#23496=VERTEX_POINT('',#78894);
#23497=VERTEX_POINT('',#78900);
#23498=VERTEX_POINT('',#78901);
#23499=VERTEX_POINT('',#78905);
#23500=VERTEX_POINT('',#78909);
#23501=VERTEX_POINT('',#78915);
#23502=VERTEX_POINT('',#78916);
#23503=VERTEX_POINT('',#78920);
#23504=VERTEX_POINT('',#78924);
#23505=VERTEX_POINT('',#78930);
#23506=VERTEX_POINT('',#78931);
#23507=VERTEX_POINT('',#78935);
#23508=VERTEX_POINT('',#78939);
#23509=VERTEX_POINT('',#78945);
#23510=VERTEX_POINT('',#78946);
#23511=VERTEX_POINT('',#78950);
#23512=VERTEX_POINT('',#78954);
#23513=VERTEX_POINT('',#78960);
#23514=VERTEX_POINT('',#78961);
#23515=VERTEX_POINT('',#78965);
#23516=VERTEX_POINT('',#78969);
#23517=VERTEX_POINT('',#78975);
#23518=VERTEX_POINT('',#78977);
#23519=VERTEX_POINT('',#78981);
#23520=VERTEX_POINT('',#78985);
#23521=VERTEX_POINT('',#78989);
#23522=VERTEX_POINT('',#78995);
#23523=VERTEX_POINT('',#78997);
#23524=VERTEX_POINT('',#79001);
#23525=VERTEX_POINT('',#79005);
#23526=VERTEX_POINT('',#79009);
#23527=VERTEX_POINT('',#79015);
#23528=VERTEX_POINT('',#79017);
#23529=VERTEX_POINT('',#79021);
#23530=VERTEX_POINT('',#79025);
#23531=VERTEX_POINT('',#79029);
#23532=VERTEX_POINT('',#79035);
#23533=VERTEX_POINT('',#79037);
#23534=VERTEX_POINT('',#79041);
#23535=VERTEX_POINT('',#79045);
#23536=VERTEX_POINT('',#79049);
#23537=VERTEX_POINT('',#79055);
#23538=VERTEX_POINT('',#79057);
#23539=VERTEX_POINT('',#79061);
#23540=VERTEX_POINT('',#79065);
#23541=VERTEX_POINT('',#79069);
#23542=VERTEX_POINT('',#79075);
#23543=VERTEX_POINT('',#79077);
#23544=VERTEX_POINT('',#79081);
#23545=VERTEX_POINT('',#79085);
#23546=VERTEX_POINT('',#79089);
#23547=VERTEX_POINT('',#79095);
#23548=VERTEX_POINT('',#79097);
#23549=VERTEX_POINT('',#79101);
#23550=VERTEX_POINT('',#79105);
#23551=VERTEX_POINT('',#79109);
#23552=VERTEX_POINT('',#79115);
#23553=VERTEX_POINT('',#79117);
#23554=VERTEX_POINT('',#79121);
#23555=VERTEX_POINT('',#79125);
#23556=VERTEX_POINT('',#79129);
#23557=VERTEX_POINT('',#79135);
#23558=VERTEX_POINT('',#79137);
#23559=VERTEX_POINT('',#79141);
#23560=VERTEX_POINT('',#79145);
#23561=VERTEX_POINT('',#79149);
#23562=VERTEX_POINT('',#79155);
#23563=VERTEX_POINT('',#79157);
#23564=VERTEX_POINT('',#79161);
#23565=VERTEX_POINT('',#79165);
#23566=VERTEX_POINT('',#79169);
#23567=VERTEX_POINT('',#79175);
#23568=VERTEX_POINT('',#79177);
#23569=VERTEX_POINT('',#79181);
#23570=VERTEX_POINT('',#79185);
#23571=VERTEX_POINT('',#79189);
#23572=VERTEX_POINT('',#79195);
#23573=VERTEX_POINT('',#79197);
#23574=VERTEX_POINT('',#79201);
#23575=VERTEX_POINT('',#79205);
#23576=VERTEX_POINT('',#79209);
#23577=VERTEX_POINT('',#79215);
#23578=VERTEX_POINT('',#79217);
#23579=VERTEX_POINT('',#79221);
#23580=VERTEX_POINT('',#79225);
#23581=VERTEX_POINT('',#79229);
#23582=VERTEX_POINT('',#79235);
#23583=VERTEX_POINT('',#79237);
#23584=VERTEX_POINT('',#79241);
#23585=VERTEX_POINT('',#79245);
#23586=VERTEX_POINT('',#79249);
#23587=VERTEX_POINT('',#79255);
#23588=VERTEX_POINT('',#79257);
#23589=VERTEX_POINT('',#79261);
#23590=VERTEX_POINT('',#79265);
#23591=VERTEX_POINT('',#79269);
#23592=VERTEX_POINT('',#79275);
#23593=VERTEX_POINT('',#79277);
#23594=VERTEX_POINT('',#79281);
#23595=VERTEX_POINT('',#79285);
#23596=VERTEX_POINT('',#79289);
#23597=VERTEX_POINT('',#79295);
#23598=VERTEX_POINT('',#79297);
#23599=VERTEX_POINT('',#79301);
#23600=VERTEX_POINT('',#79305);
#23601=VERTEX_POINT('',#79309);
#23602=VERTEX_POINT('',#79315);
#23603=VERTEX_POINT('',#79317);
#23604=VERTEX_POINT('',#79321);
#23605=VERTEX_POINT('',#79325);
#23606=VERTEX_POINT('',#79329);
#23607=VERTEX_POINT('',#79335);
#23608=VERTEX_POINT('',#79337);
#23609=VERTEX_POINT('',#79341);
#23610=VERTEX_POINT('',#79345);
#23611=VERTEX_POINT('',#79349);
#23612=VERTEX_POINT('',#79355);
#23613=VERTEX_POINT('',#79357);
#23614=VERTEX_POINT('',#79361);
#23615=VERTEX_POINT('',#79365);
#23616=VERTEX_POINT('',#79369);
#23617=VERTEX_POINT('',#79375);
#23618=VERTEX_POINT('',#79377);
#23619=VERTEX_POINT('',#79381);
#23620=VERTEX_POINT('',#79385);
#23621=VERTEX_POINT('',#79389);
#23622=VERTEX_POINT('',#79395);
#23623=VERTEX_POINT('',#79397);
#23624=VERTEX_POINT('',#79401);
#23625=VERTEX_POINT('',#79405);
#23626=VERTEX_POINT('',#79409);
#23627=VERTEX_POINT('',#79415);
#23628=VERTEX_POINT('',#79417);
#23629=VERTEX_POINT('',#79421);
#23630=VERTEX_POINT('',#79425);
#23631=VERTEX_POINT('',#79429);
#23632=VERTEX_POINT('',#79435);
#23633=VERTEX_POINT('',#79437);
#23634=VERTEX_POINT('',#79441);
#23635=VERTEX_POINT('',#79445);
#23636=VERTEX_POINT('',#79449);
#23637=VERTEX_POINT('',#79455);
#23638=VERTEX_POINT('',#79457);
#23639=VERTEX_POINT('',#79461);
#23640=VERTEX_POINT('',#79465);
#23641=VERTEX_POINT('',#79469);
#23642=VERTEX_POINT('',#79475);
#23643=VERTEX_POINT('',#79477);
#23644=VERTEX_POINT('',#79481);
#23645=VERTEX_POINT('',#79485);
#23646=VERTEX_POINT('',#79489);
#23647=VERTEX_POINT('',#79495);
#23648=VERTEX_POINT('',#79497);
#23649=VERTEX_POINT('',#79501);
#23650=VERTEX_POINT('',#79505);
#23651=VERTEX_POINT('',#79509);
#23652=VERTEX_POINT('',#79515);
#23653=VERTEX_POINT('',#79517);
#23654=VERTEX_POINT('',#79521);
#23655=VERTEX_POINT('',#79525);
#23656=VERTEX_POINT('',#79529);
#23657=VERTEX_POINT('',#79535);
#23658=VERTEX_POINT('',#79537);
#23659=VERTEX_POINT('',#79541);
#23660=VERTEX_POINT('',#79545);
#23661=VERTEX_POINT('',#79549);
#23662=VERTEX_POINT('',#79555);
#23663=VERTEX_POINT('',#79557);
#23664=VERTEX_POINT('',#79561);
#23665=VERTEX_POINT('',#79565);
#23666=VERTEX_POINT('',#79569);
#23667=VERTEX_POINT('',#79575);
#23668=VERTEX_POINT('',#79577);
#23669=VERTEX_POINT('',#79581);
#23670=VERTEX_POINT('',#79585);
#23671=VERTEX_POINT('',#79589);
#23672=VERTEX_POINT('',#79595);
#23673=VERTEX_POINT('',#79597);
#23674=VERTEX_POINT('',#79601);
#23675=VERTEX_POINT('',#79605);
#23676=VERTEX_POINT('',#79609);
#23677=VERTEX_POINT('',#79615);
#23678=VERTEX_POINT('',#79617);
#23679=VERTEX_POINT('',#79621);
#23680=VERTEX_POINT('',#79625);
#23681=VERTEX_POINT('',#79629);
#23682=VERTEX_POINT('',#79635);
#23683=VERTEX_POINT('',#79641);
#23684=VERTEX_POINT('',#79647);
#23685=VERTEX_POINT('',#79653);
#23686=VERTEX_POINT('',#79659);
#23687=VERTEX_POINT('',#79665);
#23688=VERTEX_POINT('',#79671);
#23689=VERTEX_POINT('',#79677);
#23690=VERTEX_POINT('',#79683);
#23691=VERTEX_POINT('',#79689);
#23692=VERTEX_POINT('',#79695);
#23693=VERTEX_POINT('',#79701);
#23694=VERTEX_POINT('',#79707);
#23695=VERTEX_POINT('',#79713);
#23696=VERTEX_POINT('',#79719);
#23697=VERTEX_POINT('',#79725);
#23698=VERTEX_POINT('',#79731);
#23699=VERTEX_POINT('',#79737);
#23700=VERTEX_POINT('',#79743);
#23701=VERTEX_POINT('',#79749);
#23702=VERTEX_POINT('',#79755);
#23703=VERTEX_POINT('',#79761);
#23704=VERTEX_POINT('',#79767);
#23705=VERTEX_POINT('',#79773);
#23706=VERTEX_POINT('',#79779);
#23707=VERTEX_POINT('',#79785);
#23708=VERTEX_POINT('',#79791);
#23709=VERTEX_POINT('',#79797);
#23710=VERTEX_POINT('',#79803);
#23711=VERTEX_POINT('',#79809);
#23712=VERTEX_POINT('',#79815);
#23713=VERTEX_POINT('',#79821);
#23714=VERTEX_POINT('',#79827);
#23715=VERTEX_POINT('',#79833);
#23716=VERTEX_POINT('',#79837);
#23717=VERTEX_POINT('',#79841);
#23718=VERTEX_POINT('',#79845);
#23719=VERTEX_POINT('',#79849);
#23720=VERTEX_POINT('',#79853);
#23721=VERTEX_POINT('',#79857);
#23722=VERTEX_POINT('',#79861);
#23723=VERTEX_POINT('',#79865);
#23724=VERTEX_POINT('',#79869);
#23725=VERTEX_POINT('',#79873);
#23726=VERTEX_POINT('',#79877);
#23727=VERTEX_POINT('',#79881);
#23728=VERTEX_POINT('',#79885);
#23729=VERTEX_POINT('',#79889);
#23730=VERTEX_POINT('',#79893);
#23731=VERTEX_POINT('',#79897);
#23732=VERTEX_POINT('',#79901);
#23733=VERTEX_POINT('',#79905);
#23734=VERTEX_POINT('',#79909);
#23735=VERTEX_POINT('',#79913);
#23736=VERTEX_POINT('',#79916);
#23737=VERTEX_POINT('',#79920);
#23738=VERTEX_POINT('',#79924);
#23739=VERTEX_POINT('',#79928);
#23740=VERTEX_POINT('',#79932);
#23741=VERTEX_POINT('',#79936);
#23742=VERTEX_POINT('',#79940);
#23743=VERTEX_POINT('',#79944);
#23744=VERTEX_POINT('',#79948);
#23745=VERTEX_POINT('',#79952);
#23746=VERTEX_POINT('',#79956);
#23747=VERTEX_POINT('',#79960);
#23748=VERTEX_POINT('',#79964);
#23749=VERTEX_POINT('',#79968);
#23750=VERTEX_POINT('',#79972);
#23751=VERTEX_POINT('',#79976);
#23752=VERTEX_POINT('',#79980);
#23753=VERTEX_POINT('',#79984);
#23754=VERTEX_POINT('',#79988);
#23755=VERTEX_POINT('',#79992);
#23756=VERTEX_POINT('',#79996);
#23757=VERTEX_POINT('',#80000);
#23758=VERTEX_POINT('',#80003);
#23759=VERTEX_POINT('',#80007);
#23760=VERTEX_POINT('',#80011);
#23761=VERTEX_POINT('',#80015);
#23762=VERTEX_POINT('',#80019);
#23763=VERTEX_POINT('',#80023);
#23764=VERTEX_POINT('',#80027);
#23765=VERTEX_POINT('',#80031);
#23766=VERTEX_POINT('',#80035);
#23767=VERTEX_POINT('',#80039);
#23768=VERTEX_POINT('',#80043);
#23769=VERTEX_POINT('',#80047);
#23770=VERTEX_POINT('',#80051);
#23771=VERTEX_POINT('',#80055);
#23772=VERTEX_POINT('',#80059);
#23773=VERTEX_POINT('',#80063);
#23774=VERTEX_POINT('',#80067);
#23775=VERTEX_POINT('',#80071);
#23776=VERTEX_POINT('',#80075);
#23777=VERTEX_POINT('',#80079);
#23778=VERTEX_POINT('',#80083);
#23779=VERTEX_POINT('',#80087);
#23780=VERTEX_POINT('',#80090);
#23781=VERTEX_POINT('',#80325);
#23782=VERTEX_POINT('',#80326);
#23783=VERTEX_POINT('',#80328);
#23784=VERTEX_POINT('',#80333);
#23785=VERTEX_POINT('',#80336);
#23786=VERTEX_POINT('',#80340);
#23787=VERTEX_POINT('',#80342);
#23788=VERTEX_POINT('',#80344);
#23789=VERTEX_POINT('',#80348);
#23790=VERTEX_POINT('',#80353);
#23791=VERTEX_POINT('',#80355);
#23792=VERTEX_POINT('',#80359);
#23793=VERTEX_POINT('',#80363);
#23794=VERTEX_POINT('',#80364);
#23795=VERTEX_POINT('',#80369);
#23796=VERTEX_POINT('',#80373);
#23797=VERTEX_POINT('',#80375);
#23798=VERTEX_POINT('',#80379);
#23799=VERTEX_POINT('',#80385);
#29463=EDGE_CURVE('',#23084,#23085,#19132,.T.);
#29464=EDGE_CURVE('',#23086,#23084,#4835,.T.);
#29465=EDGE_CURVE('',#23087,#23086,#4836,.T.);
#29466=EDGE_CURVE('',#23088,#23087,#4837,.T.);
#29467=EDGE_CURVE('',#23089,#23088,#19133,.T.);
#29468=EDGE_CURVE('',#23085,#23089,#4838,.T.);
#29469=EDGE_CURVE('',#23090,#23091,#19134,.T.);
#29470=EDGE_CURVE('',#23092,#23090,#4839,.T.);
#29471=EDGE_CURVE('',#23093,#23092,#19135,.T.);
#29472=EDGE_CURVE('',#23094,#23093,#4840,.T.);
#29473=EDGE_CURVE('',#23094,#23095,#4841,.T.);
#29474=EDGE_CURVE('',#23091,#23095,#4842,.T.);
#29475=EDGE_CURVE('',#23087,#23094,#4843,.T.);
#29476=EDGE_CURVE('',#23095,#23086,#4844,.T.);
#29477=EDGE_CURVE('',#23089,#23096,#19743,.T.);
#29478=EDGE_CURVE('',#23096,#23097,#4845,.T.);
#29479=EDGE_CURVE('',#23085,#23097,#19744,.T.);
#29480=EDGE_CURVE('',#23098,#23091,#19745,.T.);
#29481=EDGE_CURVE('',#23098,#23099,#19136,.T.);
#29482=EDGE_CURVE('',#23099,#23100,#19746,.T.);
#29483=EDGE_CURVE('',#23100,#23101,#19137,.T.);
#29484=EDGE_CURVE('',#23101,#23102,#19138,.T.);
#29485=EDGE_CURVE('',#23102,#23103,#19139,.T.);
#29486=EDGE_CURVE('',#23103,#23104,#19747,.T.);
#29487=EDGE_CURVE('',#23104,#23105,#19140,.T.);
#29488=EDGE_CURVE('',#23105,#23106,#19141,.T.);
#29489=EDGE_CURVE('',#23106,#23107,#19142,.T.);
#29490=EDGE_CURVE('',#23107,#23108,#19748,.T.);
#29491=EDGE_CURVE('',#23108,#23109,#19143,.T.);
#29492=EDGE_CURVE('',#23109,#23110,#19144,.T.);
#29493=EDGE_CURVE('',#23110,#23111,#19145,.T.);
#29494=EDGE_CURVE('',#23111,#23112,#19749,.T.);
#29495=EDGE_CURVE('',#23112,#23113,#19146,.T.);
#29496=EDGE_CURVE('',#23113,#23114,#19147,.T.);
#29497=EDGE_CURVE('',#23114,#23115,#19148,.T.);
#29498=EDGE_CURVE('',#23115,#23116,#19750,.T.);
#29499=EDGE_CURVE('',#23116,#23117,#19149,.T.);
#29500=EDGE_CURVE('',#23117,#23118,#19150,.T.);
#29501=EDGE_CURVE('',#23118,#23119,#19151,.T.);
#29502=EDGE_CURVE('',#23119,#23120,#19751,.T.);
#29503=EDGE_CURVE('',#23120,#23121,#19152,.T.);
#29504=EDGE_CURVE('',#23121,#23122,#19153,.T.);
#29505=EDGE_CURVE('',#23122,#23123,#19154,.T.);
#29506=EDGE_CURVE('',#23123,#23124,#19752,.T.);
#29507=EDGE_CURVE('',#23124,#23125,#19155,.T.);
#29508=EDGE_CURVE('',#23125,#23126,#19156,.T.);
#29509=EDGE_CURVE('',#23126,#23127,#19157,.T.);
#29510=EDGE_CURVE('',#23127,#23128,#19753,.T.);
#29511=EDGE_CURVE('',#23128,#23129,#19158,.T.);
#29512=EDGE_CURVE('',#23129,#23130,#19159,.T.);
#29513=EDGE_CURVE('',#23130,#23131,#19160,.T.);
#29514=EDGE_CURVE('',#23131,#23132,#19754,.T.);
#29515=EDGE_CURVE('',#23132,#23133,#19161,.T.);
#29516=EDGE_CURVE('',#23133,#23134,#19162,.T.);
#29517=EDGE_CURVE('',#23134,#23135,#19163,.T.);
#29518=EDGE_CURVE('',#23135,#23136,#19755,.T.);
#29519=EDGE_CURVE('',#23136,#23137,#19164,.T.);
#29520=EDGE_CURVE('',#23137,#23138,#19165,.T.);
#29521=EDGE_CURVE('',#23138,#23139,#19166,.T.);
#29522=EDGE_CURVE('',#23139,#23140,#19756,.T.);
#29523=EDGE_CURVE('',#23140,#23141,#19167,.T.);
#29524=EDGE_CURVE('',#23141,#23142,#19168,.T.);
#29525=EDGE_CURVE('',#23142,#23143,#19169,.T.);
#29526=EDGE_CURVE('',#23143,#23090,#19757,.T.);
#29527=EDGE_CURVE('',#23144,#23093,#19758,.T.);
#29528=EDGE_CURVE('',#23144,#23145,#4846,.T.);
#29529=EDGE_CURVE('',#23145,#23146,#4847,.T.);
#29530=EDGE_CURVE('',#23146,#23147,#4848,.T.);
#29531=EDGE_CURVE('',#23148,#23147,#19759,.T.);
#29532=EDGE_CURVE('',#23148,#23149,#4849,.T.);
#29533=EDGE_CURVE('',#23149,#23150,#4850,.T.);
#29534=EDGE_CURVE('',#23150,#23151,#4851,.T.);
#29535=EDGE_CURVE('',#23088,#23151,#19760,.T.);
#29536=EDGE_CURVE('',#23152,#23152,#19761,.T.);
#29537=EDGE_CURVE('',#23153,#23092,#19762,.T.);
#29538=EDGE_CURVE('',#23153,#23154,#19170,.T.);
#29539=EDGE_CURVE('',#23154,#23155,#19171,.T.);
#29540=EDGE_CURVE('',#23155,#23156,#19172,.T.);
#29541=EDGE_CURVE('',#23157,#23156,#19763,.T.);
#29542=EDGE_CURVE('',#23157,#23158,#19173,.T.);
#29543=EDGE_CURVE('',#23158,#23159,#19174,.T.);
#29544=EDGE_CURVE('',#23159,#23160,#19175,.T.);
#29545=EDGE_CURVE('',#23161,#23160,#19764,.T.);
#29546=EDGE_CURVE('',#23161,#23162,#19176,.T.);
#29547=EDGE_CURVE('',#23162,#23163,#19177,.T.);
#29548=EDGE_CURVE('',#23163,#23164,#19178,.T.);
#29549=EDGE_CURVE('',#23165,#23164,#19765,.T.);
#29550=EDGE_CURVE('',#23165,#23166,#19179,.T.);
#29551=EDGE_CURVE('',#23166,#23167,#19180,.T.);
#29552=EDGE_CURVE('',#23167,#23168,#19181,.T.);
#29553=EDGE_CURVE('',#23169,#23168,#19766,.T.);
#29554=EDGE_CURVE('',#23169,#23170,#19182,.T.);
#29555=EDGE_CURVE('',#23170,#23171,#19183,.T.);
#29556=EDGE_CURVE('',#23171,#23172,#19184,.T.);
#29557=EDGE_CURVE('',#23173,#23172,#19767,.T.);
#29558=EDGE_CURVE('',#23173,#23174,#19185,.T.);
#29559=EDGE_CURVE('',#23174,#23175,#19186,.T.);
#29560=EDGE_CURVE('',#23175,#23176,#19187,.T.);
#29561=EDGE_CURVE('',#23177,#23176,#19768,.T.);
#29562=EDGE_CURVE('',#23177,#23178,#19188,.T.);
#29563=EDGE_CURVE('',#23178,#23179,#19189,.T.);
#29564=EDGE_CURVE('',#23179,#23180,#19190,.T.);
#29565=EDGE_CURVE('',#23181,#23180,#19769,.T.);
#29566=EDGE_CURVE('',#23181,#23182,#19191,.T.);
#29567=EDGE_CURVE('',#23182,#23183,#19192,.T.);
#29568=EDGE_CURVE('',#23183,#23184,#19193,.T.);
#29569=EDGE_CURVE('',#23185,#23184,#19770,.T.);
#29570=EDGE_CURVE('',#23185,#23186,#19194,.T.);
#29571=EDGE_CURVE('',#23186,#23187,#19195,.T.);
#29572=EDGE_CURVE('',#23187,#23188,#19196,.T.);
#29573=EDGE_CURVE('',#23189,#23188,#19771,.T.);
#29574=EDGE_CURVE('',#23189,#23190,#19197,.T.);
#29575=EDGE_CURVE('',#23190,#23191,#19198,.T.);
#29576=EDGE_CURVE('',#23191,#23192,#19199,.T.);
#29577=EDGE_CURVE('',#23193,#23192,#19772,.T.);
#29578=EDGE_CURVE('',#23193,#23194,#19200,.T.);
#29579=EDGE_CURVE('',#23194,#23195,#19201,.T.);
#29580=EDGE_CURVE('',#23195,#23196,#19202,.T.);
#29581=EDGE_CURVE('',#23197,#23196,#19773,.T.);
#29582=EDGE_CURVE('',#23197,#23144,#19203,.T.);
#29583=EDGE_CURVE('',#23151,#23198,#19204,.T.);
#29584=EDGE_CURVE('',#23199,#23198,#19774,.T.);
#29585=EDGE_CURVE('',#23199,#23200,#19205,.T.);
#29586=EDGE_CURVE('',#23200,#23201,#19206,.T.);
#29587=EDGE_CURVE('',#23201,#23202,#19207,.T.);
#29588=EDGE_CURVE('',#23203,#23202,#19775,.T.);
#29589=EDGE_CURVE('',#23203,#23204,#19208,.T.);
#29590=EDGE_CURVE('',#23204,#23205,#19209,.T.);
#29591=EDGE_CURVE('',#23205,#23206,#19210,.T.);
#29592=EDGE_CURVE('',#23207,#23206,#19776,.T.);
#29593=EDGE_CURVE('',#23207,#23208,#19211,.T.);
#29594=EDGE_CURVE('',#23208,#23209,#19212,.T.);
#29595=EDGE_CURVE('',#23209,#23210,#19213,.T.);
#29596=EDGE_CURVE('',#23211,#23210,#19777,.T.);
#29597=EDGE_CURVE('',#23211,#23212,#19214,.T.);
#29598=EDGE_CURVE('',#23212,#23213,#19215,.T.);
#29599=EDGE_CURVE('',#23213,#23214,#19216,.T.);
#29600=EDGE_CURVE('',#23215,#23214,#19778,.T.);
#29601=EDGE_CURVE('',#23215,#23216,#19217,.T.);
#29602=EDGE_CURVE('',#23216,#23217,#19218,.T.);
#29603=EDGE_CURVE('',#23217,#23218,#19219,.T.);
#29604=EDGE_CURVE('',#23219,#23218,#19779,.T.);
#29605=EDGE_CURVE('',#23219,#23220,#19220,.T.);
#29606=EDGE_CURVE('',#23220,#23221,#19221,.T.);
#29607=EDGE_CURVE('',#23221,#23222,#19222,.T.);
#29608=EDGE_CURVE('',#23223,#23222,#19780,.T.);
#29609=EDGE_CURVE('',#23223,#23224,#19223,.T.);
#29610=EDGE_CURVE('',#23224,#23225,#19224,.T.);
#29611=EDGE_CURVE('',#23225,#23226,#19225,.T.);
#29612=EDGE_CURVE('',#23227,#23226,#19781,.T.);
#29613=EDGE_CURVE('',#23227,#23228,#19226,.T.);
#29614=EDGE_CURVE('',#23228,#23229,#19227,.T.);
#29615=EDGE_CURVE('',#23229,#23230,#19228,.T.);
#29616=EDGE_CURVE('',#23231,#23230,#19782,.T.);
#29617=EDGE_CURVE('',#23231,#23232,#19229,.T.);
#29618=EDGE_CURVE('',#23232,#23233,#19230,.T.);
#29619=EDGE_CURVE('',#23233,#23234,#19231,.T.);
#29620=EDGE_CURVE('',#23235,#23234,#19783,.T.);
#29621=EDGE_CURVE('',#23235,#23236,#19232,.T.);
#29622=EDGE_CURVE('',#23236,#23237,#19233,.T.);
#29623=EDGE_CURVE('',#23237,#23238,#19234,.T.);
#29624=EDGE_CURVE('',#23239,#23238,#19784,.T.);
#29625=EDGE_CURVE('',#23239,#23240,#19235,.T.);
#29626=EDGE_CURVE('',#23240,#23241,#19236,.T.);
#29627=EDGE_CURVE('',#23241,#23096,#19237,.T.);
#29628=EDGE_CURVE('',#23242,#23098,#4852,.T.);
#29629=EDGE_CURVE('',#23145,#23242,#4853,.T.);
#29630=EDGE_CURVE('',#23099,#23197,#4854,.T.);
#29631=EDGE_CURVE('',#23243,#23244,#19238,.T.);
#29632=EDGE_CURVE('',#23245,#23243,#4855,.T.);
#29633=EDGE_CURVE('',#23147,#23245,#19239,.T.);
#29634=EDGE_CURVE('',#23146,#23246,#4856,.T.);
#29635=EDGE_CURVE('',#23244,#23246,#4857,.T.);
#29636=EDGE_CURVE('',#23246,#23242,#4858,.T.);
#29637=EDGE_CURVE('',#23247,#23244,#19785,.T.);
#29638=EDGE_CURVE('',#23247,#23248,#19240,.T.);
#29639=EDGE_CURVE('',#23248,#23249,#19786,.T.);
#29640=EDGE_CURVE('',#23249,#23250,#19241,.T.);
#29641=EDGE_CURVE('',#23250,#23251,#19242,.T.);
#29642=EDGE_CURVE('',#23251,#23252,#19243,.T.);
#29643=EDGE_CURVE('',#23252,#23253,#19787,.T.);
#29644=EDGE_CURVE('',#23253,#23254,#19244,.T.);
#29645=EDGE_CURVE('',#23254,#23255,#19245,.T.);
#29646=EDGE_CURVE('',#23255,#23256,#19246,.T.);
#29647=EDGE_CURVE('',#23256,#23257,#19788,.T.);
#29648=EDGE_CURVE('',#23257,#23258,#19247,.T.);
#29649=EDGE_CURVE('',#23258,#23259,#19248,.T.);
#29650=EDGE_CURVE('',#23259,#23260,#19249,.T.);
#29651=EDGE_CURVE('',#23260,#23261,#19789,.T.);
#29652=EDGE_CURVE('',#23261,#23262,#19250,.T.);
#29653=EDGE_CURVE('',#23262,#23263,#19251,.T.);
#29654=EDGE_CURVE('',#23263,#23264,#19252,.T.);
#29655=EDGE_CURVE('',#23264,#23265,#19790,.T.);
#29656=EDGE_CURVE('',#23265,#23266,#19253,.T.);
#29657=EDGE_CURVE('',#23266,#23267,#19254,.T.);
#29658=EDGE_CURVE('',#23267,#23268,#19255,.T.);
#29659=EDGE_CURVE('',#23268,#23269,#19791,.T.);
#29660=EDGE_CURVE('',#23269,#23270,#19256,.T.);
#29661=EDGE_CURVE('',#23270,#23271,#19257,.T.);
#29662=EDGE_CURVE('',#23271,#23272,#19258,.T.);
#29663=EDGE_CURVE('',#23272,#23273,#19792,.T.);
#29664=EDGE_CURVE('',#23273,#23274,#19259,.T.);
#29665=EDGE_CURVE('',#23274,#23275,#19260,.T.);
#29666=EDGE_CURVE('',#23275,#23276,#19261,.T.);
#29667=EDGE_CURVE('',#23276,#23277,#19793,.T.);
#29668=EDGE_CURVE('',#23277,#23278,#19262,.T.);
#29669=EDGE_CURVE('',#23278,#23279,#19263,.T.);
#29670=EDGE_CURVE('',#23279,#23280,#19264,.T.);
#29671=EDGE_CURVE('',#23280,#23281,#19794,.T.);
#29672=EDGE_CURVE('',#23281,#23282,#19265,.T.);
#29673=EDGE_CURVE('',#23282,#23283,#19266,.T.);
#29674=EDGE_CURVE('',#23283,#23284,#19267,.T.);
#29675=EDGE_CURVE('',#23284,#23285,#19795,.T.);
#29676=EDGE_CURVE('',#23285,#23286,#19268,.T.);
#29677=EDGE_CURVE('',#23286,#23287,#19269,.T.);
#29678=EDGE_CURVE('',#23287,#23288,#19270,.T.);
#29679=EDGE_CURVE('',#23288,#23289,#19796,.T.);
#29680=EDGE_CURVE('',#23289,#23290,#19271,.T.);
#29681=EDGE_CURVE('',#23290,#23291,#19272,.T.);
#29682=EDGE_CURVE('',#23291,#23292,#19273,.T.);
#29683=EDGE_CURVE('',#23292,#23243,#19797,.T.);
#29684=EDGE_CURVE('',#23097,#23293,#19274,.T.);
#29685=EDGE_CURVE('',#23293,#23294,#19275,.T.);
#29686=EDGE_CURVE('',#23294,#23295,#19276,.T.);
#29687=EDGE_CURVE('',#23295,#23296,#19798,.T.);
#29688=EDGE_CURVE('',#23296,#23297,#19277,.T.);
#29689=EDGE_CURVE('',#23297,#23298,#19278,.T.);
#29690=EDGE_CURVE('',#23298,#23299,#19279,.T.);
#29691=EDGE_CURVE('',#23299,#23300,#19799,.T.);
#29692=EDGE_CURVE('',#23300,#23301,#19280,.T.);
#29693=EDGE_CURVE('',#23301,#23302,#19281,.T.);
#29694=EDGE_CURVE('',#23302,#23303,#19282,.T.);
#29695=EDGE_CURVE('',#23303,#23304,#19800,.T.);
#29696=EDGE_CURVE('',#23304,#23305,#19283,.T.);
#29697=EDGE_CURVE('',#23305,#23306,#19284,.T.);
#29698=EDGE_CURVE('',#23306,#23307,#19285,.T.);
#29699=EDGE_CURVE('',#23307,#23308,#19801,.T.);
#29700=EDGE_CURVE('',#23308,#23309,#19286,.T.);
#29701=EDGE_CURVE('',#23309,#23310,#19287,.T.);
#29702=EDGE_CURVE('',#23310,#23311,#19288,.T.);
#29703=EDGE_CURVE('',#23311,#23312,#19802,.T.);
#29704=EDGE_CURVE('',#23312,#23313,#19289,.T.);
#29705=EDGE_CURVE('',#23313,#23314,#19290,.T.);
#29706=EDGE_CURVE('',#23314,#23315,#19291,.T.);
#29707=EDGE_CURVE('',#23315,#23316,#19803,.T.);
#29708=EDGE_CURVE('',#23316,#23317,#19292,.T.);
#29709=EDGE_CURVE('',#23317,#23318,#19293,.T.);
#29710=EDGE_CURVE('',#23318,#23319,#19294,.T.);
#29711=EDGE_CURVE('',#23319,#23320,#19804,.T.);
#29712=EDGE_CURVE('',#23320,#23321,#19295,.T.);
#29713=EDGE_CURVE('',#23321,#23322,#19296,.T.);
#29714=EDGE_CURVE('',#23322,#23323,#19297,.T.);
#29715=EDGE_CURVE('',#23323,#23324,#19805,.T.);
#29716=EDGE_CURVE('',#23324,#23325,#19298,.T.);
#29717=EDGE_CURVE('',#23325,#23326,#19299,.T.);
#29718=EDGE_CURVE('',#23326,#23327,#19300,.T.);
#29719=EDGE_CURVE('',#23327,#23328,#19806,.T.);
#29720=EDGE_CURVE('',#23328,#23329,#19301,.T.);
#29721=EDGE_CURVE('',#23329,#23330,#19302,.T.);
#29722=EDGE_CURVE('',#23330,#23331,#19303,.T.);
#29723=EDGE_CURVE('',#23331,#23332,#19807,.T.);
#29724=EDGE_CURVE('',#23332,#23333,#19304,.T.);
#29725=EDGE_CURVE('',#23333,#23334,#19305,.T.);
#29726=EDGE_CURVE('',#23334,#23335,#19306,.T.);
#29727=EDGE_CURVE('',#23335,#23336,#19808,.T.);
#29728=EDGE_CURVE('',#23336,#23337,#19307,.T.);
#29729=EDGE_CURVE('',#23084,#23337,#19809,.T.);
#29730=EDGE_CURVE('',#23196,#23100,#4859,.T.);
#29731=EDGE_CURVE('',#23338,#23245,#19810,.T.);
#29732=EDGE_CURVE('',#23338,#23339,#19308,.T.);
#29733=EDGE_CURVE('',#23339,#23340,#19309,.T.);
#29734=EDGE_CURVE('',#23340,#23341,#19310,.T.);
#29735=EDGE_CURVE('',#23342,#23341,#19811,.T.);
#29736=EDGE_CURVE('',#23342,#23343,#19311,.T.);
#29737=EDGE_CURVE('',#23343,#23344,#19312,.T.);
#29738=EDGE_CURVE('',#23344,#23345,#19313,.T.);
#29739=EDGE_CURVE('',#23346,#23345,#19812,.T.);
#29740=EDGE_CURVE('',#23346,#23347,#19314,.T.);
#29741=EDGE_CURVE('',#23347,#23348,#19315,.T.);
#29742=EDGE_CURVE('',#23348,#23349,#19316,.T.);
#29743=EDGE_CURVE('',#23350,#23349,#19813,.T.);
#29744=EDGE_CURVE('',#23350,#23351,#19317,.T.);
#29745=EDGE_CURVE('',#23351,#23352,#19318,.T.);
#29746=EDGE_CURVE('',#23352,#23353,#19319,.T.);
#29747=EDGE_CURVE('',#23354,#23353,#19814,.T.);
#29748=EDGE_CURVE('',#23354,#23355,#19320,.T.);
#29749=EDGE_CURVE('',#23355,#23356,#19321,.T.);
#29750=EDGE_CURVE('',#23356,#23357,#19322,.T.);
#29751=EDGE_CURVE('',#23358,#23357,#19815,.T.);
#29752=EDGE_CURVE('',#23358,#23359,#19323,.T.);
#29753=EDGE_CURVE('',#23359,#23360,#19324,.T.);
#29754=EDGE_CURVE('',#23360,#23361,#19325,.T.);
#29755=EDGE_CURVE('',#23362,#23361,#19816,.T.);
#29756=EDGE_CURVE('',#23362,#23363,#19326,.T.);
#29757=EDGE_CURVE('',#23363,#23364,#19327,.T.);
#29758=EDGE_CURVE('',#23364,#23365,#19328,.T.);
#29759=EDGE_CURVE('',#23366,#23365,#19817,.T.);
#29760=EDGE_CURVE('',#23366,#23367,#19329,.T.);
#29761=EDGE_CURVE('',#23367,#23368,#19330,.T.);
#29762=EDGE_CURVE('',#23368,#23369,#19331,.T.);
#29763=EDGE_CURVE('',#23370,#23369,#19818,.T.);
#29764=EDGE_CURVE('',#23370,#23371,#19332,.T.);
#29765=EDGE_CURVE('',#23371,#23372,#19333,.T.);
#29766=EDGE_CURVE('',#23372,#23373,#19334,.T.);
#29767=EDGE_CURVE('',#23374,#23373,#19819,.T.);
#29768=EDGE_CURVE('',#23374,#23375,#19335,.T.);
#29769=EDGE_CURVE('',#23375,#23376,#19336,.T.);
#29770=EDGE_CURVE('',#23376,#23377,#19337,.T.);
#29771=EDGE_CURVE('',#23378,#23377,#19820,.T.);
#29772=EDGE_CURVE('',#23378,#23379,#19338,.T.);
#29773=EDGE_CURVE('',#23379,#23380,#19339,.T.);
#29774=EDGE_CURVE('',#23380,#23381,#19340,.T.);
#29775=EDGE_CURVE('',#23382,#23381,#19821,.T.);
#29776=EDGE_CURVE('',#23382,#23148,#19341,.T.);
#29777=EDGE_CURVE('',#23383,#23247,#4860,.T.);
#29778=EDGE_CURVE('',#23149,#23383,#4861,.T.);
#29779=EDGE_CURVE('',#23248,#23382,#4862,.T.);
#29780=EDGE_CURVE('',#23198,#23336,#4863,.T.);
#29781=EDGE_CURVE('',#23150,#23384,#4864,.T.);
#29782=EDGE_CURVE('',#23337,#23384,#4865,.T.);
#29783=EDGE_CURVE('',#23384,#23383,#4866,.T.);
#29784=EDGE_CURVE('',#23381,#23249,#4867,.T.);
#29785=EDGE_CURVE('',#23385,#23386,#19342,.T.);
#29786=EDGE_CURVE('',#23387,#23385,#19343,.T.);
#29787=EDGE_CURVE('',#23388,#23387,#19344,.T.);
#29788=EDGE_CURVE('',#23386,#23388,#19822,.T.);
#29789=EDGE_CURVE('',#23389,#23390,#19345,.T.);
#29790=EDGE_CURVE('',#23391,#23389,#19346,.T.);
#29791=EDGE_CURVE('',#23392,#23391,#19347,.T.);
#29792=EDGE_CURVE('',#23390,#23392,#19823,.T.);
#29793=EDGE_CURVE('',#23393,#23394,#19348,.T.);
#29794=EDGE_CURVE('',#23395,#23393,#19349,.T.);
#29795=EDGE_CURVE('',#23396,#23395,#19350,.T.);
#29796=EDGE_CURVE('',#23394,#23396,#19824,.T.);
#29797=EDGE_CURVE('',#23397,#23398,#19351,.T.);
#29798=EDGE_CURVE('',#23399,#23397,#19352,.T.);
#29799=EDGE_CURVE('',#23400,#23399,#19353,.T.);
#29800=EDGE_CURVE('',#23398,#23400,#19825,.T.);
#29801=EDGE_CURVE('',#23401,#23402,#19354,.T.);
#29802=EDGE_CURVE('',#23403,#23401,#19355,.T.);
#29803=EDGE_CURVE('',#23404,#23403,#19356,.T.);
#29804=EDGE_CURVE('',#23402,#23404,#19826,.T.);
#29805=EDGE_CURVE('',#23405,#23406,#19357,.T.);
#29806=EDGE_CURVE('',#23407,#23405,#19358,.T.);
#29807=EDGE_CURVE('',#23408,#23407,#19359,.T.);
#29808=EDGE_CURVE('',#23406,#23408,#19827,.T.);
#29809=EDGE_CURVE('',#23409,#23410,#19360,.T.);
#29810=EDGE_CURVE('',#23411,#23409,#19361,.T.);
#29811=EDGE_CURVE('',#23412,#23411,#19362,.T.);
#29812=EDGE_CURVE('',#23410,#23412,#19828,.T.);
#29813=EDGE_CURVE('',#23413,#23414,#19363,.T.);
#29814=EDGE_CURVE('',#23415,#23413,#19364,.T.);
#29815=EDGE_CURVE('',#23416,#23415,#19365,.T.);
#29816=EDGE_CURVE('',#23414,#23416,#19829,.T.);
#29817=EDGE_CURVE('',#23417,#23418,#19366,.T.);
#29818=EDGE_CURVE('',#23419,#23417,#19367,.T.);
#29819=EDGE_CURVE('',#23420,#23419,#19368,.T.);
#29820=EDGE_CURVE('',#23418,#23420,#19830,.T.);
#29821=EDGE_CURVE('',#23421,#23422,#19369,.T.);
#29822=EDGE_CURVE('',#23423,#23421,#19370,.T.);
#29823=EDGE_CURVE('',#23424,#23423,#19371,.T.);
#29824=EDGE_CURVE('',#23422,#23424,#19831,.T.);
#29825=EDGE_CURVE('',#23425,#23426,#19372,.T.);
#29826=EDGE_CURVE('',#23427,#23425,#19373,.T.);
#29827=EDGE_CURVE('',#23428,#23427,#19374,.T.);
#29828=EDGE_CURVE('',#23426,#23428,#19832,.T.);
#29829=EDGE_CURVE('',#23429,#23430,#19375,.T.);
#29830=EDGE_CURVE('',#23431,#23429,#19376,.T.);
#29831=EDGE_CURVE('',#23432,#23431,#19377,.T.);
#29832=EDGE_CURVE('',#23430,#23432,#19833,.T.);
#29833=EDGE_CURVE('',#23433,#23434,#19378,.T.);
#29834=EDGE_CURVE('',#23435,#23433,#19379,.T.);
#29835=EDGE_CURVE('',#23436,#23435,#19380,.T.);
#29836=EDGE_CURVE('',#23434,#23436,#19834,.T.);
#29837=EDGE_CURVE('',#23437,#23438,#19381,.T.);
#29838=EDGE_CURVE('',#23439,#23437,#19382,.T.);
#29839=EDGE_CURVE('',#23440,#23439,#19383,.T.);
#29840=EDGE_CURVE('',#23438,#23440,#19835,.T.);
#29841=EDGE_CURVE('',#23441,#23442,#19384,.T.);
#29842=EDGE_CURVE('',#23443,#23441,#19385,.T.);
#29843=EDGE_CURVE('',#23444,#23443,#19386,.T.);
#29844=EDGE_CURVE('',#23442,#23444,#19836,.T.);
#29845=EDGE_CURVE('',#23445,#23446,#19387,.T.);
#29846=EDGE_CURVE('',#23447,#23445,#19388,.T.);
#29847=EDGE_CURVE('',#23448,#23447,#19389,.T.);
#29848=EDGE_CURVE('',#23446,#23448,#19837,.T.);
#29849=EDGE_CURVE('',#23449,#23450,#19390,.T.);
#29850=EDGE_CURVE('',#23451,#23449,#19391,.T.);
#29851=EDGE_CURVE('',#23452,#23451,#19392,.T.);
#29852=EDGE_CURVE('',#23450,#23452,#19838,.T.);
#29853=EDGE_CURVE('',#23453,#23454,#19393,.T.);
#29854=EDGE_CURVE('',#23455,#23453,#19394,.T.);
#29855=EDGE_CURVE('',#23456,#23455,#19395,.T.);
#29856=EDGE_CURVE('',#23454,#23456,#19839,.T.);
#29857=EDGE_CURVE('',#23457,#23458,#19396,.T.);
#29858=EDGE_CURVE('',#23459,#23457,#19397,.T.);
#29859=EDGE_CURVE('',#23460,#23459,#19398,.T.);
#29860=EDGE_CURVE('',#23458,#23460,#19840,.T.);
#29861=EDGE_CURVE('',#23461,#23462,#19399,.T.);
#29862=EDGE_CURVE('',#23463,#23461,#19400,.T.);
#29863=EDGE_CURVE('',#23464,#23463,#19401,.T.);
#29864=EDGE_CURVE('',#23462,#23464,#19841,.T.);
#29865=EDGE_CURVE('',#23465,#23466,#19402,.T.);
#29866=EDGE_CURVE('',#23467,#23465,#19403,.T.);
#29867=EDGE_CURVE('',#23468,#23467,#19404,.T.);
#29868=EDGE_CURVE('',#23466,#23468,#19842,.T.);
#29869=EDGE_CURVE('',#23469,#23470,#19405,.T.);
#29870=EDGE_CURVE('',#23471,#23469,#19406,.T.);
#29871=EDGE_CURVE('',#23472,#23471,#19407,.T.);
#29872=EDGE_CURVE('',#23470,#23472,#19843,.T.);
#29873=EDGE_CURVE('',#23473,#23474,#19408,.T.);
#29874=EDGE_CURVE('',#23475,#23473,#19409,.T.);
#29875=EDGE_CURVE('',#23476,#23475,#19410,.T.);
#29876=EDGE_CURVE('',#23474,#23476,#19844,.T.);
#29877=EDGE_CURVE('',#23477,#23478,#19411,.T.);
#29878=EDGE_CURVE('',#23479,#23477,#19412,.T.);
#29879=EDGE_CURVE('',#23480,#23479,#19413,.T.);
#29880=EDGE_CURVE('',#23478,#23480,#19845,.T.);
#29881=EDGE_CURVE('',#23481,#23482,#19414,.T.);
#29882=EDGE_CURVE('',#23483,#23481,#19415,.T.);
#29883=EDGE_CURVE('',#23484,#23483,#19416,.T.);
#29884=EDGE_CURVE('',#23482,#23484,#19846,.T.);
#29885=EDGE_CURVE('',#23485,#23486,#19417,.T.);
#29886=EDGE_CURVE('',#23487,#23485,#19418,.T.);
#29887=EDGE_CURVE('',#23488,#23487,#19419,.T.);
#29888=EDGE_CURVE('',#23486,#23488,#19847,.T.);
#29889=EDGE_CURVE('',#23489,#23490,#19420,.T.);
#29890=EDGE_CURVE('',#23491,#23489,#19421,.T.);
#29891=EDGE_CURVE('',#23492,#23491,#19422,.T.);
#29892=EDGE_CURVE('',#23490,#23492,#19848,.T.);
#29893=EDGE_CURVE('',#23493,#23494,#19423,.T.);
#29894=EDGE_CURVE('',#23495,#23493,#19424,.T.);
#29895=EDGE_CURVE('',#23496,#23495,#19425,.T.);
#29896=EDGE_CURVE('',#23494,#23496,#19849,.T.);
#29897=EDGE_CURVE('',#23497,#23498,#19426,.T.);
#29898=EDGE_CURVE('',#23499,#23497,#19427,.T.);
#29899=EDGE_CURVE('',#23500,#23499,#19428,.T.);
#29900=EDGE_CURVE('',#23498,#23500,#19850,.T.);
#29901=EDGE_CURVE('',#23501,#23502,#19429,.T.);
#29902=EDGE_CURVE('',#23503,#23501,#19430,.T.);
#29903=EDGE_CURVE('',#23504,#23503,#19431,.T.);
#29904=EDGE_CURVE('',#23502,#23504,#19851,.T.);
#29905=EDGE_CURVE('',#23505,#23506,#19432,.T.);
#29906=EDGE_CURVE('',#23507,#23505,#19433,.T.);
#29907=EDGE_CURVE('',#23508,#23507,#19434,.T.);
#29908=EDGE_CURVE('',#23506,#23508,#19852,.T.);
#29909=EDGE_CURVE('',#23509,#23510,#19435,.T.);
#29910=EDGE_CURVE('',#23511,#23509,#19436,.T.);
#29911=EDGE_CURVE('',#23512,#23511,#19437,.T.);
#29912=EDGE_CURVE('',#23510,#23512,#19853,.T.);
#29913=EDGE_CURVE('',#23513,#23514,#19438,.T.);
#29914=EDGE_CURVE('',#23515,#23513,#19439,.T.);
#29915=EDGE_CURVE('',#23516,#23515,#19440,.T.);
#29916=EDGE_CURVE('',#23514,#23516,#19854,.T.);
#29917=EDGE_CURVE('',#23517,#23515,#4868,.T.);
#29918=EDGE_CURVE('',#23517,#23518,#19441,.T.);
#29919=EDGE_CURVE('',#23518,#23519,#4869,.T.);
#29920=EDGE_CURVE('',#23519,#23200,#4870,.T.);
#29921=EDGE_CURVE('',#23335,#23199,#4871,.T.);
#29922=EDGE_CURVE('',#23334,#23520,#4872,.T.);
#29923=EDGE_CURVE('',#23516,#23520,#4873,.T.);
#29924=EDGE_CURVE('',#23521,#23513,#4874,.T.);
#29925=EDGE_CURVE('',#23521,#23517,#19442,.T.);
#29926=EDGE_CURVE('',#23522,#23511,#4875,.T.);
#29927=EDGE_CURVE('',#23522,#23523,#19443,.T.);
#29928=EDGE_CURVE('',#23523,#23524,#4876,.T.);
#29929=EDGE_CURVE('',#23524,#23204,#4877,.T.);
#29930=EDGE_CURVE('',#23331,#23203,#4878,.T.);
#29931=EDGE_CURVE('',#23330,#23525,#4879,.T.);
#29932=EDGE_CURVE('',#23512,#23525,#4880,.T.);
#29933=EDGE_CURVE('',#23526,#23509,#4881,.T.);
#29934=EDGE_CURVE('',#23526,#23522,#19444,.T.);
#29935=EDGE_CURVE('',#23527,#23507,#4882,.T.);
#29936=EDGE_CURVE('',#23527,#23528,#19445,.T.);
#29937=EDGE_CURVE('',#23528,#23529,#4883,.T.);
#29938=EDGE_CURVE('',#23529,#23208,#4884,.T.);
#29939=EDGE_CURVE('',#23327,#23207,#4885,.T.);
#29940=EDGE_CURVE('',#23326,#23530,#4886,.T.);
#29941=EDGE_CURVE('',#23508,#23530,#4887,.T.);
#29942=EDGE_CURVE('',#23531,#23505,#4888,.T.);
#29943=EDGE_CURVE('',#23531,#23527,#19446,.T.);
#29944=EDGE_CURVE('',#23532,#23503,#4889,.T.);
#29945=EDGE_CURVE('',#23532,#23533,#19447,.T.);
#29946=EDGE_CURVE('',#23533,#23534,#4890,.T.);
#29947=EDGE_CURVE('',#23534,#23212,#4891,.T.);
#29948=EDGE_CURVE('',#23323,#23211,#4892,.T.);
#29949=EDGE_CURVE('',#23322,#23535,#4893,.T.);
#29950=EDGE_CURVE('',#23504,#23535,#4894,.T.);
#29951=EDGE_CURVE('',#23536,#23501,#4895,.T.);
#29952=EDGE_CURVE('',#23536,#23532,#19448,.T.);
#29953=EDGE_CURVE('',#23537,#23499,#4896,.T.);
#29954=EDGE_CURVE('',#23537,#23538,#19449,.T.);
#29955=EDGE_CURVE('',#23538,#23539,#4897,.T.);
#29956=EDGE_CURVE('',#23539,#23216,#4898,.T.);
#29957=EDGE_CURVE('',#23319,#23215,#4899,.T.);
#29958=EDGE_CURVE('',#23318,#23540,#4900,.T.);
#29959=EDGE_CURVE('',#23500,#23540,#4901,.T.);
#29960=EDGE_CURVE('',#23541,#23497,#4902,.T.);
#29961=EDGE_CURVE('',#23541,#23537,#19450,.T.);
#29962=EDGE_CURVE('',#23542,#23495,#4903,.T.);
#29963=EDGE_CURVE('',#23542,#23543,#19451,.T.);
#29964=EDGE_CURVE('',#23543,#23544,#4904,.T.);
#29965=EDGE_CURVE('',#23544,#23220,#4905,.T.);
#29966=EDGE_CURVE('',#23315,#23219,#4906,.T.);
#29967=EDGE_CURVE('',#23314,#23545,#4907,.T.);
#29968=EDGE_CURVE('',#23496,#23545,#4908,.T.);
#29969=EDGE_CURVE('',#23546,#23493,#4909,.T.);
#29970=EDGE_CURVE('',#23546,#23542,#19452,.T.);
#29971=EDGE_CURVE('',#23547,#23491,#4910,.T.);
#29972=EDGE_CURVE('',#23547,#23548,#19453,.T.);
#29973=EDGE_CURVE('',#23548,#23549,#4911,.T.);
#29974=EDGE_CURVE('',#23549,#23224,#4912,.T.);
#29975=EDGE_CURVE('',#23311,#23223,#4913,.T.);
#29976=EDGE_CURVE('',#23310,#23550,#4914,.T.);
#29977=EDGE_CURVE('',#23492,#23550,#4915,.T.);
#29978=EDGE_CURVE('',#23551,#23489,#4916,.T.);
#29979=EDGE_CURVE('',#23551,#23547,#19454,.T.);
#29980=EDGE_CURVE('',#23552,#23487,#4917,.T.);
#29981=EDGE_CURVE('',#23552,#23553,#19455,.T.);
#29982=EDGE_CURVE('',#23553,#23554,#4918,.T.);
#29983=EDGE_CURVE('',#23554,#23228,#4919,.T.);
#29984=EDGE_CURVE('',#23307,#23227,#4920,.T.);
#29985=EDGE_CURVE('',#23306,#23555,#4921,.T.);
#29986=EDGE_CURVE('',#23488,#23555,#4922,.T.);
#29987=EDGE_CURVE('',#23556,#23485,#4923,.T.);
#29988=EDGE_CURVE('',#23556,#23552,#19456,.T.);
#29989=EDGE_CURVE('',#23557,#23483,#4924,.T.);
#29990=EDGE_CURVE('',#23557,#23558,#19457,.T.);
#29991=EDGE_CURVE('',#23558,#23559,#4925,.T.);
#29992=EDGE_CURVE('',#23559,#23232,#4926,.T.);
#29993=EDGE_CURVE('',#23303,#23231,#4927,.T.);
#29994=EDGE_CURVE('',#23302,#23560,#4928,.T.);
#29995=EDGE_CURVE('',#23484,#23560,#4929,.T.);
#29996=EDGE_CURVE('',#23561,#23481,#4930,.T.);
#29997=EDGE_CURVE('',#23561,#23557,#19458,.T.);
#29998=EDGE_CURVE('',#23562,#23479,#4931,.T.);
#29999=EDGE_CURVE('',#23562,#23563,#19459,.T.);
#30000=EDGE_CURVE('',#23563,#23564,#4932,.T.);
#30001=EDGE_CURVE('',#23564,#23236,#4933,.T.);
#30002=EDGE_CURVE('',#23299,#23235,#4934,.T.);
#30003=EDGE_CURVE('',#23298,#23565,#4935,.T.);
#30004=EDGE_CURVE('',#23480,#23565,#4936,.T.);
#30005=EDGE_CURVE('',#23566,#23477,#4937,.T.);
#30006=EDGE_CURVE('',#23566,#23562,#19460,.T.);
#30007=EDGE_CURVE('',#23567,#23475,#4938,.T.);
#30008=EDGE_CURVE('',#23567,#23568,#19461,.T.);
#30009=EDGE_CURVE('',#23568,#23569,#4939,.T.);
#30010=EDGE_CURVE('',#23569,#23240,#4940,.T.);
#30011=EDGE_CURVE('',#23295,#23239,#4941,.T.);
#30012=EDGE_CURVE('',#23294,#23570,#4942,.T.);
#30013=EDGE_CURVE('',#23476,#23570,#4943,.T.);
#30014=EDGE_CURVE('',#23571,#23473,#4944,.T.);
#30015=EDGE_CURVE('',#23571,#23567,#19462,.T.);
#30016=EDGE_CURVE('',#23572,#23471,#4945,.T.);
#30017=EDGE_CURVE('',#23572,#23573,#19463,.T.);
#30018=EDGE_CURVE('',#23573,#23574,#4946,.T.);
#30019=EDGE_CURVE('',#23574,#23154,#4947,.T.);
#30020=EDGE_CURVE('',#23143,#23153,#4948,.T.);
#30021=EDGE_CURVE('',#23142,#23575,#4949,.T.);
#30022=EDGE_CURVE('',#23472,#23575,#4950,.T.);
#30023=EDGE_CURVE('',#23576,#23469,#4951,.T.);
#30024=EDGE_CURVE('',#23576,#23572,#19464,.T.);
#30025=EDGE_CURVE('',#23577,#23467,#4952,.T.);
#30026=EDGE_CURVE('',#23577,#23578,#19465,.T.);
#30027=EDGE_CURVE('',#23578,#23579,#4953,.T.);
#30028=EDGE_CURVE('',#23579,#23158,#4954,.T.);
#30029=EDGE_CURVE('',#23139,#23157,#4955,.T.);
#30030=EDGE_CURVE('',#23138,#23580,#4956,.T.);
#30031=EDGE_CURVE('',#23468,#23580,#4957,.T.);
#30032=EDGE_CURVE('',#23581,#23465,#4958,.T.);
#30033=EDGE_CURVE('',#23581,#23577,#19466,.T.);
#30034=EDGE_CURVE('',#23582,#23463,#4959,.T.);
#30035=EDGE_CURVE('',#23582,#23583,#19467,.T.);
#30036=EDGE_CURVE('',#23583,#23584,#4960,.T.);
#30037=EDGE_CURVE('',#23584,#23162,#4961,.T.);
#30038=EDGE_CURVE('',#23135,#23161,#4962,.T.);
#30039=EDGE_CURVE('',#23134,#23585,#4963,.T.);
#30040=EDGE_CURVE('',#23464,#23585,#4964,.T.);
#30041=EDGE_CURVE('',#23586,#23461,#4965,.T.);
#30042=EDGE_CURVE('',#23586,#23582,#19468,.T.);
#30043=EDGE_CURVE('',#23587,#23459,#4966,.T.);
#30044=EDGE_CURVE('',#23587,#23588,#19469,.T.);
#30045=EDGE_CURVE('',#23588,#23589,#4967,.T.);
#30046=EDGE_CURVE('',#23589,#23166,#4968,.T.);
#30047=EDGE_CURVE('',#23131,#23165,#4969,.T.);
#30048=EDGE_CURVE('',#23130,#23590,#4970,.T.);
#30049=EDGE_CURVE('',#23460,#23590,#4971,.T.);
#30050=EDGE_CURVE('',#23591,#23457,#4972,.T.);
#30051=EDGE_CURVE('',#23591,#23587,#19470,.T.);
#30052=EDGE_CURVE('',#23592,#23455,#4973,.T.);
#30053=EDGE_CURVE('',#23592,#23593,#19471,.T.);
#30054=EDGE_CURVE('',#23593,#23594,#4974,.T.);
#30055=EDGE_CURVE('',#23594,#23170,#4975,.T.);
#30056=EDGE_CURVE('',#23127,#23169,#4976,.T.);
#30057=EDGE_CURVE('',#23126,#23595,#4977,.T.);
#30058=EDGE_CURVE('',#23456,#23595,#4978,.T.);
#30059=EDGE_CURVE('',#23596,#23453,#4979,.T.);
#30060=EDGE_CURVE('',#23596,#23592,#19472,.T.);
#30061=EDGE_CURVE('',#23597,#23451,#4980,.T.);
#30062=EDGE_CURVE('',#23597,#23598,#19473,.T.);
#30063=EDGE_CURVE('',#23598,#23599,#4981,.T.);
#30064=EDGE_CURVE('',#23599,#23174,#4982,.T.);
#30065=EDGE_CURVE('',#23123,#23173,#4983,.T.);
#30066=EDGE_CURVE('',#23122,#23600,#4984,.T.);
#30067=EDGE_CURVE('',#23452,#23600,#4985,.T.);
#30068=EDGE_CURVE('',#23601,#23449,#4986,.T.);
#30069=EDGE_CURVE('',#23601,#23597,#19474,.T.);
#30070=EDGE_CURVE('',#23602,#23447,#4987,.T.);
#30071=EDGE_CURVE('',#23602,#23603,#19475,.T.);
#30072=EDGE_CURVE('',#23603,#23604,#4988,.T.);
#30073=EDGE_CURVE('',#23604,#23178,#4989,.T.);
#30074=EDGE_CURVE('',#23119,#23177,#4990,.T.);
#30075=EDGE_CURVE('',#23118,#23605,#4991,.T.);
#30076=EDGE_CURVE('',#23448,#23605,#4992,.T.);
#30077=EDGE_CURVE('',#23606,#23445,#4993,.T.);
#30078=EDGE_CURVE('',#23606,#23602,#19476,.T.);
#30079=EDGE_CURVE('',#23607,#23443,#4994,.T.);
#30080=EDGE_CURVE('',#23607,#23608,#19477,.T.);
#30081=EDGE_CURVE('',#23608,#23609,#4995,.T.);
#30082=EDGE_CURVE('',#23609,#23182,#4996,.T.);
#30083=EDGE_CURVE('',#23115,#23181,#4997,.T.);
#30084=EDGE_CURVE('',#23114,#23610,#4998,.T.);
#30085=EDGE_CURVE('',#23444,#23610,#4999,.T.);
#30086=EDGE_CURVE('',#23611,#23441,#5000,.T.);
#30087=EDGE_CURVE('',#23611,#23607,#19478,.T.);
#30088=EDGE_CURVE('',#23612,#23439,#5001,.T.);
#30089=EDGE_CURVE('',#23612,#23613,#19479,.T.);
#30090=EDGE_CURVE('',#23613,#23614,#5002,.T.);
#30091=EDGE_CURVE('',#23614,#23186,#5003,.T.);
#30092=EDGE_CURVE('',#23111,#23185,#5004,.T.);
#30093=EDGE_CURVE('',#23110,#23615,#5005,.T.);
#30094=EDGE_CURVE('',#23440,#23615,#5006,.T.);
#30095=EDGE_CURVE('',#23616,#23437,#5007,.T.);
#30096=EDGE_CURVE('',#23616,#23612,#19480,.T.);
#30097=EDGE_CURVE('',#23617,#23435,#5008,.T.);
#30098=EDGE_CURVE('',#23617,#23618,#19481,.T.);
#30099=EDGE_CURVE('',#23618,#23619,#5009,.T.);
#30100=EDGE_CURVE('',#23619,#23190,#5010,.T.);
#30101=EDGE_CURVE('',#23107,#23189,#5011,.T.);
#30102=EDGE_CURVE('',#23106,#23620,#5012,.T.);
#30103=EDGE_CURVE('',#23436,#23620,#5013,.T.);
#30104=EDGE_CURVE('',#23621,#23433,#5014,.T.);
#30105=EDGE_CURVE('',#23621,#23617,#19482,.T.);
#30106=EDGE_CURVE('',#23622,#23431,#5015,.T.);
#30107=EDGE_CURVE('',#23622,#23623,#19483,.T.);
#30108=EDGE_CURVE('',#23623,#23624,#5016,.T.);
#30109=EDGE_CURVE('',#23624,#23194,#5017,.T.);
#30110=EDGE_CURVE('',#23103,#23193,#5018,.T.);
#30111=EDGE_CURVE('',#23102,#23625,#5019,.T.);
#30112=EDGE_CURVE('',#23432,#23625,#5020,.T.);
#30113=EDGE_CURVE('',#23626,#23429,#5021,.T.);
#30114=EDGE_CURVE('',#23626,#23622,#19484,.T.);
#30115=EDGE_CURVE('',#23627,#23427,#5022,.T.);
#30116=EDGE_CURVE('',#23627,#23628,#19485,.T.);
#30117=EDGE_CURVE('',#23628,#23629,#5023,.T.);
#30118=EDGE_CURVE('',#23629,#23339,#5024,.T.);
#30119=EDGE_CURVE('',#23292,#23338,#5025,.T.);
#30120=EDGE_CURVE('',#23291,#23630,#5026,.T.);
#30121=EDGE_CURVE('',#23428,#23630,#5027,.T.);
#30122=EDGE_CURVE('',#23631,#23425,#5028,.T.);
#30123=EDGE_CURVE('',#23631,#23627,#19486,.T.);
#30124=EDGE_CURVE('',#23632,#23423,#5029,.T.);
#30125=EDGE_CURVE('',#23632,#23633,#19487,.T.);
#30126=EDGE_CURVE('',#23633,#23634,#5030,.T.);
#30127=EDGE_CURVE('',#23634,#23343,#5031,.T.);
#30128=EDGE_CURVE('',#23288,#23342,#5032,.T.);
#30129=EDGE_CURVE('',#23287,#23635,#5033,.T.);
#30130=EDGE_CURVE('',#23424,#23635,#5034,.T.);
#30131=EDGE_CURVE('',#23636,#23421,#5035,.T.);
#30132=EDGE_CURVE('',#23636,#23632,#19488,.T.);
#30133=EDGE_CURVE('',#23637,#23419,#5036,.T.);
#30134=EDGE_CURVE('',#23637,#23638,#19489,.T.);
#30135=EDGE_CURVE('',#23638,#23639,#5037,.T.);
#30136=EDGE_CURVE('',#23639,#23347,#5038,.T.);
#30137=EDGE_CURVE('',#23284,#23346,#5039,.T.);
#30138=EDGE_CURVE('',#23283,#23640,#5040,.T.);
#30139=EDGE_CURVE('',#23420,#23640,#5041,.T.);
#30140=EDGE_CURVE('',#23641,#23417,#5042,.T.);
#30141=EDGE_CURVE('',#23641,#23637,#19490,.T.);
#30142=EDGE_CURVE('',#23642,#23415,#5043,.T.);
#30143=EDGE_CURVE('',#23642,#23643,#19491,.T.);
#30144=EDGE_CURVE('',#23643,#23644,#5044,.T.);
#30145=EDGE_CURVE('',#23644,#23351,#5045,.T.);
#30146=EDGE_CURVE('',#23280,#23350,#5046,.T.);
#30147=EDGE_CURVE('',#23279,#23645,#5047,.T.);
#30148=EDGE_CURVE('',#23416,#23645,#5048,.T.);
#30149=EDGE_CURVE('',#23646,#23413,#5049,.T.);
#30150=EDGE_CURVE('',#23646,#23642,#19492,.T.);
#30151=EDGE_CURVE('',#23647,#23411,#5050,.T.);
#30152=EDGE_CURVE('',#23647,#23648,#19493,.T.);
#30153=EDGE_CURVE('',#23648,#23649,#5051,.T.);
#30154=EDGE_CURVE('',#23649,#23355,#5052,.T.);
#30155=EDGE_CURVE('',#23276,#23354,#5053,.T.);
#30156=EDGE_CURVE('',#23275,#23650,#5054,.T.);
#30157=EDGE_CURVE('',#23412,#23650,#5055,.T.);
#30158=EDGE_CURVE('',#23651,#23409,#5056,.T.);
#30159=EDGE_CURVE('',#23651,#23647,#19494,.T.);
#30160=EDGE_CURVE('',#23652,#23407,#5057,.T.);
#30161=EDGE_CURVE('',#23652,#23653,#19495,.T.);
#30162=EDGE_CURVE('',#23653,#23654,#5058,.T.);
#30163=EDGE_CURVE('',#23654,#23359,#5059,.T.);
#30164=EDGE_CURVE('',#23272,#23358,#5060,.T.);
#30165=EDGE_CURVE('',#23271,#23655,#5061,.T.);
#30166=EDGE_CURVE('',#23408,#23655,#5062,.T.);
#30167=EDGE_CURVE('',#23656,#23405,#5063,.T.);
#30168=EDGE_CURVE('',#23656,#23652,#19496,.T.);
#30169=EDGE_CURVE('',#23657,#23403,#5064,.T.);
#30170=EDGE_CURVE('',#23657,#23658,#19497,.T.);
#30171=EDGE_CURVE('',#23658,#23659,#5065,.T.);
#30172=EDGE_CURVE('',#23659,#23363,#5066,.T.);
#30173=EDGE_CURVE('',#23268,#23362,#5067,.T.);
#30174=EDGE_CURVE('',#23267,#23660,#5068,.T.);
#30175=EDGE_CURVE('',#23404,#23660,#5069,.T.);
#30176=EDGE_CURVE('',#23661,#23401,#5070,.T.);
#30177=EDGE_CURVE('',#23661,#23657,#19498,.T.);
#30178=EDGE_CURVE('',#23662,#23399,#5071,.T.);
#30179=EDGE_CURVE('',#23662,#23663,#19499,.T.);
#30180=EDGE_CURVE('',#23663,#23664,#5072,.T.);
#30181=EDGE_CURVE('',#23664,#23367,#5073,.T.);
#30182=EDGE_CURVE('',#23264,#23366,#5074,.T.);
#30183=EDGE_CURVE('',#23263,#23665,#5075,.T.);
#30184=EDGE_CURVE('',#23400,#23665,#5076,.T.);
#30185=EDGE_CURVE('',#23666,#23397,#5077,.T.);
#30186=EDGE_CURVE('',#23666,#23662,#19500,.T.);
#30187=EDGE_CURVE('',#23667,#23395,#5078,.T.);
#30188=EDGE_CURVE('',#23667,#23668,#19501,.T.);
#30189=EDGE_CURVE('',#23668,#23669,#5079,.T.);
#30190=EDGE_CURVE('',#23669,#23371,#5080,.T.);
#30191=EDGE_CURVE('',#23260,#23370,#5081,.T.);
#30192=EDGE_CURVE('',#23259,#23670,#5082,.T.);
#30193=EDGE_CURVE('',#23396,#23670,#5083,.T.);
#30194=EDGE_CURVE('',#23671,#23393,#5084,.T.);
#30195=EDGE_CURVE('',#23671,#23667,#19502,.T.);
#30196=EDGE_CURVE('',#23672,#23391,#5085,.T.);
#30197=EDGE_CURVE('',#23672,#23673,#19503,.T.);
#30198=EDGE_CURVE('',#23673,#23674,#5086,.T.);
#30199=EDGE_CURVE('',#23674,#23375,#5087,.T.);
#30200=EDGE_CURVE('',#23256,#23374,#5088,.T.);
#30201=EDGE_CURVE('',#23255,#23675,#5089,.T.);
#30202=EDGE_CURVE('',#23392,#23675,#5090,.T.);
#30203=EDGE_CURVE('',#23676,#23389,#5091,.T.);
#30204=EDGE_CURVE('',#23676,#23672,#19504,.T.);
#30205=EDGE_CURVE('',#23677,#23387,#5092,.T.);
#30206=EDGE_CURVE('',#23677,#23678,#19505,.T.);
#30207=EDGE_CURVE('',#23678,#23679,#5093,.T.);
#30208=EDGE_CURVE('',#23679,#23379,#5094,.T.);
#30209=EDGE_CURVE('',#23252,#23378,#5095,.T.);
#30210=EDGE_CURVE('',#23251,#23680,#5096,.T.);
#30211=EDGE_CURVE('',#23388,#23680,#5097,.T.);
#30212=EDGE_CURVE('',#23681,#23385,#5098,.T.);
#30213=EDGE_CURVE('',#23681,#23677,#19506,.T.);
#30214=EDGE_CURVE('',#23682,#23681,#19507,.T.);
#30215=EDGE_CURVE('',#23678,#23682,#19855,.T.);
#30216=EDGE_CURVE('',#23683,#23676,#19508,.T.);
#30217=EDGE_CURVE('',#23673,#23683,#19856,.T.);
#30218=EDGE_CURVE('',#23684,#23671,#19509,.T.);
#30219=EDGE_CURVE('',#23668,#23684,#19857,.T.);
#30220=EDGE_CURVE('',#23685,#23666,#19510,.T.);
#30221=EDGE_CURVE('',#23663,#23685,#19858,.T.);
#30222=EDGE_CURVE('',#23686,#23661,#19511,.T.);
#30223=EDGE_CURVE('',#23658,#23686,#19859,.T.);
#30224=EDGE_CURVE('',#23687,#23656,#19512,.T.);
#30225=EDGE_CURVE('',#23653,#23687,#19860,.T.);
#30226=EDGE_CURVE('',#23688,#23651,#19513,.T.);
#30227=EDGE_CURVE('',#23648,#23688,#19861,.T.);
#30228=EDGE_CURVE('',#23689,#23646,#19514,.T.);
#30229=EDGE_CURVE('',#23643,#23689,#19862,.T.);
#30230=EDGE_CURVE('',#23690,#23641,#19515,.T.);
#30231=EDGE_CURVE('',#23638,#23690,#19863,.T.);
#30232=EDGE_CURVE('',#23691,#23636,#19516,.T.);
#30233=EDGE_CURVE('',#23633,#23691,#19864,.T.);
#30234=EDGE_CURVE('',#23692,#23631,#19517,.T.);
#30235=EDGE_CURVE('',#23628,#23692,#19865,.T.);
#30236=EDGE_CURVE('',#23693,#23626,#19518,.T.);
#30237=EDGE_CURVE('',#23623,#23693,#19866,.T.);
#30238=EDGE_CURVE('',#23694,#23621,#19519,.T.);
#30239=EDGE_CURVE('',#23618,#23694,#19867,.T.);
#30240=EDGE_CURVE('',#23695,#23616,#19520,.T.);
#30241=EDGE_CURVE('',#23613,#23695,#19868,.T.);
#30242=EDGE_CURVE('',#23696,#23611,#19521,.T.);
#30243=EDGE_CURVE('',#23608,#23696,#19869,.T.);
#30244=EDGE_CURVE('',#23697,#23606,#19522,.T.);
#30245=EDGE_CURVE('',#23603,#23697,#19870,.T.);
#30246=EDGE_CURVE('',#23698,#23601,#19523,.T.);
#30247=EDGE_CURVE('',#23598,#23698,#19871,.T.);
#30248=EDGE_CURVE('',#23699,#23596,#19524,.T.);
#30249=EDGE_CURVE('',#23593,#23699,#19872,.T.);
#30250=EDGE_CURVE('',#23700,#23591,#19525,.T.);
#30251=EDGE_CURVE('',#23588,#23700,#19873,.T.);
#30252=EDGE_CURVE('',#23701,#23586,#19526,.T.);
#30253=EDGE_CURVE('',#23583,#23701,#19874,.T.);
#30254=EDGE_CURVE('',#23702,#23581,#19527,.T.);
#30255=EDGE_CURVE('',#23578,#23702,#19875,.T.);
#30256=EDGE_CURVE('',#23703,#23576,#19528,.T.);
#30257=EDGE_CURVE('',#23573,#23703,#19876,.T.);
#30258=EDGE_CURVE('',#23704,#23571,#19529,.T.);
#30259=EDGE_CURVE('',#23568,#23704,#19877,.T.);
#30260=EDGE_CURVE('',#23705,#23566,#19530,.T.);
#30261=EDGE_CURVE('',#23563,#23705,#19878,.T.);
#30262=EDGE_CURVE('',#23706,#23561,#19531,.T.);
#30263=EDGE_CURVE('',#23558,#23706,#19879,.T.);
#30264=EDGE_CURVE('',#23707,#23556,#19532,.T.);
#30265=EDGE_CURVE('',#23553,#23707,#19880,.T.);
#30266=EDGE_CURVE('',#23708,#23551,#19533,.T.);
#30267=EDGE_CURVE('',#23548,#23708,#19881,.T.);
#30268=EDGE_CURVE('',#23709,#23546,#19534,.T.);
#30269=EDGE_CURVE('',#23543,#23709,#19882,.T.);
#30270=EDGE_CURVE('',#23710,#23541,#19535,.T.);
#30271=EDGE_CURVE('',#23538,#23710,#19883,.T.);
#30272=EDGE_CURVE('',#23711,#23536,#19536,.T.);
#30273=EDGE_CURVE('',#23533,#23711,#19884,.T.);
#30274=EDGE_CURVE('',#23712,#23531,#19537,.T.);
#30275=EDGE_CURVE('',#23528,#23712,#19885,.T.);
#30276=EDGE_CURVE('',#23713,#23526,#19538,.T.);
#30277=EDGE_CURVE('',#23523,#23713,#19886,.T.);
#30278=EDGE_CURVE('',#23714,#23521,#19539,.T.);
#30279=EDGE_CURVE('',#23518,#23714,#19887,.T.);
#30280=EDGE_CURVE('',#23715,#23514,#5099,.T.);
#30281=EDGE_CURVE('',#23333,#23715,#5100,.T.);
#30282=EDGE_CURVE('',#23202,#23332,#5101,.T.);
#30283=EDGE_CURVE('',#23716,#23201,#5102,.T.);
#30284=EDGE_CURVE('',#23716,#23714,#5103,.T.);
#30285=EDGE_CURVE('',#23717,#23510,#5104,.T.);
#30286=EDGE_CURVE('',#23329,#23717,#5105,.T.);
#30287=EDGE_CURVE('',#23206,#23328,#5106,.T.);
#30288=EDGE_CURVE('',#23718,#23205,#5107,.T.);
#30289=EDGE_CURVE('',#23718,#23713,#5108,.T.);
#30290=EDGE_CURVE('',#23719,#23506,#5109,.T.);
#30291=EDGE_CURVE('',#23325,#23719,#5110,.T.);
#30292=EDGE_CURVE('',#23210,#23324,#5111,.T.);
#30293=EDGE_CURVE('',#23720,#23209,#5112,.T.);
#30294=EDGE_CURVE('',#23720,#23712,#5113,.T.);
#30295=EDGE_CURVE('',#23721,#23502,#5114,.T.);
#30296=EDGE_CURVE('',#23321,#23721,#5115,.T.);
#30297=EDGE_CURVE('',#23214,#23320,#5116,.T.);
#30298=EDGE_CURVE('',#23722,#23213,#5117,.T.);
#30299=EDGE_CURVE('',#23722,#23711,#5118,.T.);
#30300=EDGE_CURVE('',#23723,#23498,#5119,.T.);
#30301=EDGE_CURVE('',#23317,#23723,#5120,.T.);
#30302=EDGE_CURVE('',#23218,#23316,#5121,.T.);
#30303=EDGE_CURVE('',#23724,#23217,#5122,.T.);
#30304=EDGE_CURVE('',#23724,#23710,#5123,.T.);
#30305=EDGE_CURVE('',#23725,#23494,#5124,.T.);
#30306=EDGE_CURVE('',#23313,#23725,#5125,.T.);
#30307=EDGE_CURVE('',#23222,#23312,#5126,.T.);
#30308=EDGE_CURVE('',#23726,#23221,#5127,.T.);
#30309=EDGE_CURVE('',#23726,#23709,#5128,.T.);
#30310=EDGE_CURVE('',#23727,#23490,#5129,.T.);
#30311=EDGE_CURVE('',#23309,#23727,#5130,.T.);
#30312=EDGE_CURVE('',#23226,#23308,#5131,.T.);
#30313=EDGE_CURVE('',#23728,#23225,#5132,.T.);
#30314=EDGE_CURVE('',#23728,#23708,#5133,.T.);
#30315=EDGE_CURVE('',#23729,#23486,#5134,.T.);
#30316=EDGE_CURVE('',#23305,#23729,#5135,.T.);
#30317=EDGE_CURVE('',#23230,#23304,#5136,.T.);
#30318=EDGE_CURVE('',#23730,#23229,#5137,.T.);
#30319=EDGE_CURVE('',#23730,#23707,#5138,.T.);
#30320=EDGE_CURVE('',#23731,#23482,#5139,.T.);
#30321=EDGE_CURVE('',#23301,#23731,#5140,.T.);
#30322=EDGE_CURVE('',#23234,#23300,#5141,.T.);
#30323=EDGE_CURVE('',#23732,#23233,#5142,.T.);
#30324=EDGE_CURVE('',#23732,#23706,#5143,.T.);
#30325=EDGE_CURVE('',#23733,#23478,#5144,.T.);
#30326=EDGE_CURVE('',#23297,#23733,#5145,.T.);
#30327=EDGE_CURVE('',#23238,#23296,#5146,.T.);
#30328=EDGE_CURVE('',#23734,#23237,#5147,.T.);
#30329=EDGE_CURVE('',#23734,#23705,#5148,.T.);
#30330=EDGE_CURVE('',#23735,#23474,#5149,.T.);
#30331=EDGE_CURVE('',#23293,#23735,#5150,.T.);
#30332=EDGE_CURVE('',#23736,#23241,#5151,.T.);
#30333=EDGE_CURVE('',#23736,#23704,#5152,.T.);
#30334=EDGE_CURVE('',#23737,#23470,#5153,.T.);
#30335=EDGE_CURVE('',#23141,#23737,#5154,.T.);
#30336=EDGE_CURVE('',#23156,#23140,#5155,.T.);
#30337=EDGE_CURVE('',#23738,#23155,#5156,.T.);
#30338=EDGE_CURVE('',#23738,#23703,#5157,.T.);
#30339=EDGE_CURVE('',#23739,#23466,#5158,.T.);
#30340=EDGE_CURVE('',#23137,#23739,#5159,.T.);
#30341=EDGE_CURVE('',#23160,#23136,#5160,.T.);
#30342=EDGE_CURVE('',#23740,#23159,#5161,.T.);
#30343=EDGE_CURVE('',#23740,#23702,#5162,.T.);
#30344=EDGE_CURVE('',#23741,#23462,#5163,.T.);
#30345=EDGE_CURVE('',#23133,#23741,#5164,.T.);
#30346=EDGE_CURVE('',#23164,#23132,#5165,.T.);
#30347=EDGE_CURVE('',#23742,#23163,#5166,.T.);
#30348=EDGE_CURVE('',#23742,#23701,#5167,.T.);
#30349=EDGE_CURVE('',#23743,#23458,#5168,.T.);
#30350=EDGE_CURVE('',#23129,#23743,#5169,.T.);
#30351=EDGE_CURVE('',#23168,#23128,#5170,.T.);
#30352=EDGE_CURVE('',#23744,#23167,#5171,.T.);
#30353=EDGE_CURVE('',#23744,#23700,#5172,.T.);
#30354=EDGE_CURVE('',#23745,#23454,#5173,.T.);
#30355=EDGE_CURVE('',#23125,#23745,#5174,.T.);
#30356=EDGE_CURVE('',#23172,#23124,#5175,.T.);
#30357=EDGE_CURVE('',#23746,#23171,#5176,.T.);
#30358=EDGE_CURVE('',#23746,#23699,#5177,.T.);
#30359=EDGE_CURVE('',#23747,#23450,#5178,.T.);
#30360=EDGE_CURVE('',#23121,#23747,#5179,.T.);
#30361=EDGE_CURVE('',#23176,#23120,#5180,.T.);
#30362=EDGE_CURVE('',#23748,#23175,#5181,.T.);
#30363=EDGE_CURVE('',#23748,#23698,#5182,.T.);
#30364=EDGE_CURVE('',#23749,#23446,#5183,.T.);
#30365=EDGE_CURVE('',#23117,#23749,#5184,.T.);
#30366=EDGE_CURVE('',#23180,#23116,#5185,.T.);
#30367=EDGE_CURVE('',#23750,#23179,#5186,.T.);
#30368=EDGE_CURVE('',#23750,#23697,#5187,.T.);
#30369=EDGE_CURVE('',#23751,#23442,#5188,.T.);
#30370=EDGE_CURVE('',#23113,#23751,#5189,.T.);
#30371=EDGE_CURVE('',#23184,#23112,#5190,.T.);
#30372=EDGE_CURVE('',#23752,#23183,#5191,.T.);
#30373=EDGE_CURVE('',#23752,#23696,#5192,.T.);
#30374=EDGE_CURVE('',#23753,#23438,#5193,.T.);
#30375=EDGE_CURVE('',#23109,#23753,#5194,.T.);
#30376=EDGE_CURVE('',#23188,#23108,#5195,.T.);
#30377=EDGE_CURVE('',#23754,#23187,#5196,.T.);
#30378=EDGE_CURVE('',#23754,#23695,#5197,.T.);
#30379=EDGE_CURVE('',#23755,#23434,#5198,.T.);
#30380=EDGE_CURVE('',#23105,#23755,#5199,.T.);
#30381=EDGE_CURVE('',#23192,#23104,#5200,.T.);
#30382=EDGE_CURVE('',#23756,#23191,#5201,.T.);
#30383=EDGE_CURVE('',#23756,#23694,#5202,.T.);
#30384=EDGE_CURVE('',#23757,#23430,#5203,.T.);
#30385=EDGE_CURVE('',#23101,#23757,#5204,.T.);
#30386=EDGE_CURVE('',#23758,#23195,#5205,.T.);
#30387=EDGE_CURVE('',#23758,#23693,#5206,.T.);
#30388=EDGE_CURVE('',#23759,#23426,#5207,.T.);
#30389=EDGE_CURVE('',#23290,#23759,#5208,.T.);
#30390=EDGE_CURVE('',#23341,#23289,#5209,.T.);
#30391=EDGE_CURVE('',#23760,#23340,#5210,.T.);
#30392=EDGE_CURVE('',#23760,#23692,#5211,.T.);
#30393=EDGE_CURVE('',#23761,#23422,#5212,.T.);
#30394=EDGE_CURVE('',#23286,#23761,#5213,.T.);
#30395=EDGE_CURVE('',#23345,#23285,#5214,.T.);
#30396=EDGE_CURVE('',#23762,#23344,#5215,.T.);
#30397=EDGE_CURVE('',#23762,#23691,#5216,.T.);
#30398=EDGE_CURVE('',#23763,#23418,#5217,.T.);
#30399=EDGE_CURVE('',#23282,#23763,#5218,.T.);
#30400=EDGE_CURVE('',#23349,#23281,#5219,.T.);
#30401=EDGE_CURVE('',#23764,#23348,#5220,.T.);
#30402=EDGE_CURVE('',#23764,#23690,#5221,.T.);
#30403=EDGE_CURVE('',#23765,#23414,#5222,.T.);
#30404=EDGE_CURVE('',#23278,#23765,#5223,.T.);
#30405=EDGE_CURVE('',#23353,#23277,#5224,.T.);
#30406=EDGE_CURVE('',#23766,#23352,#5225,.T.);
#30407=EDGE_CURVE('',#23766,#23689,#5226,.T.);
#30408=EDGE_CURVE('',#23767,#23410,#5227,.T.);
#30409=EDGE_CURVE('',#23274,#23767,#5228,.T.);
#30410=EDGE_CURVE('',#23357,#23273,#5229,.T.);
#30411=EDGE_CURVE('',#23768,#23356,#5230,.T.);
#30412=EDGE_CURVE('',#23768,#23688,#5231,.T.);
#30413=EDGE_CURVE('',#23769,#23406,#5232,.T.);
#30414=EDGE_CURVE('',#23270,#23769,#5233,.T.);
#30415=EDGE_CURVE('',#23361,#23269,#5234,.T.);
#30416=EDGE_CURVE('',#23770,#23360,#5235,.T.);
#30417=EDGE_CURVE('',#23770,#23687,#5236,.T.);
#30418=EDGE_CURVE('',#23771,#23402,#5237,.T.);
#30419=EDGE_CURVE('',#23266,#23771,#5238,.T.);
#30420=EDGE_CURVE('',#23365,#23265,#5239,.T.);
#30421=EDGE_CURVE('',#23772,#23364,#5240,.T.);
#30422=EDGE_CURVE('',#23772,#23686,#5241,.T.);
#30423=EDGE_CURVE('',#23773,#23398,#5242,.T.);
#30424=EDGE_CURVE('',#23262,#23773,#5243,.T.);
#30425=EDGE_CURVE('',#23369,#23261,#5244,.T.);
#30426=EDGE_CURVE('',#23774,#23368,#5245,.T.);
#30427=EDGE_CURVE('',#23774,#23685,#5246,.T.);
#30428=EDGE_CURVE('',#23775,#23394,#5247,.T.);
#30429=EDGE_CURVE('',#23258,#23775,#5248,.T.);
#30430=EDGE_CURVE('',#23373,#23257,#5249,.T.);
#30431=EDGE_CURVE('',#23776,#23372,#5250,.T.);
#30432=EDGE_CURVE('',#23776,#23684,#5251,.T.);
#30433=EDGE_CURVE('',#23777,#23390,#5252,.T.);
#30434=EDGE_CURVE('',#23254,#23777,#5253,.T.);
#30435=EDGE_CURVE('',#23377,#23253,#5254,.T.);
#30436=EDGE_CURVE('',#23778,#23376,#5255,.T.);
#30437=EDGE_CURVE('',#23778,#23683,#5256,.T.);
#30438=EDGE_CURVE('',#23779,#23386,#5257,.T.);
#30439=EDGE_CURVE('',#23250,#23779,#5258,.T.);
#30440=EDGE_CURVE('',#23780,#23380,#5259,.T.);
#30441=EDGE_CURVE('',#23780,#23682,#5260,.T.);
#30442=EDGE_CURVE('',#23519,#23716,#5261,.T.);
#30443=EDGE_CURVE('',#23520,#23715,#5262,.T.);
#30444=EDGE_CURVE('',#23524,#23718,#5263,.T.);
#30445=EDGE_CURVE('',#23525,#23717,#5264,.T.);
#30446=EDGE_CURVE('',#23529,#23720,#5265,.T.);
#30447=EDGE_CURVE('',#23530,#23719,#5266,.T.);
#30448=EDGE_CURVE('',#23534,#23722,#5267,.T.);
#30449=EDGE_CURVE('',#23535,#23721,#5268,.T.);
#30450=EDGE_CURVE('',#23539,#23724,#5269,.T.);
#30451=EDGE_CURVE('',#23540,#23723,#5270,.T.);
#30452=EDGE_CURVE('',#23544,#23726,#5271,.T.);
#30453=EDGE_CURVE('',#23545,#23725,#5272,.T.);
#30454=EDGE_CURVE('',#23549,#23728,#5273,.T.);
#30455=EDGE_CURVE('',#23550,#23727,#5274,.T.);
#30456=EDGE_CURVE('',#23554,#23730,#5275,.T.);
#30457=EDGE_CURVE('',#23555,#23729,#5276,.T.);
#30458=EDGE_CURVE('',#23559,#23732,#5277,.T.);
#30459=EDGE_CURVE('',#23560,#23731,#5278,.T.);
#30460=EDGE_CURVE('',#23564,#23734,#5279,.T.);
#30461=EDGE_CURVE('',#23565,#23733,#5280,.T.);
#30462=EDGE_CURVE('',#23569,#23736,#5281,.T.);
#30463=EDGE_CURVE('',#23570,#23735,#5282,.T.);
#30464=EDGE_CURVE('',#23574,#23738,#5283,.T.);
#30465=EDGE_CURVE('',#23575,#23737,#5284,.T.);
#30466=EDGE_CURVE('',#23579,#23740,#5285,.T.);
#30467=EDGE_CURVE('',#23580,#23739,#5286,.T.);
#30468=EDGE_CURVE('',#23584,#23742,#5287,.T.);
#30469=EDGE_CURVE('',#23585,#23741,#5288,.T.);
#30470=EDGE_CURVE('',#23589,#23744,#5289,.T.);
#30471=EDGE_CURVE('',#23590,#23743,#5290,.T.);
#30472=EDGE_CURVE('',#23594,#23746,#5291,.T.);
#30473=EDGE_CURVE('',#23595,#23745,#5292,.T.);
#30474=EDGE_CURVE('',#23599,#23748,#5293,.T.);
#30475=EDGE_CURVE('',#23600,#23747,#5294,.T.);
#30476=EDGE_CURVE('',#23604,#23750,#5295,.T.);
#30477=EDGE_CURVE('',#23605,#23749,#5296,.T.);
#30478=EDGE_CURVE('',#23609,#23752,#5297,.T.);
#30479=EDGE_CURVE('',#23610,#23751,#5298,.T.);
#30480=EDGE_CURVE('',#23614,#23754,#5299,.T.);
#30481=EDGE_CURVE('',#23615,#23753,#5300,.T.);
#30482=EDGE_CURVE('',#23619,#23756,#5301,.T.);
#30483=EDGE_CURVE('',#23620,#23755,#5302,.T.);
#30484=EDGE_CURVE('',#23624,#23758,#5303,.T.);
#30485=EDGE_CURVE('',#23625,#23757,#5304,.T.);
#30486=EDGE_CURVE('',#23629,#23760,#5305,.T.);
#30487=EDGE_CURVE('',#23630,#23759,#5306,.T.);
#30488=EDGE_CURVE('',#23634,#23762,#5307,.T.);
#30489=EDGE_CURVE('',#23635,#23761,#5308,.T.);
#30490=EDGE_CURVE('',#23639,#23764,#5309,.T.);
#30491=EDGE_CURVE('',#23640,#23763,#5310,.T.);
#30492=EDGE_CURVE('',#23644,#23766,#5311,.T.);
#30493=EDGE_CURVE('',#23645,#23765,#5312,.T.);
#30494=EDGE_CURVE('',#23649,#23768,#5313,.T.);
#30495=EDGE_CURVE('',#23650,#23767,#5314,.T.);
#30496=EDGE_CURVE('',#23654,#23770,#5315,.T.);
#30497=EDGE_CURVE('',#23655,#23769,#5316,.T.);
#30498=EDGE_CURVE('',#23659,#23772,#5317,.T.);
#30499=EDGE_CURVE('',#23660,#23771,#5318,.T.);
#30500=EDGE_CURVE('',#23664,#23774,#5319,.T.);
#30501=EDGE_CURVE('',#23665,#23773,#5320,.T.);
#30502=EDGE_CURVE('',#23669,#23776,#5321,.T.);
#30503=EDGE_CURVE('',#23670,#23775,#5322,.T.);
#30504=EDGE_CURVE('',#23674,#23778,#5323,.T.);
#30505=EDGE_CURVE('',#23675,#23777,#5324,.T.);
#30506=EDGE_CURVE('',#23679,#23780,#5325,.T.);
#30507=EDGE_CURVE('',#23680,#23779,#5326,.T.);
#30508=EDGE_CURVE('',#23781,#23782,#19888,.T.);
#30509=EDGE_CURVE('',#23782,#23783,#19889,.T.);
#30510=EDGE_CURVE('',#23783,#23783,#19890,.T.);
#30511=EDGE_CURVE('',#23782,#23781,#19891,.T.);
#30512=EDGE_CURVE('',#23784,#23784,#19892,.T.);
#30513=EDGE_CURVE('',#23785,#23785,#19893,.T.);
#30514=EDGE_CURVE('',#23785,#23781,#5327,.T.);
#30515=EDGE_CURVE('',#23786,#23786,#19894,.T.);
#30516=EDGE_CURVE('',#23786,#23787,#19895,.T.);
#30517=EDGE_CURVE('',#23787,#23788,#19896,.T.);
#30518=EDGE_CURVE('',#23788,#23787,#19897,.T.);
#30519=EDGE_CURVE('',#23789,#23789,#19898,.T.);
#30520=EDGE_CURVE('',#23788,#23152,#5328,.T.);
#30521=EDGE_CURVE('',#23784,#23790,#19899,.T.);
#30522=EDGE_CURVE('',#23790,#23791,#19900,.T.);
#30523=EDGE_CURVE('',#23791,#23790,#19901,.T.);
#30524=EDGE_CURVE('',#23792,#23792,#19902,.T.);
#30525=EDGE_CURVE('',#23792,#23791,#5329,.T.);
#30526=EDGE_CURVE('',#23793,#23794,#19903,.T.);
#30527=EDGE_CURVE('',#23794,#23789,#19904,.T.);
#30528=EDGE_CURVE('',#23794,#23793,#19905,.T.);
#30529=EDGE_CURVE('',#23793,#23795,#5330,.T.);
#30530=EDGE_CURVE('',#23795,#23795,#19906,.T.);
#30531=EDGE_CURVE('',#23796,#23796,#19907,.T.);
#30532=EDGE_CURVE('',#23796,#23797,#5331,.T.);
#30533=EDGE_CURVE('',#23797,#23797,#19908,.T.);
#30534=EDGE_CURVE('',#23797,#23798,#5332,.T.);
#30535=EDGE_CURVE('',#23798,#23798,#19909,.T.);
#30536=EDGE_CURVE('',#23799,#23799,#19910,.T.);
#30537=EDGE_CURVE('',#23799,#23796,#5333,.T.);
#41203=ORIENTED_EDGE('',*,*,#29463,.F.);
#41204=ORIENTED_EDGE('',*,*,#29464,.F.);
#41205=ORIENTED_EDGE('',*,*,#29465,.F.);
#41206=ORIENTED_EDGE('',*,*,#29466,.F.);
#41207=ORIENTED_EDGE('',*,*,#29467,.F.);
#41208=ORIENTED_EDGE('',*,*,#29468,.F.);
#41209=ORIENTED_EDGE('',*,*,#29469,.F.);
#41210=ORIENTED_EDGE('',*,*,#29470,.F.);
#41211=ORIENTED_EDGE('',*,*,#29471,.F.);
#41212=ORIENTED_EDGE('',*,*,#29472,.F.);
#41213=ORIENTED_EDGE('',*,*,#29473,.T.);
#41214=ORIENTED_EDGE('',*,*,#29474,.F.);
#41215=ORIENTED_EDGE('',*,*,#29475,.F.);
#41216=ORIENTED_EDGE('',*,*,#29465,.T.);
#41217=ORIENTED_EDGE('',*,*,#29476,.F.);
#41218=ORIENTED_EDGE('',*,*,#29473,.F.);
#41219=ORIENTED_EDGE('',*,*,#29468,.T.);
#41220=ORIENTED_EDGE('',*,*,#29477,.T.);
#41221=ORIENTED_EDGE('',*,*,#29478,.T.);
#41222=ORIENTED_EDGE('',*,*,#29479,.F.);
#41223=ORIENTED_EDGE('',*,*,#29469,.T.);
#41224=ORIENTED_EDGE('',*,*,#29480,.F.);
#41225=ORIENTED_EDGE('',*,*,#29481,.T.);
#41226=ORIENTED_EDGE('',*,*,#29482,.T.);
#41227=ORIENTED_EDGE('',*,*,#29483,.T.);
#41228=ORIENTED_EDGE('',*,*,#29484,.T.);
#41229=ORIENTED_EDGE('',*,*,#29485,.T.);
#41230=ORIENTED_EDGE('',*,*,#29486,.T.);
#41231=ORIENTED_EDGE('',*,*,#29487,.T.);
#41232=ORIENTED_EDGE('',*,*,#29488,.T.);
#41233=ORIENTED_EDGE('',*,*,#29489,.T.);
#41234=ORIENTED_EDGE('',*,*,#29490,.T.);
#41235=ORIENTED_EDGE('',*,*,#29491,.T.);
#41236=ORIENTED_EDGE('',*,*,#29492,.T.);
#41237=ORIENTED_EDGE('',*,*,#29493,.T.);
#41238=ORIENTED_EDGE('',*,*,#29494,.T.);
#41239=ORIENTED_EDGE('',*,*,#29495,.T.);
#41240=ORIENTED_EDGE('',*,*,#29496,.T.);
#41241=ORIENTED_EDGE('',*,*,#29497,.T.);
#41242=ORIENTED_EDGE('',*,*,#29498,.T.);
#41243=ORIENTED_EDGE('',*,*,#29499,.T.);
#41244=ORIENTED_EDGE('',*,*,#29500,.T.);
#41245=ORIENTED_EDGE('',*,*,#29501,.T.);
#41246=ORIENTED_EDGE('',*,*,#29502,.T.);
#41247=ORIENTED_EDGE('',*,*,#29503,.T.);
#41248=ORIENTED_EDGE('',*,*,#29504,.T.);
#41249=ORIENTED_EDGE('',*,*,#29505,.T.);
#41250=ORIENTED_EDGE('',*,*,#29506,.T.);
#41251=ORIENTED_EDGE('',*,*,#29507,.T.);
#41252=ORIENTED_EDGE('',*,*,#29508,.T.);
#41253=ORIENTED_EDGE('',*,*,#29509,.T.);
#41254=ORIENTED_EDGE('',*,*,#29510,.T.);
#41255=ORIENTED_EDGE('',*,*,#29511,.T.);
#41256=ORIENTED_EDGE('',*,*,#29512,.T.);
#41257=ORIENTED_EDGE('',*,*,#29513,.T.);
#41258=ORIENTED_EDGE('',*,*,#29514,.T.);
#41259=ORIENTED_EDGE('',*,*,#29515,.T.);
#41260=ORIENTED_EDGE('',*,*,#29516,.T.);
#41261=ORIENTED_EDGE('',*,*,#29517,.T.);
#41262=ORIENTED_EDGE('',*,*,#29518,.T.);
#41263=ORIENTED_EDGE('',*,*,#29519,.T.);
#41264=ORIENTED_EDGE('',*,*,#29520,.T.);
#41265=ORIENTED_EDGE('',*,*,#29521,.T.);
#41266=ORIENTED_EDGE('',*,*,#29522,.T.);
#41267=ORIENTED_EDGE('',*,*,#29523,.T.);
#41268=ORIENTED_EDGE('',*,*,#29524,.T.);
#41269=ORIENTED_EDGE('',*,*,#29525,.T.);
#41270=ORIENTED_EDGE('',*,*,#29526,.T.);
#41271=ORIENTED_EDGE('',*,*,#29466,.T.);
#41272=ORIENTED_EDGE('',*,*,#29475,.T.);
#41273=ORIENTED_EDGE('',*,*,#29472,.T.);
#41274=ORIENTED_EDGE('',*,*,#29527,.F.);
#41275=ORIENTED_EDGE('',*,*,#29528,.T.);
#41276=ORIENTED_EDGE('',*,*,#29529,.T.);
#41277=ORIENTED_EDGE('',*,*,#29530,.T.);
#41278=ORIENTED_EDGE('',*,*,#29531,.F.);
#41279=ORIENTED_EDGE('',*,*,#29532,.T.);
#41280=ORIENTED_EDGE('',*,*,#29533,.T.);
#41281=ORIENTED_EDGE('',*,*,#29534,.T.);
#41282=ORIENTED_EDGE('',*,*,#29535,.F.);
#41283=ORIENTED_EDGE('',*,*,#29536,.T.);
#41284=ORIENTED_EDGE('',*,*,#29471,.T.);
#41285=ORIENTED_EDGE('',*,*,#29537,.F.);
#41286=ORIENTED_EDGE('',*,*,#29538,.T.);
#41287=ORIENTED_EDGE('',*,*,#29539,.T.);
#41288=ORIENTED_EDGE('',*,*,#29540,.T.);
#41289=ORIENTED_EDGE('',*,*,#29541,.F.);
#41290=ORIENTED_EDGE('',*,*,#29542,.T.);
#41291=ORIENTED_EDGE('',*,*,#29543,.T.);
#41292=ORIENTED_EDGE('',*,*,#29544,.T.);
#41293=ORIENTED_EDGE('',*,*,#29545,.F.);
#41294=ORIENTED_EDGE('',*,*,#29546,.T.);
#41295=ORIENTED_EDGE('',*,*,#29547,.T.);
#41296=ORIENTED_EDGE('',*,*,#29548,.T.);
#41297=ORIENTED_EDGE('',*,*,#29549,.F.);
#41298=ORIENTED_EDGE('',*,*,#29550,.T.);
#41299=ORIENTED_EDGE('',*,*,#29551,.T.);
#41300=ORIENTED_EDGE('',*,*,#29552,.T.);
#41301=ORIENTED_EDGE('',*,*,#29553,.F.);
#41302=ORIENTED_EDGE('',*,*,#29554,.T.);
#41303=ORIENTED_EDGE('',*,*,#29555,.T.);
#41304=ORIENTED_EDGE('',*,*,#29556,.T.);
#41305=ORIENTED_EDGE('',*,*,#29557,.F.);
#41306=ORIENTED_EDGE('',*,*,#29558,.T.);
#41307=ORIENTED_EDGE('',*,*,#29559,.T.);
#41308=ORIENTED_EDGE('',*,*,#29560,.T.);
#41309=ORIENTED_EDGE('',*,*,#29561,.F.);
#41310=ORIENTED_EDGE('',*,*,#29562,.T.);
#41311=ORIENTED_EDGE('',*,*,#29563,.T.);
#41312=ORIENTED_EDGE('',*,*,#29564,.T.);
#41313=ORIENTED_EDGE('',*,*,#29565,.F.);
#41314=ORIENTED_EDGE('',*,*,#29566,.T.);
#41315=ORIENTED_EDGE('',*,*,#29567,.T.);
#41316=ORIENTED_EDGE('',*,*,#29568,.T.);
#41317=ORIENTED_EDGE('',*,*,#29569,.F.);
#41318=ORIENTED_EDGE('',*,*,#29570,.T.);
#41319=ORIENTED_EDGE('',*,*,#29571,.T.);
#41320=ORIENTED_EDGE('',*,*,#29572,.T.);
#41321=ORIENTED_EDGE('',*,*,#29573,.F.);
#41322=ORIENTED_EDGE('',*,*,#29574,.T.);
#41323=ORIENTED_EDGE('',*,*,#29575,.T.);
#41324=ORIENTED_EDGE('',*,*,#29576,.T.);
#41325=ORIENTED_EDGE('',*,*,#29577,.F.);
#41326=ORIENTED_EDGE('',*,*,#29578,.T.);
#41327=ORIENTED_EDGE('',*,*,#29579,.T.);
#41328=ORIENTED_EDGE('',*,*,#29580,.T.);
#41329=ORIENTED_EDGE('',*,*,#29581,.F.);
#41330=ORIENTED_EDGE('',*,*,#29582,.T.);
#41331=ORIENTED_EDGE('',*,*,#29527,.T.);
#41332=ORIENTED_EDGE('',*,*,#29467,.T.);
#41333=ORIENTED_EDGE('',*,*,#29535,.T.);
#41334=ORIENTED_EDGE('',*,*,#29583,.T.);
#41335=ORIENTED_EDGE('',*,*,#29584,.F.);
#41336=ORIENTED_EDGE('',*,*,#29585,.T.);
#41337=ORIENTED_EDGE('',*,*,#29586,.T.);
#41338=ORIENTED_EDGE('',*,*,#29587,.T.);
#41339=ORIENTED_EDGE('',*,*,#29588,.F.);
#41340=ORIENTED_EDGE('',*,*,#29589,.T.);
#41341=ORIENTED_EDGE('',*,*,#29590,.T.);
#41342=ORIENTED_EDGE('',*,*,#29591,.T.);
#41343=ORIENTED_EDGE('',*,*,#29592,.F.);
#41344=ORIENTED_EDGE('',*,*,#29593,.T.);
#41345=ORIENTED_EDGE('',*,*,#29594,.T.);
#41346=ORIENTED_EDGE('',*,*,#29595,.T.);
#41347=ORIENTED_EDGE('',*,*,#29596,.F.);
#41348=ORIENTED_EDGE('',*,*,#29597,.T.);
#41349=ORIENTED_EDGE('',*,*,#29598,.T.);
#41350=ORIENTED_EDGE('',*,*,#29599,.T.);
#41351=ORIENTED_EDGE('',*,*,#29600,.F.);
#41352=ORIENTED_EDGE('',*,*,#29601,.T.);
#41353=ORIENTED_EDGE('',*,*,#29602,.T.);
#41354=ORIENTED_EDGE('',*,*,#29603,.T.);
#41355=ORIENTED_EDGE('',*,*,#29604,.F.);
#41356=ORIENTED_EDGE('',*,*,#29605,.T.);
#41357=ORIENTED_EDGE('',*,*,#29606,.T.);
#41358=ORIENTED_EDGE('',*,*,#29607,.T.);
#41359=ORIENTED_EDGE('',*,*,#29608,.F.);
#41360=ORIENTED_EDGE('',*,*,#29609,.T.);
#41361=ORIENTED_EDGE('',*,*,#29610,.T.);
#41362=ORIENTED_EDGE('',*,*,#29611,.T.);
#41363=ORIENTED_EDGE('',*,*,#29612,.F.);
#41364=ORIENTED_EDGE('',*,*,#29613,.T.);
#41365=ORIENTED_EDGE('',*,*,#29614,.T.);
#41366=ORIENTED_EDGE('',*,*,#29615,.T.);
#41367=ORIENTED_EDGE('',*,*,#29616,.F.);
#41368=ORIENTED_EDGE('',*,*,#29617,.T.);
#41369=ORIENTED_EDGE('',*,*,#29618,.T.);
#41370=ORIENTED_EDGE('',*,*,#29619,.T.);
#41371=ORIENTED_EDGE('',*,*,#29620,.F.);
#41372=ORIENTED_EDGE('',*,*,#29621,.T.);
#41373=ORIENTED_EDGE('',*,*,#29622,.T.);
#41374=ORIENTED_EDGE('',*,*,#29623,.T.);
#41375=ORIENTED_EDGE('',*,*,#29624,.F.);
#41376=ORIENTED_EDGE('',*,*,#29625,.T.);
#41377=ORIENTED_EDGE('',*,*,#29626,.T.);
#41378=ORIENTED_EDGE('',*,*,#29627,.T.);
#41379=ORIENTED_EDGE('',*,*,#29477,.F.);
#41380=ORIENTED_EDGE('',*,*,#29481,.F.);
#41381=ORIENTED_EDGE('',*,*,#29628,.F.);
#41382=ORIENTED_EDGE('',*,*,#29629,.F.);
#41383=ORIENTED_EDGE('',*,*,#29528,.F.);
#41384=ORIENTED_EDGE('',*,*,#29582,.F.);
#41385=ORIENTED_EDGE('',*,*,#29630,.F.);
#41386=ORIENTED_EDGE('',*,*,#29631,.F.);
#41387=ORIENTED_EDGE('',*,*,#29632,.F.);
#41388=ORIENTED_EDGE('',*,*,#29633,.F.);
#41389=ORIENTED_EDGE('',*,*,#29530,.F.);
#41390=ORIENTED_EDGE('',*,*,#29634,.T.);
#41391=ORIENTED_EDGE('',*,*,#29635,.F.);
#41392=ORIENTED_EDGE('',*,*,#29529,.F.);
#41393=ORIENTED_EDGE('',*,*,#29629,.T.);
#41394=ORIENTED_EDGE('',*,*,#29636,.F.);
#41395=ORIENTED_EDGE('',*,*,#29634,.F.);
#41396=ORIENTED_EDGE('',*,*,#29631,.T.);
#41397=ORIENTED_EDGE('',*,*,#29637,.F.);
#41398=ORIENTED_EDGE('',*,*,#29638,.T.);
#41399=ORIENTED_EDGE('',*,*,#29639,.T.);
#41400=ORIENTED_EDGE('',*,*,#29640,.T.);
#41401=ORIENTED_EDGE('',*,*,#29641,.T.);
#41402=ORIENTED_EDGE('',*,*,#29642,.T.);
#41403=ORIENTED_EDGE('',*,*,#29643,.T.);
#41404=ORIENTED_EDGE('',*,*,#29644,.T.);
#41405=ORIENTED_EDGE('',*,*,#29645,.T.);
#41406=ORIENTED_EDGE('',*,*,#29646,.T.);
#41407=ORIENTED_EDGE('',*,*,#29647,.T.);
#41408=ORIENTED_EDGE('',*,*,#29648,.T.);
#41409=ORIENTED_EDGE('',*,*,#29649,.T.);
#41410=ORIENTED_EDGE('',*,*,#29650,.T.);
#41411=ORIENTED_EDGE('',*,*,#29651,.T.);
#41412=ORIENTED_EDGE('',*,*,#29652,.T.);
#41413=ORIENTED_EDGE('',*,*,#29653,.T.);
#41414=ORIENTED_EDGE('',*,*,#29654,.T.);
#41415=ORIENTED_EDGE('',*,*,#29655,.T.);
#41416=ORIENTED_EDGE('',*,*,#29656,.T.);
#41417=ORIENTED_EDGE('',*,*,#29657,.T.);
#41418=ORIENTED_EDGE('',*,*,#29658,.T.);
#41419=ORIENTED_EDGE('',*,*,#29659,.T.);
#41420=ORIENTED_EDGE('',*,*,#29660,.T.);
#41421=ORIENTED_EDGE('',*,*,#29661,.T.);
#41422=ORIENTED_EDGE('',*,*,#29662,.T.);
#41423=ORIENTED_EDGE('',*,*,#29663,.T.);
#41424=ORIENTED_EDGE('',*,*,#29664,.T.);
#41425=ORIENTED_EDGE('',*,*,#29665,.T.);
#41426=ORIENTED_EDGE('',*,*,#29666,.T.);
#41427=ORIENTED_EDGE('',*,*,#29667,.T.);
#41428=ORIENTED_EDGE('',*,*,#29668,.T.);
#41429=ORIENTED_EDGE('',*,*,#29669,.T.);
#41430=ORIENTED_EDGE('',*,*,#29670,.T.);
#41431=ORIENTED_EDGE('',*,*,#29671,.T.);
#41432=ORIENTED_EDGE('',*,*,#29672,.T.);
#41433=ORIENTED_EDGE('',*,*,#29673,.T.);
#41434=ORIENTED_EDGE('',*,*,#29674,.T.);
#41435=ORIENTED_EDGE('',*,*,#29675,.T.);
#41436=ORIENTED_EDGE('',*,*,#29676,.T.);
#41437=ORIENTED_EDGE('',*,*,#29677,.T.);
#41438=ORIENTED_EDGE('',*,*,#29678,.T.);
#41439=ORIENTED_EDGE('',*,*,#29679,.T.);
#41440=ORIENTED_EDGE('',*,*,#29680,.T.);
#41441=ORIENTED_EDGE('',*,*,#29681,.T.);
#41442=ORIENTED_EDGE('',*,*,#29682,.T.);
#41443=ORIENTED_EDGE('',*,*,#29683,.T.);
#41444=ORIENTED_EDGE('',*,*,#29463,.T.);
#41445=ORIENTED_EDGE('',*,*,#29479,.T.);
#41446=ORIENTED_EDGE('',*,*,#29684,.T.);
#41447=ORIENTED_EDGE('',*,*,#29685,.T.);
#41448=ORIENTED_EDGE('',*,*,#29686,.T.);
#41449=ORIENTED_EDGE('',*,*,#29687,.T.);
#41450=ORIENTED_EDGE('',*,*,#29688,.T.);
#41451=ORIENTED_EDGE('',*,*,#29689,.T.);
#41452=ORIENTED_EDGE('',*,*,#29690,.T.);
#41453=ORIENTED_EDGE('',*,*,#29691,.T.);
#41454=ORIENTED_EDGE('',*,*,#29692,.T.);
#41455=ORIENTED_EDGE('',*,*,#29693,.T.);
#41456=ORIENTED_EDGE('',*,*,#29694,.T.);
#41457=ORIENTED_EDGE('',*,*,#29695,.T.);
#41458=ORIENTED_EDGE('',*,*,#29696,.T.);
#41459=ORIENTED_EDGE('',*,*,#29697,.T.);
#41460=ORIENTED_EDGE('',*,*,#29698,.T.);
#41461=ORIENTED_EDGE('',*,*,#29699,.T.);
#41462=ORIENTED_EDGE('',*,*,#29700,.T.);
#41463=ORIENTED_EDGE('',*,*,#29701,.T.);
#41464=ORIENTED_EDGE('',*,*,#29702,.T.);
#41465=ORIENTED_EDGE('',*,*,#29703,.T.);
#41466=ORIENTED_EDGE('',*,*,#29704,.T.);
#41467=ORIENTED_EDGE('',*,*,#29705,.T.);
#41468=ORIENTED_EDGE('',*,*,#29706,.T.);
#41469=ORIENTED_EDGE('',*,*,#29707,.T.);
#41470=ORIENTED_EDGE('',*,*,#29708,.T.);
#41471=ORIENTED_EDGE('',*,*,#29709,.T.);
#41472=ORIENTED_EDGE('',*,*,#29710,.T.);
#41473=ORIENTED_EDGE('',*,*,#29711,.T.);
#41474=ORIENTED_EDGE('',*,*,#29712,.T.);
#41475=ORIENTED_EDGE('',*,*,#29713,.T.);
#41476=ORIENTED_EDGE('',*,*,#29714,.T.);
#41477=ORIENTED_EDGE('',*,*,#29715,.T.);
#41478=ORIENTED_EDGE('',*,*,#29716,.T.);
#41479=ORIENTED_EDGE('',*,*,#29717,.T.);
#41480=ORIENTED_EDGE('',*,*,#29718,.T.);
#41481=ORIENTED_EDGE('',*,*,#29719,.T.);
#41482=ORIENTED_EDGE('',*,*,#29720,.T.);
#41483=ORIENTED_EDGE('',*,*,#29721,.T.);
#41484=ORIENTED_EDGE('',*,*,#29722,.T.);
#41485=ORIENTED_EDGE('',*,*,#29723,.T.);
#41486=ORIENTED_EDGE('',*,*,#29724,.T.);
#41487=ORIENTED_EDGE('',*,*,#29725,.T.);
#41488=ORIENTED_EDGE('',*,*,#29726,.T.);
#41489=ORIENTED_EDGE('',*,*,#29727,.T.);
#41490=ORIENTED_EDGE('',*,*,#29728,.T.);
#41491=ORIENTED_EDGE('',*,*,#29729,.F.);
#41492=ORIENTED_EDGE('',*,*,#29630,.T.);
#41493=ORIENTED_EDGE('',*,*,#29581,.T.);
#41494=ORIENTED_EDGE('',*,*,#29730,.T.);
#41495=ORIENTED_EDGE('',*,*,#29482,.F.);
#41496=ORIENTED_EDGE('',*,*,#29633,.T.);
#41497=ORIENTED_EDGE('',*,*,#29731,.F.);
#41498=ORIENTED_EDGE('',*,*,#29732,.T.);
#41499=ORIENTED_EDGE('',*,*,#29733,.T.);
#41500=ORIENTED_EDGE('',*,*,#29734,.T.);
#41501=ORIENTED_EDGE('',*,*,#29735,.F.);
#41502=ORIENTED_EDGE('',*,*,#29736,.T.);
#41503=ORIENTED_EDGE('',*,*,#29737,.T.);
#41504=ORIENTED_EDGE('',*,*,#29738,.T.);
#41505=ORIENTED_EDGE('',*,*,#29739,.F.);
#41506=ORIENTED_EDGE('',*,*,#29740,.T.);
#41507=ORIENTED_EDGE('',*,*,#29741,.T.);
#41508=ORIENTED_EDGE('',*,*,#29742,.T.);
#41509=ORIENTED_EDGE('',*,*,#29743,.F.);
#41510=ORIENTED_EDGE('',*,*,#29744,.T.);
#41511=ORIENTED_EDGE('',*,*,#29745,.T.);
#41512=ORIENTED_EDGE('',*,*,#29746,.T.);
#41513=ORIENTED_EDGE('',*,*,#29747,.F.);
#41514=ORIENTED_EDGE('',*,*,#29748,.T.);
#41515=ORIENTED_EDGE('',*,*,#29749,.T.);
#41516=ORIENTED_EDGE('',*,*,#29750,.T.);
#41517=ORIENTED_EDGE('',*,*,#29751,.F.);
#41518=ORIENTED_EDGE('',*,*,#29752,.T.);
#41519=ORIENTED_EDGE('',*,*,#29753,.T.);
#41520=ORIENTED_EDGE('',*,*,#29754,.T.);
#41521=ORIENTED_EDGE('',*,*,#29755,.F.);
#41522=ORIENTED_EDGE('',*,*,#29756,.T.);
#41523=ORIENTED_EDGE('',*,*,#29757,.T.);
#41524=ORIENTED_EDGE('',*,*,#29758,.T.);
#41525=ORIENTED_EDGE('',*,*,#29759,.F.);
#41526=ORIENTED_EDGE('',*,*,#29760,.T.);
#41527=ORIENTED_EDGE('',*,*,#29761,.T.);
#41528=ORIENTED_EDGE('',*,*,#29762,.T.);
#41529=ORIENTED_EDGE('',*,*,#29763,.F.);
#41530=ORIENTED_EDGE('',*,*,#29764,.T.);
#41531=ORIENTED_EDGE('',*,*,#29765,.T.);
#41532=ORIENTED_EDGE('',*,*,#29766,.T.);
#41533=ORIENTED_EDGE('',*,*,#29767,.F.);
#41534=ORIENTED_EDGE('',*,*,#29768,.T.);
#41535=ORIENTED_EDGE('',*,*,#29769,.T.);
#41536=ORIENTED_EDGE('',*,*,#29770,.T.);
#41537=ORIENTED_EDGE('',*,*,#29771,.F.);
#41538=ORIENTED_EDGE('',*,*,#29772,.T.);
#41539=ORIENTED_EDGE('',*,*,#29773,.T.);
#41540=ORIENTED_EDGE('',*,*,#29774,.T.);
#41541=ORIENTED_EDGE('',*,*,#29775,.F.);
#41542=ORIENTED_EDGE('',*,*,#29776,.T.);
#41543=ORIENTED_EDGE('',*,*,#29531,.T.);
#41544=ORIENTED_EDGE('',*,*,#29638,.F.);
#41545=ORIENTED_EDGE('',*,*,#29777,.F.);
#41546=ORIENTED_EDGE('',*,*,#29778,.F.);
#41547=ORIENTED_EDGE('',*,*,#29532,.F.);
#41548=ORIENTED_EDGE('',*,*,#29776,.F.);
#41549=ORIENTED_EDGE('',*,*,#29779,.F.);
#41550=ORIENTED_EDGE('',*,*,#29728,.F.);
#41551=ORIENTED_EDGE('',*,*,#29780,.F.);
#41552=ORIENTED_EDGE('',*,*,#29583,.F.);
#41553=ORIENTED_EDGE('',*,*,#29534,.F.);
#41554=ORIENTED_EDGE('',*,*,#29781,.T.);
#41555=ORIENTED_EDGE('',*,*,#29782,.F.);
#41556=ORIENTED_EDGE('',*,*,#29533,.F.);
#41557=ORIENTED_EDGE('',*,*,#29778,.T.);
#41558=ORIENTED_EDGE('',*,*,#29783,.F.);
#41559=ORIENTED_EDGE('',*,*,#29781,.F.);
#41560=ORIENTED_EDGE('',*,*,#29779,.T.);
#41561=ORIENTED_EDGE('',*,*,#29775,.T.);
#41562=ORIENTED_EDGE('',*,*,#29784,.T.);
#41563=ORIENTED_EDGE('',*,*,#29639,.F.);
#41564=ORIENTED_EDGE('',*,*,#29785,.F.);
#41565=ORIENTED_EDGE('',*,*,#29786,.F.);
#41566=ORIENTED_EDGE('',*,*,#29787,.F.);
#41567=ORIENTED_EDGE('',*,*,#29788,.F.);
#41568=ORIENTED_EDGE('',*,*,#29789,.F.);
#41569=ORIENTED_EDGE('',*,*,#29790,.F.);
#41570=ORIENTED_EDGE('',*,*,#29791,.F.);
#41571=ORIENTED_EDGE('',*,*,#29792,.F.);
#41572=ORIENTED_EDGE('',*,*,#29793,.F.);
#41573=ORIENTED_EDGE('',*,*,#29794,.F.);
#41574=ORIENTED_EDGE('',*,*,#29795,.F.);
#41575=ORIENTED_EDGE('',*,*,#29796,.F.);
#41576=ORIENTED_EDGE('',*,*,#29797,.F.);
#41577=ORIENTED_EDGE('',*,*,#29798,.F.);
#41578=ORIENTED_EDGE('',*,*,#29799,.F.);
#41579=ORIENTED_EDGE('',*,*,#29800,.F.);
#41580=ORIENTED_EDGE('',*,*,#29801,.F.);
#41581=ORIENTED_EDGE('',*,*,#29802,.F.);
#41582=ORIENTED_EDGE('',*,*,#29803,.F.);
#41583=ORIENTED_EDGE('',*,*,#29804,.F.);
#41584=ORIENTED_EDGE('',*,*,#29805,.F.);
#41585=ORIENTED_EDGE('',*,*,#29806,.F.);
#41586=ORIENTED_EDGE('',*,*,#29807,.F.);
#41587=ORIENTED_EDGE('',*,*,#29808,.F.);
#41588=ORIENTED_EDGE('',*,*,#29809,.F.);
#41589=ORIENTED_EDGE('',*,*,#29810,.F.);
#41590=ORIENTED_EDGE('',*,*,#29811,.F.);
#41591=ORIENTED_EDGE('',*,*,#29812,.F.);
#41592=ORIENTED_EDGE('',*,*,#29813,.F.);
#41593=ORIENTED_EDGE('',*,*,#29814,.F.);
#41594=ORIENTED_EDGE('',*,*,#29815,.F.);
#41595=ORIENTED_EDGE('',*,*,#29816,.F.);
#41596=ORIENTED_EDGE('',*,*,#29817,.F.);
#41597=ORIENTED_EDGE('',*,*,#29818,.F.);
#41598=ORIENTED_EDGE('',*,*,#29819,.F.);
#41599=ORIENTED_EDGE('',*,*,#29820,.F.);
#41600=ORIENTED_EDGE('',*,*,#29821,.F.);
#41601=ORIENTED_EDGE('',*,*,#29822,.F.);
#41602=ORIENTED_EDGE('',*,*,#29823,.F.);
#41603=ORIENTED_EDGE('',*,*,#29824,.F.);
#41604=ORIENTED_EDGE('',*,*,#29825,.F.);
#41605=ORIENTED_EDGE('',*,*,#29826,.F.);
#41606=ORIENTED_EDGE('',*,*,#29827,.F.);
#41607=ORIENTED_EDGE('',*,*,#29828,.F.);
#41608=ORIENTED_EDGE('',*,*,#29829,.F.);
#41609=ORIENTED_EDGE('',*,*,#29830,.F.);
#41610=ORIENTED_EDGE('',*,*,#29831,.F.);
#41611=ORIENTED_EDGE('',*,*,#29832,.F.);
#41612=ORIENTED_EDGE('',*,*,#29833,.F.);
#41613=ORIENTED_EDGE('',*,*,#29834,.F.);
#41614=ORIENTED_EDGE('',*,*,#29835,.F.);
#41615=ORIENTED_EDGE('',*,*,#29836,.F.);
#41616=ORIENTED_EDGE('',*,*,#29837,.F.);
#41617=ORIENTED_EDGE('',*,*,#29838,.F.);
#41618=ORIENTED_EDGE('',*,*,#29839,.F.);
#41619=ORIENTED_EDGE('',*,*,#29840,.F.);
#41620=ORIENTED_EDGE('',*,*,#29841,.F.);
#41621=ORIENTED_EDGE('',*,*,#29842,.F.);
#41622=ORIENTED_EDGE('',*,*,#29843,.F.);
#41623=ORIENTED_EDGE('',*,*,#29844,.F.);
#41624=ORIENTED_EDGE('',*,*,#29845,.F.);
#41625=ORIENTED_EDGE('',*,*,#29846,.F.);
#41626=ORIENTED_EDGE('',*,*,#29847,.F.);
#41627=ORIENTED_EDGE('',*,*,#29848,.F.);
#41628=ORIENTED_EDGE('',*,*,#29849,.F.);
#41629=ORIENTED_EDGE('',*,*,#29850,.F.);
#41630=ORIENTED_EDGE('',*,*,#29851,.F.);
#41631=ORIENTED_EDGE('',*,*,#29852,.F.);
#41632=ORIENTED_EDGE('',*,*,#29853,.F.);
#41633=ORIENTED_EDGE('',*,*,#29854,.F.);
#41634=ORIENTED_EDGE('',*,*,#29855,.F.);
#41635=ORIENTED_EDGE('',*,*,#29856,.F.);
#41636=ORIENTED_EDGE('',*,*,#29857,.F.);
#41637=ORIENTED_EDGE('',*,*,#29858,.F.);
#41638=ORIENTED_EDGE('',*,*,#29859,.F.);
#41639=ORIENTED_EDGE('',*,*,#29860,.F.);
#41640=ORIENTED_EDGE('',*,*,#29861,.F.);
#41641=ORIENTED_EDGE('',*,*,#29862,.F.);
#41642=ORIENTED_EDGE('',*,*,#29863,.F.);
#41643=ORIENTED_EDGE('',*,*,#29864,.F.);
#41644=ORIENTED_EDGE('',*,*,#29865,.F.);
#41645=ORIENTED_EDGE('',*,*,#29866,.F.);
#41646=ORIENTED_EDGE('',*,*,#29867,.F.);
#41647=ORIENTED_EDGE('',*,*,#29868,.F.);
#41648=ORIENTED_EDGE('',*,*,#29869,.F.);
#41649=ORIENTED_EDGE('',*,*,#29870,.F.);
#41650=ORIENTED_EDGE('',*,*,#29871,.F.);
#41651=ORIENTED_EDGE('',*,*,#29872,.F.);
#41652=ORIENTED_EDGE('',*,*,#29873,.F.);
#41653=ORIENTED_EDGE('',*,*,#29874,.F.);
#41654=ORIENTED_EDGE('',*,*,#29875,.F.);
#41655=ORIENTED_EDGE('',*,*,#29876,.F.);
#41656=ORIENTED_EDGE('',*,*,#29877,.F.);
#41657=ORIENTED_EDGE('',*,*,#29878,.F.);
#41658=ORIENTED_EDGE('',*,*,#29879,.F.);
#41659=ORIENTED_EDGE('',*,*,#29880,.F.);
#41660=ORIENTED_EDGE('',*,*,#29881,.F.);
#41661=ORIENTED_EDGE('',*,*,#29882,.F.);
#41662=ORIENTED_EDGE('',*,*,#29883,.F.);
#41663=ORIENTED_EDGE('',*,*,#29884,.F.);
#41664=ORIENTED_EDGE('',*,*,#29885,.F.);
#41665=ORIENTED_EDGE('',*,*,#29886,.F.);
#41666=ORIENTED_EDGE('',*,*,#29887,.F.);
#41667=ORIENTED_EDGE('',*,*,#29888,.F.);
#41668=ORIENTED_EDGE('',*,*,#29889,.F.);
#41669=ORIENTED_EDGE('',*,*,#29890,.F.);
#41670=ORIENTED_EDGE('',*,*,#29891,.F.);
#41671=ORIENTED_EDGE('',*,*,#29892,.F.);
#41672=ORIENTED_EDGE('',*,*,#29893,.F.);
#41673=ORIENTED_EDGE('',*,*,#29894,.F.);
#41674=ORIENTED_EDGE('',*,*,#29895,.F.);
#41675=ORIENTED_EDGE('',*,*,#29896,.F.);
#41676=ORIENTED_EDGE('',*,*,#29897,.F.);
#41677=ORIENTED_EDGE('',*,*,#29898,.F.);
#41678=ORIENTED_EDGE('',*,*,#29899,.F.);
#41679=ORIENTED_EDGE('',*,*,#29900,.F.);
#41680=ORIENTED_EDGE('',*,*,#29901,.F.);
#41681=ORIENTED_EDGE('',*,*,#29902,.F.);
#41682=ORIENTED_EDGE('',*,*,#29903,.F.);
#41683=ORIENTED_EDGE('',*,*,#29904,.F.);
#41684=ORIENTED_EDGE('',*,*,#29905,.F.);
#41685=ORIENTED_EDGE('',*,*,#29906,.F.);
#41686=ORIENTED_EDGE('',*,*,#29907,.F.);
#41687=ORIENTED_EDGE('',*,*,#29908,.F.);
#41688=ORIENTED_EDGE('',*,*,#29909,.F.);
#41689=ORIENTED_EDGE('',*,*,#29910,.F.);
#41690=ORIENTED_EDGE('',*,*,#29911,.F.);
#41691=ORIENTED_EDGE('',*,*,#29912,.F.);
#41692=ORIENTED_EDGE('',*,*,#29913,.F.);
#41693=ORIENTED_EDGE('',*,*,#29914,.F.);
#41694=ORIENTED_EDGE('',*,*,#29915,.F.);
#41695=ORIENTED_EDGE('',*,*,#29916,.F.);
#41696=ORIENTED_EDGE('',*,*,#29915,.T.);
#41697=ORIENTED_EDGE('',*,*,#29917,.F.);
#41698=ORIENTED_EDGE('',*,*,#29918,.T.);
#41699=ORIENTED_EDGE('',*,*,#29919,.T.);
#41700=ORIENTED_EDGE('',*,*,#29920,.T.);
#41701=ORIENTED_EDGE('',*,*,#29585,.F.);
#41702=ORIENTED_EDGE('',*,*,#29921,.F.);
#41703=ORIENTED_EDGE('',*,*,#29726,.F.);
#41704=ORIENTED_EDGE('',*,*,#29922,.T.);
#41705=ORIENTED_EDGE('',*,*,#29923,.F.);
#41706=ORIENTED_EDGE('',*,*,#29914,.T.);
#41707=ORIENTED_EDGE('',*,*,#29924,.F.);
#41708=ORIENTED_EDGE('',*,*,#29925,.T.);
#41709=ORIENTED_EDGE('',*,*,#29917,.T.);
#41710=ORIENTED_EDGE('',*,*,#29911,.T.);
#41711=ORIENTED_EDGE('',*,*,#29926,.F.);
#41712=ORIENTED_EDGE('',*,*,#29927,.T.);
#41713=ORIENTED_EDGE('',*,*,#29928,.T.);
#41714=ORIENTED_EDGE('',*,*,#29929,.T.);
#41715=ORIENTED_EDGE('',*,*,#29589,.F.);
#41716=ORIENTED_EDGE('',*,*,#29930,.F.);
#41717=ORIENTED_EDGE('',*,*,#29722,.F.);
#41718=ORIENTED_EDGE('',*,*,#29931,.T.);
#41719=ORIENTED_EDGE('',*,*,#29932,.F.);
#41720=ORIENTED_EDGE('',*,*,#29910,.T.);
#41721=ORIENTED_EDGE('',*,*,#29933,.F.);
#41722=ORIENTED_EDGE('',*,*,#29934,.T.);
#41723=ORIENTED_EDGE('',*,*,#29926,.T.);
#41724=ORIENTED_EDGE('',*,*,#29907,.T.);
#41725=ORIENTED_EDGE('',*,*,#29935,.F.);
#41726=ORIENTED_EDGE('',*,*,#29936,.T.);
#41727=ORIENTED_EDGE('',*,*,#29937,.T.);
#41728=ORIENTED_EDGE('',*,*,#29938,.T.);
#41729=ORIENTED_EDGE('',*,*,#29593,.F.);
#41730=ORIENTED_EDGE('',*,*,#29939,.F.);
#41731=ORIENTED_EDGE('',*,*,#29718,.F.);
#41732=ORIENTED_EDGE('',*,*,#29940,.T.);
#41733=ORIENTED_EDGE('',*,*,#29941,.F.);
#41734=ORIENTED_EDGE('',*,*,#29906,.T.);
#41735=ORIENTED_EDGE('',*,*,#29942,.F.);
#41736=ORIENTED_EDGE('',*,*,#29943,.T.);
#41737=ORIENTED_EDGE('',*,*,#29935,.T.);
#41738=ORIENTED_EDGE('',*,*,#29903,.T.);
#41739=ORIENTED_EDGE('',*,*,#29944,.F.);
#41740=ORIENTED_EDGE('',*,*,#29945,.T.);
#41741=ORIENTED_EDGE('',*,*,#29946,.T.);
#41742=ORIENTED_EDGE('',*,*,#29947,.T.);
#41743=ORIENTED_EDGE('',*,*,#29597,.F.);
#41744=ORIENTED_EDGE('',*,*,#29948,.F.);
#41745=ORIENTED_EDGE('',*,*,#29714,.F.);
#41746=ORIENTED_EDGE('',*,*,#29949,.T.);
#41747=ORIENTED_EDGE('',*,*,#29950,.F.);
#41748=ORIENTED_EDGE('',*,*,#29902,.T.);
#41749=ORIENTED_EDGE('',*,*,#29951,.F.);
#41750=ORIENTED_EDGE('',*,*,#29952,.T.);
#41751=ORIENTED_EDGE('',*,*,#29944,.T.);
#41752=ORIENTED_EDGE('',*,*,#29899,.T.);
#41753=ORIENTED_EDGE('',*,*,#29953,.F.);
#41754=ORIENTED_EDGE('',*,*,#29954,.T.);
#41755=ORIENTED_EDGE('',*,*,#29955,.T.);
#41756=ORIENTED_EDGE('',*,*,#29956,.T.);
#41757=ORIENTED_EDGE('',*,*,#29601,.F.);
#41758=ORIENTED_EDGE('',*,*,#29957,.F.);
#41759=ORIENTED_EDGE('',*,*,#29710,.F.);
#41760=ORIENTED_EDGE('',*,*,#29958,.T.);
#41761=ORIENTED_EDGE('',*,*,#29959,.F.);
#41762=ORIENTED_EDGE('',*,*,#29898,.T.);
#41763=ORIENTED_EDGE('',*,*,#29960,.F.);
#41764=ORIENTED_EDGE('',*,*,#29961,.T.);
#41765=ORIENTED_EDGE('',*,*,#29953,.T.);
#41766=ORIENTED_EDGE('',*,*,#29895,.T.);
#41767=ORIENTED_EDGE('',*,*,#29962,.F.);
#41768=ORIENTED_EDGE('',*,*,#29963,.T.);
#41769=ORIENTED_EDGE('',*,*,#29964,.T.);
#41770=ORIENTED_EDGE('',*,*,#29965,.T.);
#41771=ORIENTED_EDGE('',*,*,#29605,.F.);
#41772=ORIENTED_EDGE('',*,*,#29966,.F.);
#41773=ORIENTED_EDGE('',*,*,#29706,.F.);
#41774=ORIENTED_EDGE('',*,*,#29967,.T.);
#41775=ORIENTED_EDGE('',*,*,#29968,.F.);
#41776=ORIENTED_EDGE('',*,*,#29894,.T.);
#41777=ORIENTED_EDGE('',*,*,#29969,.F.);
#41778=ORIENTED_EDGE('',*,*,#29970,.T.);
#41779=ORIENTED_EDGE('',*,*,#29962,.T.);
#41780=ORIENTED_EDGE('',*,*,#29891,.T.);
#41781=ORIENTED_EDGE('',*,*,#29971,.F.);
#41782=ORIENTED_EDGE('',*,*,#29972,.T.);
#41783=ORIENTED_EDGE('',*,*,#29973,.T.);
#41784=ORIENTED_EDGE('',*,*,#29974,.T.);
#41785=ORIENTED_EDGE('',*,*,#29609,.F.);
#41786=ORIENTED_EDGE('',*,*,#29975,.F.);
#41787=ORIENTED_EDGE('',*,*,#29702,.F.);
#41788=ORIENTED_EDGE('',*,*,#29976,.T.);
#41789=ORIENTED_EDGE('',*,*,#29977,.F.);
#41790=ORIENTED_EDGE('',*,*,#29890,.T.);
#41791=ORIENTED_EDGE('',*,*,#29978,.F.);
#41792=ORIENTED_EDGE('',*,*,#29979,.T.);
#41793=ORIENTED_EDGE('',*,*,#29971,.T.);
#41794=ORIENTED_EDGE('',*,*,#29887,.T.);
#41795=ORIENTED_EDGE('',*,*,#29980,.F.);
#41796=ORIENTED_EDGE('',*,*,#29981,.T.);
#41797=ORIENTED_EDGE('',*,*,#29982,.T.);
#41798=ORIENTED_EDGE('',*,*,#29983,.T.);
#41799=ORIENTED_EDGE('',*,*,#29613,.F.);
#41800=ORIENTED_EDGE('',*,*,#29984,.F.);
#41801=ORIENTED_EDGE('',*,*,#29698,.F.);
#41802=ORIENTED_EDGE('',*,*,#29985,.T.);
#41803=ORIENTED_EDGE('',*,*,#29986,.F.);
#41804=ORIENTED_EDGE('',*,*,#29886,.T.);
#41805=ORIENTED_EDGE('',*,*,#29987,.F.);
#41806=ORIENTED_EDGE('',*,*,#29988,.T.);
#41807=ORIENTED_EDGE('',*,*,#29980,.T.);
#41808=ORIENTED_EDGE('',*,*,#29883,.T.);
#41809=ORIENTED_EDGE('',*,*,#29989,.F.);
#41810=ORIENTED_EDGE('',*,*,#29990,.T.);
#41811=ORIENTED_EDGE('',*,*,#29991,.T.);
#41812=ORIENTED_EDGE('',*,*,#29992,.T.);
#41813=ORIENTED_EDGE('',*,*,#29617,.F.);
#41814=ORIENTED_EDGE('',*,*,#29993,.F.);
#41815=ORIENTED_EDGE('',*,*,#29694,.F.);
#41816=ORIENTED_EDGE('',*,*,#29994,.T.);
#41817=ORIENTED_EDGE('',*,*,#29995,.F.);
#41818=ORIENTED_EDGE('',*,*,#29882,.T.);
#41819=ORIENTED_EDGE('',*,*,#29996,.F.);
#41820=ORIENTED_EDGE('',*,*,#29997,.T.);
#41821=ORIENTED_EDGE('',*,*,#29989,.T.);
#41822=ORIENTED_EDGE('',*,*,#29879,.T.);
#41823=ORIENTED_EDGE('',*,*,#29998,.F.);
#41824=ORIENTED_EDGE('',*,*,#29999,.T.);
#41825=ORIENTED_EDGE('',*,*,#30000,.T.);
#41826=ORIENTED_EDGE('',*,*,#30001,.T.);
#41827=ORIENTED_EDGE('',*,*,#29621,.F.);
#41828=ORIENTED_EDGE('',*,*,#30002,.F.);
#41829=ORIENTED_EDGE('',*,*,#29690,.F.);
#41830=ORIENTED_EDGE('',*,*,#30003,.T.);
#41831=ORIENTED_EDGE('',*,*,#30004,.F.);
#41832=ORIENTED_EDGE('',*,*,#29878,.T.);
#41833=ORIENTED_EDGE('',*,*,#30005,.F.);
#41834=ORIENTED_EDGE('',*,*,#30006,.T.);
#41835=ORIENTED_EDGE('',*,*,#29998,.T.);
#41836=ORIENTED_EDGE('',*,*,#29875,.T.);
#41837=ORIENTED_EDGE('',*,*,#30007,.F.);
#41838=ORIENTED_EDGE('',*,*,#30008,.T.);
#41839=ORIENTED_EDGE('',*,*,#30009,.T.);
#41840=ORIENTED_EDGE('',*,*,#30010,.T.);
#41841=ORIENTED_EDGE('',*,*,#29625,.F.);
#41842=ORIENTED_EDGE('',*,*,#30011,.F.);
#41843=ORIENTED_EDGE('',*,*,#29686,.F.);
#41844=ORIENTED_EDGE('',*,*,#30012,.T.);
#41845=ORIENTED_EDGE('',*,*,#30013,.F.);
#41846=ORIENTED_EDGE('',*,*,#29874,.T.);
#41847=ORIENTED_EDGE('',*,*,#30014,.F.);
#41848=ORIENTED_EDGE('',*,*,#30015,.T.);
#41849=ORIENTED_EDGE('',*,*,#30007,.T.);
#41850=ORIENTED_EDGE('',*,*,#29871,.T.);
#41851=ORIENTED_EDGE('',*,*,#30016,.F.);
#41852=ORIENTED_EDGE('',*,*,#30017,.T.);
#41853=ORIENTED_EDGE('',*,*,#30018,.T.);
#41854=ORIENTED_EDGE('',*,*,#30019,.T.);
#41855=ORIENTED_EDGE('',*,*,#29538,.F.);
#41856=ORIENTED_EDGE('',*,*,#30020,.F.);
#41857=ORIENTED_EDGE('',*,*,#29525,.F.);
#41858=ORIENTED_EDGE('',*,*,#30021,.T.);
#41859=ORIENTED_EDGE('',*,*,#30022,.F.);
#41860=ORIENTED_EDGE('',*,*,#29870,.T.);
#41861=ORIENTED_EDGE('',*,*,#30023,.F.);
#41862=ORIENTED_EDGE('',*,*,#30024,.T.);
#41863=ORIENTED_EDGE('',*,*,#30016,.T.);
#41864=ORIENTED_EDGE('',*,*,#29867,.T.);
#41865=ORIENTED_EDGE('',*,*,#30025,.F.);
#41866=ORIENTED_EDGE('',*,*,#30026,.T.);
#41867=ORIENTED_EDGE('',*,*,#30027,.T.);
#41868=ORIENTED_EDGE('',*,*,#30028,.T.);
#41869=ORIENTED_EDGE('',*,*,#29542,.F.);
#41870=ORIENTED_EDGE('',*,*,#30029,.F.);
#41871=ORIENTED_EDGE('',*,*,#29521,.F.);
#41872=ORIENTED_EDGE('',*,*,#30030,.T.);
#41873=ORIENTED_EDGE('',*,*,#30031,.F.);
#41874=ORIENTED_EDGE('',*,*,#29866,.T.);
#41875=ORIENTED_EDGE('',*,*,#30032,.F.);
#41876=ORIENTED_EDGE('',*,*,#30033,.T.);
#41877=ORIENTED_EDGE('',*,*,#30025,.T.);
#41878=ORIENTED_EDGE('',*,*,#29863,.T.);
#41879=ORIENTED_EDGE('',*,*,#30034,.F.);
#41880=ORIENTED_EDGE('',*,*,#30035,.T.);
#41881=ORIENTED_EDGE('',*,*,#30036,.T.);
#41882=ORIENTED_EDGE('',*,*,#30037,.T.);
#41883=ORIENTED_EDGE('',*,*,#29546,.F.);
#41884=ORIENTED_EDGE('',*,*,#30038,.F.);
#41885=ORIENTED_EDGE('',*,*,#29517,.F.);
#41886=ORIENTED_EDGE('',*,*,#30039,.T.);
#41887=ORIENTED_EDGE('',*,*,#30040,.F.);
#41888=ORIENTED_EDGE('',*,*,#29862,.T.);
#41889=ORIENTED_EDGE('',*,*,#30041,.F.);
#41890=ORIENTED_EDGE('',*,*,#30042,.T.);
#41891=ORIENTED_EDGE('',*,*,#30034,.T.);
#41892=ORIENTED_EDGE('',*,*,#29859,.T.);
#41893=ORIENTED_EDGE('',*,*,#30043,.F.);
#41894=ORIENTED_EDGE('',*,*,#30044,.T.);
#41895=ORIENTED_EDGE('',*,*,#30045,.T.);
#41896=ORIENTED_EDGE('',*,*,#30046,.T.);
#41897=ORIENTED_EDGE('',*,*,#29550,.F.);
#41898=ORIENTED_EDGE('',*,*,#30047,.F.);
#41899=ORIENTED_EDGE('',*,*,#29513,.F.);
#41900=ORIENTED_EDGE('',*,*,#30048,.T.);
#41901=ORIENTED_EDGE('',*,*,#30049,.F.);
#41902=ORIENTED_EDGE('',*,*,#29858,.T.);
#41903=ORIENTED_EDGE('',*,*,#30050,.F.);
#41904=ORIENTED_EDGE('',*,*,#30051,.T.);
#41905=ORIENTED_EDGE('',*,*,#30043,.T.);
#41906=ORIENTED_EDGE('',*,*,#29855,.T.);
#41907=ORIENTED_EDGE('',*,*,#30052,.F.);
#41908=ORIENTED_EDGE('',*,*,#30053,.T.);
#41909=ORIENTED_EDGE('',*,*,#30054,.T.);
#41910=ORIENTED_EDGE('',*,*,#30055,.T.);
#41911=ORIENTED_EDGE('',*,*,#29554,.F.);
#41912=ORIENTED_EDGE('',*,*,#30056,.F.);
#41913=ORIENTED_EDGE('',*,*,#29509,.F.);
#41914=ORIENTED_EDGE('',*,*,#30057,.T.);
#41915=ORIENTED_EDGE('',*,*,#30058,.F.);
#41916=ORIENTED_EDGE('',*,*,#29854,.T.);
#41917=ORIENTED_EDGE('',*,*,#30059,.F.);
#41918=ORIENTED_EDGE('',*,*,#30060,.T.);
#41919=ORIENTED_EDGE('',*,*,#30052,.T.);
#41920=ORIENTED_EDGE('',*,*,#29851,.T.);
#41921=ORIENTED_EDGE('',*,*,#30061,.F.);
#41922=ORIENTED_EDGE('',*,*,#30062,.T.);
#41923=ORIENTED_EDGE('',*,*,#30063,.T.);
#41924=ORIENTED_EDGE('',*,*,#30064,.T.);
#41925=ORIENTED_EDGE('',*,*,#29558,.F.);
#41926=ORIENTED_EDGE('',*,*,#30065,.F.);
#41927=ORIENTED_EDGE('',*,*,#29505,.F.);
#41928=ORIENTED_EDGE('',*,*,#30066,.T.);
#41929=ORIENTED_EDGE('',*,*,#30067,.F.);
#41930=ORIENTED_EDGE('',*,*,#29850,.T.);
#41931=ORIENTED_EDGE('',*,*,#30068,.F.);
#41932=ORIENTED_EDGE('',*,*,#30069,.T.);
#41933=ORIENTED_EDGE('',*,*,#30061,.T.);
#41934=ORIENTED_EDGE('',*,*,#29847,.T.);
#41935=ORIENTED_EDGE('',*,*,#30070,.F.);
#41936=ORIENTED_EDGE('',*,*,#30071,.T.);
#41937=ORIENTED_EDGE('',*,*,#30072,.T.);
#41938=ORIENTED_EDGE('',*,*,#30073,.T.);
#41939=ORIENTED_EDGE('',*,*,#29562,.F.);
#41940=ORIENTED_EDGE('',*,*,#30074,.F.);
#41941=ORIENTED_EDGE('',*,*,#29501,.F.);
#41942=ORIENTED_EDGE('',*,*,#30075,.T.);
#41943=ORIENTED_EDGE('',*,*,#30076,.F.);
#41944=ORIENTED_EDGE('',*,*,#29846,.T.);
#41945=ORIENTED_EDGE('',*,*,#30077,.F.);
#41946=ORIENTED_EDGE('',*,*,#30078,.T.);
#41947=ORIENTED_EDGE('',*,*,#30070,.T.);
#41948=ORIENTED_EDGE('',*,*,#29843,.T.);
#41949=ORIENTED_EDGE('',*,*,#30079,.F.);
#41950=ORIENTED_EDGE('',*,*,#30080,.T.);
#41951=ORIENTED_EDGE('',*,*,#30081,.T.);
#41952=ORIENTED_EDGE('',*,*,#30082,.T.);
#41953=ORIENTED_EDGE('',*,*,#29566,.F.);
#41954=ORIENTED_EDGE('',*,*,#30083,.F.);
#41955=ORIENTED_EDGE('',*,*,#29497,.F.);
#41956=ORIENTED_EDGE('',*,*,#30084,.T.);
#41957=ORIENTED_EDGE('',*,*,#30085,.F.);
#41958=ORIENTED_EDGE('',*,*,#29842,.T.);
#41959=ORIENTED_EDGE('',*,*,#30086,.F.);
#41960=ORIENTED_EDGE('',*,*,#30087,.T.);
#41961=ORIENTED_EDGE('',*,*,#30079,.T.);
#41962=ORIENTED_EDGE('',*,*,#29839,.T.);
#41963=ORIENTED_EDGE('',*,*,#30088,.F.);
#41964=ORIENTED_EDGE('',*,*,#30089,.T.);
#41965=ORIENTED_EDGE('',*,*,#30090,.T.);
#41966=ORIENTED_EDGE('',*,*,#30091,.T.);
#41967=ORIENTED_EDGE('',*,*,#29570,.F.);
#41968=ORIENTED_EDGE('',*,*,#30092,.F.);
#41969=ORIENTED_EDGE('',*,*,#29493,.F.);
#41970=ORIENTED_EDGE('',*,*,#30093,.T.);
#41971=ORIENTED_EDGE('',*,*,#30094,.F.);
#41972=ORIENTED_EDGE('',*,*,#29838,.T.);
#41973=ORIENTED_EDGE('',*,*,#30095,.F.);
#41974=ORIENTED_EDGE('',*,*,#30096,.T.);
#41975=ORIENTED_EDGE('',*,*,#30088,.T.);
#41976=ORIENTED_EDGE('',*,*,#29835,.T.);
#41977=ORIENTED_EDGE('',*,*,#30097,.F.);
#41978=ORIENTED_EDGE('',*,*,#30098,.T.);
#41979=ORIENTED_EDGE('',*,*,#30099,.T.);
#41980=ORIENTED_EDGE('',*,*,#30100,.T.);
#41981=ORIENTED_EDGE('',*,*,#29574,.F.);
#41982=ORIENTED_EDGE('',*,*,#30101,.F.);
#41983=ORIENTED_EDGE('',*,*,#29489,.F.);
#41984=ORIENTED_EDGE('',*,*,#30102,.T.);
#41985=ORIENTED_EDGE('',*,*,#30103,.F.);
#41986=ORIENTED_EDGE('',*,*,#29834,.T.);
#41987=ORIENTED_EDGE('',*,*,#30104,.F.);
#41988=ORIENTED_EDGE('',*,*,#30105,.T.);
#41989=ORIENTED_EDGE('',*,*,#30097,.T.);
#41990=ORIENTED_EDGE('',*,*,#29831,.T.);
#41991=ORIENTED_EDGE('',*,*,#30106,.F.);
#41992=ORIENTED_EDGE('',*,*,#30107,.T.);
#41993=ORIENTED_EDGE('',*,*,#30108,.T.);
#41994=ORIENTED_EDGE('',*,*,#30109,.T.);
#41995=ORIENTED_EDGE('',*,*,#29578,.F.);
#41996=ORIENTED_EDGE('',*,*,#30110,.F.);
#41997=ORIENTED_EDGE('',*,*,#29485,.F.);
#41998=ORIENTED_EDGE('',*,*,#30111,.T.);
#41999=ORIENTED_EDGE('',*,*,#30112,.F.);
#42000=ORIENTED_EDGE('',*,*,#29830,.T.);
#42001=ORIENTED_EDGE('',*,*,#30113,.F.);
#42002=ORIENTED_EDGE('',*,*,#30114,.T.);
#42003=ORIENTED_EDGE('',*,*,#30106,.T.);
#42004=ORIENTED_EDGE('',*,*,#29827,.T.);
#42005=ORIENTED_EDGE('',*,*,#30115,.F.);
#42006=ORIENTED_EDGE('',*,*,#30116,.T.);
#42007=ORIENTED_EDGE('',*,*,#30117,.T.);
#42008=ORIENTED_EDGE('',*,*,#30118,.T.);
#42009=ORIENTED_EDGE('',*,*,#29732,.F.);
#42010=ORIENTED_EDGE('',*,*,#30119,.F.);
#42011=ORIENTED_EDGE('',*,*,#29682,.F.);
#42012=ORIENTED_EDGE('',*,*,#30120,.T.);
#42013=ORIENTED_EDGE('',*,*,#30121,.F.);
#42014=ORIENTED_EDGE('',*,*,#29826,.T.);
#42015=ORIENTED_EDGE('',*,*,#30122,.F.);
#42016=ORIENTED_EDGE('',*,*,#30123,.T.);
#42017=ORIENTED_EDGE('',*,*,#30115,.T.);
#42018=ORIENTED_EDGE('',*,*,#29823,.T.);
#42019=ORIENTED_EDGE('',*,*,#30124,.F.);
#42020=ORIENTED_EDGE('',*,*,#30125,.T.);
#42021=ORIENTED_EDGE('',*,*,#30126,.T.);
#42022=ORIENTED_EDGE('',*,*,#30127,.T.);
#42023=ORIENTED_EDGE('',*,*,#29736,.F.);
#42024=ORIENTED_EDGE('',*,*,#30128,.F.);
#42025=ORIENTED_EDGE('',*,*,#29678,.F.);
#42026=ORIENTED_EDGE('',*,*,#30129,.T.);
#42027=ORIENTED_EDGE('',*,*,#30130,.F.);
#42028=ORIENTED_EDGE('',*,*,#29822,.T.);
#42029=ORIENTED_EDGE('',*,*,#30131,.F.);
#42030=ORIENTED_EDGE('',*,*,#30132,.T.);
#42031=ORIENTED_EDGE('',*,*,#30124,.T.);
#42032=ORIENTED_EDGE('',*,*,#29819,.T.);
#42033=ORIENTED_EDGE('',*,*,#30133,.F.);
#42034=ORIENTED_EDGE('',*,*,#30134,.T.);
#42035=ORIENTED_EDGE('',*,*,#30135,.T.);
#42036=ORIENTED_EDGE('',*,*,#30136,.T.);
#42037=ORIENTED_EDGE('',*,*,#29740,.F.);
#42038=ORIENTED_EDGE('',*,*,#30137,.F.);
#42039=ORIENTED_EDGE('',*,*,#29674,.F.);
#42040=ORIENTED_EDGE('',*,*,#30138,.T.);
#42041=ORIENTED_EDGE('',*,*,#30139,.F.);
#42042=ORIENTED_EDGE('',*,*,#29818,.T.);
#42043=ORIENTED_EDGE('',*,*,#30140,.F.);
#42044=ORIENTED_EDGE('',*,*,#30141,.T.);
#42045=ORIENTED_EDGE('',*,*,#30133,.T.);
#42046=ORIENTED_EDGE('',*,*,#29815,.T.);
#42047=ORIENTED_EDGE('',*,*,#30142,.F.);
#42048=ORIENTED_EDGE('',*,*,#30143,.T.);
#42049=ORIENTED_EDGE('',*,*,#30144,.T.);
#42050=ORIENTED_EDGE('',*,*,#30145,.T.);
#42051=ORIENTED_EDGE('',*,*,#29744,.F.);
#42052=ORIENTED_EDGE('',*,*,#30146,.F.);
#42053=ORIENTED_EDGE('',*,*,#29670,.F.);
#42054=ORIENTED_EDGE('',*,*,#30147,.T.);
#42055=ORIENTED_EDGE('',*,*,#30148,.F.);
#42056=ORIENTED_EDGE('',*,*,#29814,.T.);
#42057=ORIENTED_EDGE('',*,*,#30149,.F.);
#42058=ORIENTED_EDGE('',*,*,#30150,.T.);
#42059=ORIENTED_EDGE('',*,*,#30142,.T.);
#42060=ORIENTED_EDGE('',*,*,#29811,.T.);
#42061=ORIENTED_EDGE('',*,*,#30151,.F.);
#42062=ORIENTED_EDGE('',*,*,#30152,.T.);
#42063=ORIENTED_EDGE('',*,*,#30153,.T.);
#42064=ORIENTED_EDGE('',*,*,#30154,.T.);
#42065=ORIENTED_EDGE('',*,*,#29748,.F.);
#42066=ORIENTED_EDGE('',*,*,#30155,.F.);
#42067=ORIENTED_EDGE('',*,*,#29666,.F.);
#42068=ORIENTED_EDGE('',*,*,#30156,.T.);
#42069=ORIENTED_EDGE('',*,*,#30157,.F.);
#42070=ORIENTED_EDGE('',*,*,#29810,.T.);
#42071=ORIENTED_EDGE('',*,*,#30158,.F.);
#42072=ORIENTED_EDGE('',*,*,#30159,.T.);
#42073=ORIENTED_EDGE('',*,*,#30151,.T.);
#42074=ORIENTED_EDGE('',*,*,#29807,.T.);
#42075=ORIENTED_EDGE('',*,*,#30160,.F.);
#42076=ORIENTED_EDGE('',*,*,#30161,.T.);
#42077=ORIENTED_EDGE('',*,*,#30162,.T.);
#42078=ORIENTED_EDGE('',*,*,#30163,.T.);
#42079=ORIENTED_EDGE('',*,*,#29752,.F.);
#42080=ORIENTED_EDGE('',*,*,#30164,.F.);
#42081=ORIENTED_EDGE('',*,*,#29662,.F.);
#42082=ORIENTED_EDGE('',*,*,#30165,.T.);
#42083=ORIENTED_EDGE('',*,*,#30166,.F.);
#42084=ORIENTED_EDGE('',*,*,#29806,.T.);
#42085=ORIENTED_EDGE('',*,*,#30167,.F.);
#42086=ORIENTED_EDGE('',*,*,#30168,.T.);
#42087=ORIENTED_EDGE('',*,*,#30160,.T.);
#42088=ORIENTED_EDGE('',*,*,#29803,.T.);
#42089=ORIENTED_EDGE('',*,*,#30169,.F.);
#42090=ORIENTED_EDGE('',*,*,#30170,.T.);
#42091=ORIENTED_EDGE('',*,*,#30171,.T.);
#42092=ORIENTED_EDGE('',*,*,#30172,.T.);
#42093=ORIENTED_EDGE('',*,*,#29756,.F.);
#42094=ORIENTED_EDGE('',*,*,#30173,.F.);
#42095=ORIENTED_EDGE('',*,*,#29658,.F.);
#42096=ORIENTED_EDGE('',*,*,#30174,.T.);
#42097=ORIENTED_EDGE('',*,*,#30175,.F.);
#42098=ORIENTED_EDGE('',*,*,#29802,.T.);
#42099=ORIENTED_EDGE('',*,*,#30176,.F.);
#42100=ORIENTED_EDGE('',*,*,#30177,.T.);
#42101=ORIENTED_EDGE('',*,*,#30169,.T.);
#42102=ORIENTED_EDGE('',*,*,#29799,.T.);
#42103=ORIENTED_EDGE('',*,*,#30178,.F.);
#42104=ORIENTED_EDGE('',*,*,#30179,.T.);
#42105=ORIENTED_EDGE('',*,*,#30180,.T.);
#42106=ORIENTED_EDGE('',*,*,#30181,.T.);
#42107=ORIENTED_EDGE('',*,*,#29760,.F.);
#42108=ORIENTED_EDGE('',*,*,#30182,.F.);
#42109=ORIENTED_EDGE('',*,*,#29654,.F.);
#42110=ORIENTED_EDGE('',*,*,#30183,.T.);
#42111=ORIENTED_EDGE('',*,*,#30184,.F.);
#42112=ORIENTED_EDGE('',*,*,#29798,.T.);
#42113=ORIENTED_EDGE('',*,*,#30185,.F.);
#42114=ORIENTED_EDGE('',*,*,#30186,.T.);
#42115=ORIENTED_EDGE('',*,*,#30178,.T.);
#42116=ORIENTED_EDGE('',*,*,#29795,.T.);
#42117=ORIENTED_EDGE('',*,*,#30187,.F.);
#42118=ORIENTED_EDGE('',*,*,#30188,.T.);
#42119=ORIENTED_EDGE('',*,*,#30189,.T.);
#42120=ORIENTED_EDGE('',*,*,#30190,.T.);
#42121=ORIENTED_EDGE('',*,*,#29764,.F.);
#42122=ORIENTED_EDGE('',*,*,#30191,.F.);
#42123=ORIENTED_EDGE('',*,*,#29650,.F.);
#42124=ORIENTED_EDGE('',*,*,#30192,.T.);
#42125=ORIENTED_EDGE('',*,*,#30193,.F.);
#42126=ORIENTED_EDGE('',*,*,#29794,.T.);
#42127=ORIENTED_EDGE('',*,*,#30194,.F.);
#42128=ORIENTED_EDGE('',*,*,#30195,.T.);
#42129=ORIENTED_EDGE('',*,*,#30187,.T.);
#42130=ORIENTED_EDGE('',*,*,#29791,.T.);
#42131=ORIENTED_EDGE('',*,*,#30196,.F.);
#42132=ORIENTED_EDGE('',*,*,#30197,.T.);
#42133=ORIENTED_EDGE('',*,*,#30198,.T.);
#42134=ORIENTED_EDGE('',*,*,#30199,.T.);
#42135=ORIENTED_EDGE('',*,*,#29768,.F.);
#42136=ORIENTED_EDGE('',*,*,#30200,.F.);
#42137=ORIENTED_EDGE('',*,*,#29646,.F.);
#42138=ORIENTED_EDGE('',*,*,#30201,.T.);
#42139=ORIENTED_EDGE('',*,*,#30202,.F.);
#42140=ORIENTED_EDGE('',*,*,#29790,.T.);
#42141=ORIENTED_EDGE('',*,*,#30203,.F.);
#42142=ORIENTED_EDGE('',*,*,#30204,.T.);
#42143=ORIENTED_EDGE('',*,*,#30196,.T.);
#42144=ORIENTED_EDGE('',*,*,#29787,.T.);
#42145=ORIENTED_EDGE('',*,*,#30205,.F.);
#42146=ORIENTED_EDGE('',*,*,#30206,.T.);
#42147=ORIENTED_EDGE('',*,*,#30207,.T.);
#42148=ORIENTED_EDGE('',*,*,#30208,.T.);
#42149=ORIENTED_EDGE('',*,*,#29772,.F.);
#42150=ORIENTED_EDGE('',*,*,#30209,.F.);
#42151=ORIENTED_EDGE('',*,*,#29642,.F.);
#42152=ORIENTED_EDGE('',*,*,#30210,.T.);
#42153=ORIENTED_EDGE('',*,*,#30211,.F.);
#42154=ORIENTED_EDGE('',*,*,#29786,.T.);
#42155=ORIENTED_EDGE('',*,*,#30212,.F.);
#42156=ORIENTED_EDGE('',*,*,#30213,.T.);
#42157=ORIENTED_EDGE('',*,*,#30205,.T.);
#42158=ORIENTED_EDGE('',*,*,#30206,.F.);
#42159=ORIENTED_EDGE('',*,*,#30213,.F.);
#42160=ORIENTED_EDGE('',*,*,#30214,.F.);
#42161=ORIENTED_EDGE('',*,*,#30215,.F.);
#42162=ORIENTED_EDGE('',*,*,#30197,.F.);
#42163=ORIENTED_EDGE('',*,*,#30204,.F.);
#42164=ORIENTED_EDGE('',*,*,#30216,.F.);
#42165=ORIENTED_EDGE('',*,*,#30217,.F.);
#42166=ORIENTED_EDGE('',*,*,#30188,.F.);
#42167=ORIENTED_EDGE('',*,*,#30195,.F.);
#42168=ORIENTED_EDGE('',*,*,#30218,.F.);
#42169=ORIENTED_EDGE('',*,*,#30219,.F.);
#42170=ORIENTED_EDGE('',*,*,#30179,.F.);
#42171=ORIENTED_EDGE('',*,*,#30186,.F.);
#42172=ORIENTED_EDGE('',*,*,#30220,.F.);
#42173=ORIENTED_EDGE('',*,*,#30221,.F.);
#42174=ORIENTED_EDGE('',*,*,#30170,.F.);
#42175=ORIENTED_EDGE('',*,*,#30177,.F.);
#42176=ORIENTED_EDGE('',*,*,#30222,.F.);
#42177=ORIENTED_EDGE('',*,*,#30223,.F.);
#42178=ORIENTED_EDGE('',*,*,#30161,.F.);
#42179=ORIENTED_EDGE('',*,*,#30168,.F.);
#42180=ORIENTED_EDGE('',*,*,#30224,.F.);
#42181=ORIENTED_EDGE('',*,*,#30225,.F.);
#42182=ORIENTED_EDGE('',*,*,#30152,.F.);
#42183=ORIENTED_EDGE('',*,*,#30159,.F.);
#42184=ORIENTED_EDGE('',*,*,#30226,.F.);
#42185=ORIENTED_EDGE('',*,*,#30227,.F.);
#42186=ORIENTED_EDGE('',*,*,#30143,.F.);
#42187=ORIENTED_EDGE('',*,*,#30150,.F.);
#42188=ORIENTED_EDGE('',*,*,#30228,.F.);
#42189=ORIENTED_EDGE('',*,*,#30229,.F.);
#42190=ORIENTED_EDGE('',*,*,#30134,.F.);
#42191=ORIENTED_EDGE('',*,*,#30141,.F.);
#42192=ORIENTED_EDGE('',*,*,#30230,.F.);
#42193=ORIENTED_EDGE('',*,*,#30231,.F.);
#42194=ORIENTED_EDGE('',*,*,#30125,.F.);
#42195=ORIENTED_EDGE('',*,*,#30132,.F.);
#42196=ORIENTED_EDGE('',*,*,#30232,.F.);
#42197=ORIENTED_EDGE('',*,*,#30233,.F.);
#42198=ORIENTED_EDGE('',*,*,#30116,.F.);
#42199=ORIENTED_EDGE('',*,*,#30123,.F.);
#42200=ORIENTED_EDGE('',*,*,#30234,.F.);
#42201=ORIENTED_EDGE('',*,*,#30235,.F.);
#42202=ORIENTED_EDGE('',*,*,#30107,.F.);
#42203=ORIENTED_EDGE('',*,*,#30114,.F.);
#42204=ORIENTED_EDGE('',*,*,#30236,.F.);
#42205=ORIENTED_EDGE('',*,*,#30237,.F.);
#42206=ORIENTED_EDGE('',*,*,#30098,.F.);
#42207=ORIENTED_EDGE('',*,*,#30105,.F.);
#42208=ORIENTED_EDGE('',*,*,#30238,.F.);
#42209=ORIENTED_EDGE('',*,*,#30239,.F.);
#42210=ORIENTED_EDGE('',*,*,#30089,.F.);
#42211=ORIENTED_EDGE('',*,*,#30096,.F.);
#42212=ORIENTED_EDGE('',*,*,#30240,.F.);
#42213=ORIENTED_EDGE('',*,*,#30241,.F.);
#42214=ORIENTED_EDGE('',*,*,#30080,.F.);
#42215=ORIENTED_EDGE('',*,*,#30087,.F.);
#42216=ORIENTED_EDGE('',*,*,#30242,.F.);
#42217=ORIENTED_EDGE('',*,*,#30243,.F.);
#42218=ORIENTED_EDGE('',*,*,#30071,.F.);
#42219=ORIENTED_EDGE('',*,*,#30078,.F.);
#42220=ORIENTED_EDGE('',*,*,#30244,.F.);
#42221=ORIENTED_EDGE('',*,*,#30245,.F.);
#42222=ORIENTED_EDGE('',*,*,#30062,.F.);
#42223=ORIENTED_EDGE('',*,*,#30069,.F.);
#42224=ORIENTED_EDGE('',*,*,#30246,.F.);
#42225=ORIENTED_EDGE('',*,*,#30247,.F.);
#42226=ORIENTED_EDGE('',*,*,#30053,.F.);
#42227=ORIENTED_EDGE('',*,*,#30060,.F.);
#42228=ORIENTED_EDGE('',*,*,#30248,.F.);
#42229=ORIENTED_EDGE('',*,*,#30249,.F.);
#42230=ORIENTED_EDGE('',*,*,#30044,.F.);
#42231=ORIENTED_EDGE('',*,*,#30051,.F.);
#42232=ORIENTED_EDGE('',*,*,#30250,.F.);
#42233=ORIENTED_EDGE('',*,*,#30251,.F.);
#42234=ORIENTED_EDGE('',*,*,#30035,.F.);
#42235=ORIENTED_EDGE('',*,*,#30042,.F.);
#42236=ORIENTED_EDGE('',*,*,#30252,.F.);
#42237=ORIENTED_EDGE('',*,*,#30253,.F.);
#42238=ORIENTED_EDGE('',*,*,#30026,.F.);
#42239=ORIENTED_EDGE('',*,*,#30033,.F.);
#42240=ORIENTED_EDGE('',*,*,#30254,.F.);
#42241=ORIENTED_EDGE('',*,*,#30255,.F.);
#42242=ORIENTED_EDGE('',*,*,#30017,.F.);
#42243=ORIENTED_EDGE('',*,*,#30024,.F.);
#42244=ORIENTED_EDGE('',*,*,#30256,.F.);
#42245=ORIENTED_EDGE('',*,*,#30257,.F.);
#42246=ORIENTED_EDGE('',*,*,#30008,.F.);
#42247=ORIENTED_EDGE('',*,*,#30015,.F.);
#42248=ORIENTED_EDGE('',*,*,#30258,.F.);
#42249=ORIENTED_EDGE('',*,*,#30259,.F.);
#42250=ORIENTED_EDGE('',*,*,#29999,.F.);
#42251=ORIENTED_EDGE('',*,*,#30006,.F.);
#42252=ORIENTED_EDGE('',*,*,#30260,.F.);
#42253=ORIENTED_EDGE('',*,*,#30261,.F.);
#42254=ORIENTED_EDGE('',*,*,#29990,.F.);
#42255=ORIENTED_EDGE('',*,*,#29997,.F.);
#42256=ORIENTED_EDGE('',*,*,#30262,.F.);
#42257=ORIENTED_EDGE('',*,*,#30263,.F.);
#42258=ORIENTED_EDGE('',*,*,#29981,.F.);
#42259=ORIENTED_EDGE('',*,*,#29988,.F.);
#42260=ORIENTED_EDGE('',*,*,#30264,.F.);
#42261=ORIENTED_EDGE('',*,*,#30265,.F.);
#42262=ORIENTED_EDGE('',*,*,#29972,.F.);
#42263=ORIENTED_EDGE('',*,*,#29979,.F.);
#42264=ORIENTED_EDGE('',*,*,#30266,.F.);
#42265=ORIENTED_EDGE('',*,*,#30267,.F.);
#42266=ORIENTED_EDGE('',*,*,#29963,.F.);
#42267=ORIENTED_EDGE('',*,*,#29970,.F.);
#42268=ORIENTED_EDGE('',*,*,#30268,.F.);
#42269=ORIENTED_EDGE('',*,*,#30269,.F.);
#42270=ORIENTED_EDGE('',*,*,#29954,.F.);
#42271=ORIENTED_EDGE('',*,*,#29961,.F.);
#42272=ORIENTED_EDGE('',*,*,#30270,.F.);
#42273=ORIENTED_EDGE('',*,*,#30271,.F.);
#42274=ORIENTED_EDGE('',*,*,#29945,.F.);
#42275=ORIENTED_EDGE('',*,*,#29952,.F.);
#42276=ORIENTED_EDGE('',*,*,#30272,.F.);
#42277=ORIENTED_EDGE('',*,*,#30273,.F.);
#42278=ORIENTED_EDGE('',*,*,#29936,.F.);
#42279=ORIENTED_EDGE('',*,*,#29943,.F.);
#42280=ORIENTED_EDGE('',*,*,#30274,.F.);
#42281=ORIENTED_EDGE('',*,*,#30275,.F.);
#42282=ORIENTED_EDGE('',*,*,#29927,.F.);
#42283=ORIENTED_EDGE('',*,*,#29934,.F.);
#42284=ORIENTED_EDGE('',*,*,#30276,.F.);
#42285=ORIENTED_EDGE('',*,*,#30277,.F.);
#42286=ORIENTED_EDGE('',*,*,#29918,.F.);
#42287=ORIENTED_EDGE('',*,*,#29925,.F.);
#42288=ORIENTED_EDGE('',*,*,#30278,.F.);
#42289=ORIENTED_EDGE('',*,*,#30279,.F.);
#42290=ORIENTED_EDGE('',*,*,#29913,.T.);
#42291=ORIENTED_EDGE('',*,*,#30280,.F.);
#42292=ORIENTED_EDGE('',*,*,#30281,.F.);
#42293=ORIENTED_EDGE('',*,*,#29724,.F.);
#42294=ORIENTED_EDGE('',*,*,#30282,.F.);
#42295=ORIENTED_EDGE('',*,*,#29587,.F.);
#42296=ORIENTED_EDGE('',*,*,#30283,.F.);
#42297=ORIENTED_EDGE('',*,*,#30284,.T.);
#42298=ORIENTED_EDGE('',*,*,#30278,.T.);
#42299=ORIENTED_EDGE('',*,*,#29924,.T.);
#42300=ORIENTED_EDGE('',*,*,#29909,.T.);
#42301=ORIENTED_EDGE('',*,*,#30285,.F.);
#42302=ORIENTED_EDGE('',*,*,#30286,.F.);
#42303=ORIENTED_EDGE('',*,*,#29720,.F.);
#42304=ORIENTED_EDGE('',*,*,#30287,.F.);
#42305=ORIENTED_EDGE('',*,*,#29591,.F.);
#42306=ORIENTED_EDGE('',*,*,#30288,.F.);
#42307=ORIENTED_EDGE('',*,*,#30289,.T.);
#42308=ORIENTED_EDGE('',*,*,#30276,.T.);
#42309=ORIENTED_EDGE('',*,*,#29933,.T.);
#42310=ORIENTED_EDGE('',*,*,#29905,.T.);
#42311=ORIENTED_EDGE('',*,*,#30290,.F.);
#42312=ORIENTED_EDGE('',*,*,#30291,.F.);
#42313=ORIENTED_EDGE('',*,*,#29716,.F.);
#42314=ORIENTED_EDGE('',*,*,#30292,.F.);
#42315=ORIENTED_EDGE('',*,*,#29595,.F.);
#42316=ORIENTED_EDGE('',*,*,#30293,.F.);
#42317=ORIENTED_EDGE('',*,*,#30294,.T.);
#42318=ORIENTED_EDGE('',*,*,#30274,.T.);
#42319=ORIENTED_EDGE('',*,*,#29942,.T.);
#42320=ORIENTED_EDGE('',*,*,#29901,.T.);
#42321=ORIENTED_EDGE('',*,*,#30295,.F.);
#42322=ORIENTED_EDGE('',*,*,#30296,.F.);
#42323=ORIENTED_EDGE('',*,*,#29712,.F.);
#42324=ORIENTED_EDGE('',*,*,#30297,.F.);
#42325=ORIENTED_EDGE('',*,*,#29599,.F.);
#42326=ORIENTED_EDGE('',*,*,#30298,.F.);
#42327=ORIENTED_EDGE('',*,*,#30299,.T.);
#42328=ORIENTED_EDGE('',*,*,#30272,.T.);
#42329=ORIENTED_EDGE('',*,*,#29951,.T.);
#42330=ORIENTED_EDGE('',*,*,#29897,.T.);
#42331=ORIENTED_EDGE('',*,*,#30300,.F.);
#42332=ORIENTED_EDGE('',*,*,#30301,.F.);
#42333=ORIENTED_EDGE('',*,*,#29708,.F.);
#42334=ORIENTED_EDGE('',*,*,#30302,.F.);
#42335=ORIENTED_EDGE('',*,*,#29603,.F.);
#42336=ORIENTED_EDGE('',*,*,#30303,.F.);
#42337=ORIENTED_EDGE('',*,*,#30304,.T.);
#42338=ORIENTED_EDGE('',*,*,#30270,.T.);
#42339=ORIENTED_EDGE('',*,*,#29960,.T.);
#42340=ORIENTED_EDGE('',*,*,#29893,.T.);
#42341=ORIENTED_EDGE('',*,*,#30305,.F.);
#42342=ORIENTED_EDGE('',*,*,#30306,.F.);
#42343=ORIENTED_EDGE('',*,*,#29704,.F.);
#42344=ORIENTED_EDGE('',*,*,#30307,.F.);
#42345=ORIENTED_EDGE('',*,*,#29607,.F.);
#42346=ORIENTED_EDGE('',*,*,#30308,.F.);
#42347=ORIENTED_EDGE('',*,*,#30309,.T.);
#42348=ORIENTED_EDGE('',*,*,#30268,.T.);
#42349=ORIENTED_EDGE('',*,*,#29969,.T.);
#42350=ORIENTED_EDGE('',*,*,#29889,.T.);
#42351=ORIENTED_EDGE('',*,*,#30310,.F.);
#42352=ORIENTED_EDGE('',*,*,#30311,.F.);
#42353=ORIENTED_EDGE('',*,*,#29700,.F.);
#42354=ORIENTED_EDGE('',*,*,#30312,.F.);
#42355=ORIENTED_EDGE('',*,*,#29611,.F.);
#42356=ORIENTED_EDGE('',*,*,#30313,.F.);
#42357=ORIENTED_EDGE('',*,*,#30314,.T.);
#42358=ORIENTED_EDGE('',*,*,#30266,.T.);
#42359=ORIENTED_EDGE('',*,*,#29978,.T.);
#42360=ORIENTED_EDGE('',*,*,#29885,.T.);
#42361=ORIENTED_EDGE('',*,*,#30315,.F.);
#42362=ORIENTED_EDGE('',*,*,#30316,.F.);
#42363=ORIENTED_EDGE('',*,*,#29696,.F.);
#42364=ORIENTED_EDGE('',*,*,#30317,.F.);
#42365=ORIENTED_EDGE('',*,*,#29615,.F.);
#42366=ORIENTED_EDGE('',*,*,#30318,.F.);
#42367=ORIENTED_EDGE('',*,*,#30319,.T.);
#42368=ORIENTED_EDGE('',*,*,#30264,.T.);
#42369=ORIENTED_EDGE('',*,*,#29987,.T.);
#42370=ORIENTED_EDGE('',*,*,#29881,.T.);
#42371=ORIENTED_EDGE('',*,*,#30320,.F.);
#42372=ORIENTED_EDGE('',*,*,#30321,.F.);
#42373=ORIENTED_EDGE('',*,*,#29692,.F.);
#42374=ORIENTED_EDGE('',*,*,#30322,.F.);
#42375=ORIENTED_EDGE('',*,*,#29619,.F.);
#42376=ORIENTED_EDGE('',*,*,#30323,.F.);
#42377=ORIENTED_EDGE('',*,*,#30324,.T.);
#42378=ORIENTED_EDGE('',*,*,#30262,.T.);
#42379=ORIENTED_EDGE('',*,*,#29996,.T.);
#42380=ORIENTED_EDGE('',*,*,#29877,.T.);
#42381=ORIENTED_EDGE('',*,*,#30325,.F.);
#42382=ORIENTED_EDGE('',*,*,#30326,.F.);
#42383=ORIENTED_EDGE('',*,*,#29688,.F.);
#42384=ORIENTED_EDGE('',*,*,#30327,.F.);
#42385=ORIENTED_EDGE('',*,*,#29623,.F.);
#42386=ORIENTED_EDGE('',*,*,#30328,.F.);
#42387=ORIENTED_EDGE('',*,*,#30329,.T.);
#42388=ORIENTED_EDGE('',*,*,#30260,.T.);
#42389=ORIENTED_EDGE('',*,*,#30005,.T.);
#42390=ORIENTED_EDGE('',*,*,#29873,.T.);
#42391=ORIENTED_EDGE('',*,*,#30330,.F.);
#42392=ORIENTED_EDGE('',*,*,#30331,.F.);
#42393=ORIENTED_EDGE('',*,*,#29684,.F.);
#42394=ORIENTED_EDGE('',*,*,#29478,.F.);
#42395=ORIENTED_EDGE('',*,*,#29627,.F.);
#42396=ORIENTED_EDGE('',*,*,#30332,.F.);
#42397=ORIENTED_EDGE('',*,*,#30333,.T.);
#42398=ORIENTED_EDGE('',*,*,#30258,.T.);
#42399=ORIENTED_EDGE('',*,*,#30014,.T.);
#42400=ORIENTED_EDGE('',*,*,#29869,.T.);
#42401=ORIENTED_EDGE('',*,*,#30334,.F.);
#42402=ORIENTED_EDGE('',*,*,#30335,.F.);
#42403=ORIENTED_EDGE('',*,*,#29523,.F.);
#42404=ORIENTED_EDGE('',*,*,#30336,.F.);
#42405=ORIENTED_EDGE('',*,*,#29540,.F.);
#42406=ORIENTED_EDGE('',*,*,#30337,.F.);
#42407=ORIENTED_EDGE('',*,*,#30338,.T.);
#42408=ORIENTED_EDGE('',*,*,#30256,.T.);
#42409=ORIENTED_EDGE('',*,*,#30023,.T.);
#42410=ORIENTED_EDGE('',*,*,#29865,.T.);
#42411=ORIENTED_EDGE('',*,*,#30339,.F.);
#42412=ORIENTED_EDGE('',*,*,#30340,.F.);
#42413=ORIENTED_EDGE('',*,*,#29519,.F.);
#42414=ORIENTED_EDGE('',*,*,#30341,.F.);
#42415=ORIENTED_EDGE('',*,*,#29544,.F.);
#42416=ORIENTED_EDGE('',*,*,#30342,.F.);
#42417=ORIENTED_EDGE('',*,*,#30343,.T.);
#42418=ORIENTED_EDGE('',*,*,#30254,.T.);
#42419=ORIENTED_EDGE('',*,*,#30032,.T.);
#42420=ORIENTED_EDGE('',*,*,#29861,.T.);
#42421=ORIENTED_EDGE('',*,*,#30344,.F.);
#42422=ORIENTED_EDGE('',*,*,#30345,.F.);
#42423=ORIENTED_EDGE('',*,*,#29515,.F.);
#42424=ORIENTED_EDGE('',*,*,#30346,.F.);
#42425=ORIENTED_EDGE('',*,*,#29548,.F.);
#42426=ORIENTED_EDGE('',*,*,#30347,.F.);
#42427=ORIENTED_EDGE('',*,*,#30348,.T.);
#42428=ORIENTED_EDGE('',*,*,#30252,.T.);
#42429=ORIENTED_EDGE('',*,*,#30041,.T.);
#42430=ORIENTED_EDGE('',*,*,#29857,.T.);
#42431=ORIENTED_EDGE('',*,*,#30349,.F.);
#42432=ORIENTED_EDGE('',*,*,#30350,.F.);
#42433=ORIENTED_EDGE('',*,*,#29511,.F.);
#42434=ORIENTED_EDGE('',*,*,#30351,.F.);
#42435=ORIENTED_EDGE('',*,*,#29552,.F.);
#42436=ORIENTED_EDGE('',*,*,#30352,.F.);
#42437=ORIENTED_EDGE('',*,*,#30353,.T.);
#42438=ORIENTED_EDGE('',*,*,#30250,.T.);
#42439=ORIENTED_EDGE('',*,*,#30050,.T.);
#42440=ORIENTED_EDGE('',*,*,#29853,.T.);
#42441=ORIENTED_EDGE('',*,*,#30354,.F.);
#42442=ORIENTED_EDGE('',*,*,#30355,.F.);
#42443=ORIENTED_EDGE('',*,*,#29507,.F.);
#42444=ORIENTED_EDGE('',*,*,#30356,.F.);
#42445=ORIENTED_EDGE('',*,*,#29556,.F.);
#42446=ORIENTED_EDGE('',*,*,#30357,.F.);
#42447=ORIENTED_EDGE('',*,*,#30358,.T.);
#42448=ORIENTED_EDGE('',*,*,#30248,.T.);
#42449=ORIENTED_EDGE('',*,*,#30059,.T.);
#42450=ORIENTED_EDGE('',*,*,#29849,.T.);
#42451=ORIENTED_EDGE('',*,*,#30359,.F.);
#42452=ORIENTED_EDGE('',*,*,#30360,.F.);
#42453=ORIENTED_EDGE('',*,*,#29503,.F.);
#42454=ORIENTED_EDGE('',*,*,#30361,.F.);
#42455=ORIENTED_EDGE('',*,*,#29560,.F.);
#42456=ORIENTED_EDGE('',*,*,#30362,.F.);
#42457=ORIENTED_EDGE('',*,*,#30363,.T.);
#42458=ORIENTED_EDGE('',*,*,#30246,.T.);
#42459=ORIENTED_EDGE('',*,*,#30068,.T.);
#42460=ORIENTED_EDGE('',*,*,#29845,.T.);
#42461=ORIENTED_EDGE('',*,*,#30364,.F.);
#42462=ORIENTED_EDGE('',*,*,#30365,.F.);
#42463=ORIENTED_EDGE('',*,*,#29499,.F.);
#42464=ORIENTED_EDGE('',*,*,#30366,.F.);
#42465=ORIENTED_EDGE('',*,*,#29564,.F.);
#42466=ORIENTED_EDGE('',*,*,#30367,.F.);
#42467=ORIENTED_EDGE('',*,*,#30368,.T.);
#42468=ORIENTED_EDGE('',*,*,#30244,.T.);
#42469=ORIENTED_EDGE('',*,*,#30077,.T.);
#42470=ORIENTED_EDGE('',*,*,#29841,.T.);
#42471=ORIENTED_EDGE('',*,*,#30369,.F.);
#42472=ORIENTED_EDGE('',*,*,#30370,.F.);
#42473=ORIENTED_EDGE('',*,*,#29495,.F.);
#42474=ORIENTED_EDGE('',*,*,#30371,.F.);
#42475=ORIENTED_EDGE('',*,*,#29568,.F.);
#42476=ORIENTED_EDGE('',*,*,#30372,.F.);
#42477=ORIENTED_EDGE('',*,*,#30373,.T.);
#42478=ORIENTED_EDGE('',*,*,#30242,.T.);
#42479=ORIENTED_EDGE('',*,*,#30086,.T.);
#42480=ORIENTED_EDGE('',*,*,#29837,.T.);
#42481=ORIENTED_EDGE('',*,*,#30374,.F.);
#42482=ORIENTED_EDGE('',*,*,#30375,.F.);
#42483=ORIENTED_EDGE('',*,*,#29491,.F.);
#42484=ORIENTED_EDGE('',*,*,#30376,.F.);
#42485=ORIENTED_EDGE('',*,*,#29572,.F.);
#42486=ORIENTED_EDGE('',*,*,#30377,.F.);
#42487=ORIENTED_EDGE('',*,*,#30378,.T.);
#42488=ORIENTED_EDGE('',*,*,#30240,.T.);
#42489=ORIENTED_EDGE('',*,*,#30095,.T.);
#42490=ORIENTED_EDGE('',*,*,#29833,.T.);
#42491=ORIENTED_EDGE('',*,*,#30379,.F.);
#42492=ORIENTED_EDGE('',*,*,#30380,.F.);
#42493=ORIENTED_EDGE('',*,*,#29487,.F.);
#42494=ORIENTED_EDGE('',*,*,#30381,.F.);
#42495=ORIENTED_EDGE('',*,*,#29576,.F.);
#42496=ORIENTED_EDGE('',*,*,#30382,.F.);
#42497=ORIENTED_EDGE('',*,*,#30383,.T.);
#42498=ORIENTED_EDGE('',*,*,#30238,.T.);
#42499=ORIENTED_EDGE('',*,*,#30104,.T.);
#42500=ORIENTED_EDGE('',*,*,#29829,.T.);
#42501=ORIENTED_EDGE('',*,*,#30384,.F.);
#42502=ORIENTED_EDGE('',*,*,#30385,.F.);
#42503=ORIENTED_EDGE('',*,*,#29483,.F.);
#42504=ORIENTED_EDGE('',*,*,#29730,.F.);
#42505=ORIENTED_EDGE('',*,*,#29580,.F.);
#42506=ORIENTED_EDGE('',*,*,#30386,.F.);
#42507=ORIENTED_EDGE('',*,*,#30387,.T.);
#42508=ORIENTED_EDGE('',*,*,#30236,.T.);
#42509=ORIENTED_EDGE('',*,*,#30113,.T.);
#42510=ORIENTED_EDGE('',*,*,#29825,.T.);
#42511=ORIENTED_EDGE('',*,*,#30388,.F.);
#42512=ORIENTED_EDGE('',*,*,#30389,.F.);
#42513=ORIENTED_EDGE('',*,*,#29680,.F.);
#42514=ORIENTED_EDGE('',*,*,#30390,.F.);
#42515=ORIENTED_EDGE('',*,*,#29734,.F.);
#42516=ORIENTED_EDGE('',*,*,#30391,.F.);
#42517=ORIENTED_EDGE('',*,*,#30392,.T.);
#42518=ORIENTED_EDGE('',*,*,#30234,.T.);
#42519=ORIENTED_EDGE('',*,*,#30122,.T.);
#42520=ORIENTED_EDGE('',*,*,#29821,.T.);
#42521=ORIENTED_EDGE('',*,*,#30393,.F.);
#42522=ORIENTED_EDGE('',*,*,#30394,.F.);
#42523=ORIENTED_EDGE('',*,*,#29676,.F.);
#42524=ORIENTED_EDGE('',*,*,#30395,.F.);
#42525=ORIENTED_EDGE('',*,*,#29738,.F.);
#42526=ORIENTED_EDGE('',*,*,#30396,.F.);
#42527=ORIENTED_EDGE('',*,*,#30397,.T.);
#42528=ORIENTED_EDGE('',*,*,#30232,.T.);
#42529=ORIENTED_EDGE('',*,*,#30131,.T.);
#42530=ORIENTED_EDGE('',*,*,#29817,.T.);
#42531=ORIENTED_EDGE('',*,*,#30398,.F.);
#42532=ORIENTED_EDGE('',*,*,#30399,.F.);
#42533=ORIENTED_EDGE('',*,*,#29672,.F.);
#42534=ORIENTED_EDGE('',*,*,#30400,.F.);
#42535=ORIENTED_EDGE('',*,*,#29742,.F.);
#42536=ORIENTED_EDGE('',*,*,#30401,.F.);
#42537=ORIENTED_EDGE('',*,*,#30402,.T.);
#42538=ORIENTED_EDGE('',*,*,#30230,.T.);
#42539=ORIENTED_EDGE('',*,*,#30140,.T.);
#42540=ORIENTED_EDGE('',*,*,#29813,.T.);
#42541=ORIENTED_EDGE('',*,*,#30403,.F.);
#42542=ORIENTED_EDGE('',*,*,#30404,.F.);
#42543=ORIENTED_EDGE('',*,*,#29668,.F.);
#42544=ORIENTED_EDGE('',*,*,#30405,.F.);
#42545=ORIENTED_EDGE('',*,*,#29746,.F.);
#42546=ORIENTED_EDGE('',*,*,#30406,.F.);
#42547=ORIENTED_EDGE('',*,*,#30407,.T.);
#42548=ORIENTED_EDGE('',*,*,#30228,.T.);
#42549=ORIENTED_EDGE('',*,*,#30149,.T.);
#42550=ORIENTED_EDGE('',*,*,#29809,.T.);
#42551=ORIENTED_EDGE('',*,*,#30408,.F.);
#42552=ORIENTED_EDGE('',*,*,#30409,.F.);
#42553=ORIENTED_EDGE('',*,*,#29664,.F.);
#42554=ORIENTED_EDGE('',*,*,#30410,.F.);
#42555=ORIENTED_EDGE('',*,*,#29750,.F.);
#42556=ORIENTED_EDGE('',*,*,#30411,.F.);
#42557=ORIENTED_EDGE('',*,*,#30412,.T.);
#42558=ORIENTED_EDGE('',*,*,#30226,.T.);
#42559=ORIENTED_EDGE('',*,*,#30158,.T.);
#42560=ORIENTED_EDGE('',*,*,#29805,.T.);
#42561=ORIENTED_EDGE('',*,*,#30413,.F.);
#42562=ORIENTED_EDGE('',*,*,#30414,.F.);
#42563=ORIENTED_EDGE('',*,*,#29660,.F.);
#42564=ORIENTED_EDGE('',*,*,#30415,.F.);
#42565=ORIENTED_EDGE('',*,*,#29754,.F.);
#42566=ORIENTED_EDGE('',*,*,#30416,.F.);
#42567=ORIENTED_EDGE('',*,*,#30417,.T.);
#42568=ORIENTED_EDGE('',*,*,#30224,.T.);
#42569=ORIENTED_EDGE('',*,*,#30167,.T.);
#42570=ORIENTED_EDGE('',*,*,#29801,.T.);
#42571=ORIENTED_EDGE('',*,*,#30418,.F.);
#42572=ORIENTED_EDGE('',*,*,#30419,.F.);
#42573=ORIENTED_EDGE('',*,*,#29656,.F.);
#42574=ORIENTED_EDGE('',*,*,#30420,.F.);
#42575=ORIENTED_EDGE('',*,*,#29758,.F.);
#42576=ORIENTED_EDGE('',*,*,#30421,.F.);
#42577=ORIENTED_EDGE('',*,*,#30422,.T.);
#42578=ORIENTED_EDGE('',*,*,#30222,.T.);
#42579=ORIENTED_EDGE('',*,*,#30176,.T.);
#42580=ORIENTED_EDGE('',*,*,#29797,.T.);
#42581=ORIENTED_EDGE('',*,*,#30423,.F.);
#42582=ORIENTED_EDGE('',*,*,#30424,.F.);
#42583=ORIENTED_EDGE('',*,*,#29652,.F.);
#42584=ORIENTED_EDGE('',*,*,#30425,.F.);
#42585=ORIENTED_EDGE('',*,*,#29762,.F.);
#42586=ORIENTED_EDGE('',*,*,#30426,.F.);
#42587=ORIENTED_EDGE('',*,*,#30427,.T.);
#42588=ORIENTED_EDGE('',*,*,#30220,.T.);
#42589=ORIENTED_EDGE('',*,*,#30185,.T.);
#42590=ORIENTED_EDGE('',*,*,#29793,.T.);
#42591=ORIENTED_EDGE('',*,*,#30428,.F.);
#42592=ORIENTED_EDGE('',*,*,#30429,.F.);
#42593=ORIENTED_EDGE('',*,*,#29648,.F.);
#42594=ORIENTED_EDGE('',*,*,#30430,.F.);
#42595=ORIENTED_EDGE('',*,*,#29766,.F.);
#42596=ORIENTED_EDGE('',*,*,#30431,.F.);
#42597=ORIENTED_EDGE('',*,*,#30432,.T.);
#42598=ORIENTED_EDGE('',*,*,#30218,.T.);
#42599=ORIENTED_EDGE('',*,*,#30194,.T.);
#42600=ORIENTED_EDGE('',*,*,#29789,.T.);
#42601=ORIENTED_EDGE('',*,*,#30433,.F.);
#42602=ORIENTED_EDGE('',*,*,#30434,.F.);
#42603=ORIENTED_EDGE('',*,*,#29644,.F.);
#42604=ORIENTED_EDGE('',*,*,#30435,.F.);
#42605=ORIENTED_EDGE('',*,*,#29770,.F.);
#42606=ORIENTED_EDGE('',*,*,#30436,.F.);
#42607=ORIENTED_EDGE('',*,*,#30437,.T.);
#42608=ORIENTED_EDGE('',*,*,#30216,.T.);
#42609=ORIENTED_EDGE('',*,*,#30203,.T.);
#42610=ORIENTED_EDGE('',*,*,#29785,.T.);
#42611=ORIENTED_EDGE('',*,*,#30438,.F.);
#42612=ORIENTED_EDGE('',*,*,#30439,.F.);
#42613=ORIENTED_EDGE('',*,*,#29640,.F.);
#42614=ORIENTED_EDGE('',*,*,#29784,.F.);
#42615=ORIENTED_EDGE('',*,*,#29774,.F.);
#42616=ORIENTED_EDGE('',*,*,#30440,.F.);
#42617=ORIENTED_EDGE('',*,*,#30441,.T.);
#42618=ORIENTED_EDGE('',*,*,#30214,.T.);
#42619=ORIENTED_EDGE('',*,*,#30212,.T.);
#42620=ORIENTED_EDGE('',*,*,#29586,.F.);
#42621=ORIENTED_EDGE('',*,*,#29920,.F.);
#42622=ORIENTED_EDGE('',*,*,#30442,.T.);
#42623=ORIENTED_EDGE('',*,*,#30283,.T.);
#42624=ORIENTED_EDGE('',*,*,#29725,.F.);
#42625=ORIENTED_EDGE('',*,*,#30281,.T.);
#42626=ORIENTED_EDGE('',*,*,#30443,.F.);
#42627=ORIENTED_EDGE('',*,*,#29922,.F.);
#42628=ORIENTED_EDGE('',*,*,#29916,.T.);
#42629=ORIENTED_EDGE('',*,*,#29923,.T.);
#42630=ORIENTED_EDGE('',*,*,#30443,.T.);
#42631=ORIENTED_EDGE('',*,*,#30280,.T.);
#42632=ORIENTED_EDGE('',*,*,#30279,.T.);
#42633=ORIENTED_EDGE('',*,*,#30284,.F.);
#42634=ORIENTED_EDGE('',*,*,#30442,.F.);
#42635=ORIENTED_EDGE('',*,*,#29919,.F.);
#42636=ORIENTED_EDGE('',*,*,#30282,.T.);
#42637=ORIENTED_EDGE('',*,*,#29723,.F.);
#42638=ORIENTED_EDGE('',*,*,#29930,.T.);
#42639=ORIENTED_EDGE('',*,*,#29588,.T.);
#42640=ORIENTED_EDGE('',*,*,#29780,.T.);
#42641=ORIENTED_EDGE('',*,*,#29727,.F.);
#42642=ORIENTED_EDGE('',*,*,#29921,.T.);
#42643=ORIENTED_EDGE('',*,*,#29584,.T.);
#42644=ORIENTED_EDGE('',*,*,#29590,.F.);
#42645=ORIENTED_EDGE('',*,*,#29929,.F.);
#42646=ORIENTED_EDGE('',*,*,#30444,.T.);
#42647=ORIENTED_EDGE('',*,*,#30288,.T.);
#42648=ORIENTED_EDGE('',*,*,#29721,.F.);
#42649=ORIENTED_EDGE('',*,*,#30286,.T.);
#42650=ORIENTED_EDGE('',*,*,#30445,.F.);
#42651=ORIENTED_EDGE('',*,*,#29931,.F.);
#42652=ORIENTED_EDGE('',*,*,#29912,.T.);
#42653=ORIENTED_EDGE('',*,*,#29932,.T.);
#42654=ORIENTED_EDGE('',*,*,#30445,.T.);
#42655=ORIENTED_EDGE('',*,*,#30285,.T.);
#42656=ORIENTED_EDGE('',*,*,#30277,.T.);
#42657=ORIENTED_EDGE('',*,*,#30289,.F.);
#42658=ORIENTED_EDGE('',*,*,#30444,.F.);
#42659=ORIENTED_EDGE('',*,*,#29928,.F.);
#42660=ORIENTED_EDGE('',*,*,#30287,.T.);
#42661=ORIENTED_EDGE('',*,*,#29719,.F.);
#42662=ORIENTED_EDGE('',*,*,#29939,.T.);
#42663=ORIENTED_EDGE('',*,*,#29592,.T.);
#42664=ORIENTED_EDGE('',*,*,#29594,.F.);
#42665=ORIENTED_EDGE('',*,*,#29938,.F.);
#42666=ORIENTED_EDGE('',*,*,#30446,.T.);
#42667=ORIENTED_EDGE('',*,*,#30293,.T.);
#42668=ORIENTED_EDGE('',*,*,#29717,.F.);
#42669=ORIENTED_EDGE('',*,*,#30291,.T.);
#42670=ORIENTED_EDGE('',*,*,#30447,.F.);
#42671=ORIENTED_EDGE('',*,*,#29940,.F.);
#42672=ORIENTED_EDGE('',*,*,#29908,.T.);
#42673=ORIENTED_EDGE('',*,*,#29941,.T.);
#42674=ORIENTED_EDGE('',*,*,#30447,.T.);
#42675=ORIENTED_EDGE('',*,*,#30290,.T.);
#42676=ORIENTED_EDGE('',*,*,#30275,.T.);
#42677=ORIENTED_EDGE('',*,*,#30294,.F.);
#42678=ORIENTED_EDGE('',*,*,#30446,.F.);
#42679=ORIENTED_EDGE('',*,*,#29937,.F.);
#42680=ORIENTED_EDGE('',*,*,#30292,.T.);
#42681=ORIENTED_EDGE('',*,*,#29715,.F.);
#42682=ORIENTED_EDGE('',*,*,#29948,.T.);
#42683=ORIENTED_EDGE('',*,*,#29596,.T.);
#42684=ORIENTED_EDGE('',*,*,#29598,.F.);
#42685=ORIENTED_EDGE('',*,*,#29947,.F.);
#42686=ORIENTED_EDGE('',*,*,#30448,.T.);
#42687=ORIENTED_EDGE('',*,*,#30298,.T.);
#42688=ORIENTED_EDGE('',*,*,#29713,.F.);
#42689=ORIENTED_EDGE('',*,*,#30296,.T.);
#42690=ORIENTED_EDGE('',*,*,#30449,.F.);
#42691=ORIENTED_EDGE('',*,*,#29949,.F.);
#42692=ORIENTED_EDGE('',*,*,#29904,.T.);
#42693=ORIENTED_EDGE('',*,*,#29950,.T.);
#42694=ORIENTED_EDGE('',*,*,#30449,.T.);
#42695=ORIENTED_EDGE('',*,*,#30295,.T.);
#42696=ORIENTED_EDGE('',*,*,#30273,.T.);
#42697=ORIENTED_EDGE('',*,*,#30299,.F.);
#42698=ORIENTED_EDGE('',*,*,#30448,.F.);
#42699=ORIENTED_EDGE('',*,*,#29946,.F.);
#42700=ORIENTED_EDGE('',*,*,#30297,.T.);
#42701=ORIENTED_EDGE('',*,*,#29711,.F.);
#42702=ORIENTED_EDGE('',*,*,#29957,.T.);
#42703=ORIENTED_EDGE('',*,*,#29600,.T.);
#42704=ORIENTED_EDGE('',*,*,#29602,.F.);
#42705=ORIENTED_EDGE('',*,*,#29956,.F.);
#42706=ORIENTED_EDGE('',*,*,#30450,.T.);
#42707=ORIENTED_EDGE('',*,*,#30303,.T.);
#42708=ORIENTED_EDGE('',*,*,#29709,.F.);
#42709=ORIENTED_EDGE('',*,*,#30301,.T.);
#42710=ORIENTED_EDGE('',*,*,#30451,.F.);
#42711=ORIENTED_EDGE('',*,*,#29958,.F.);
#42712=ORIENTED_EDGE('',*,*,#29900,.T.);
#42713=ORIENTED_EDGE('',*,*,#29959,.T.);
#42714=ORIENTED_EDGE('',*,*,#30451,.T.);
#42715=ORIENTED_EDGE('',*,*,#30300,.T.);
#42716=ORIENTED_EDGE('',*,*,#30271,.T.);
#42717=ORIENTED_EDGE('',*,*,#30304,.F.);
#42718=ORIENTED_EDGE('',*,*,#30450,.F.);
#42719=ORIENTED_EDGE('',*,*,#29955,.F.);
#42720=ORIENTED_EDGE('',*,*,#30302,.T.);
#42721=ORIENTED_EDGE('',*,*,#29707,.F.);
#42722=ORIENTED_EDGE('',*,*,#29966,.T.);
#42723=ORIENTED_EDGE('',*,*,#29604,.T.);
#42724=ORIENTED_EDGE('',*,*,#29606,.F.);
#42725=ORIENTED_EDGE('',*,*,#29965,.F.);
#42726=ORIENTED_EDGE('',*,*,#30452,.T.);
#42727=ORIENTED_EDGE('',*,*,#30308,.T.);
#42728=ORIENTED_EDGE('',*,*,#29705,.F.);
#42729=ORIENTED_EDGE('',*,*,#30306,.T.);
#42730=ORIENTED_EDGE('',*,*,#30453,.F.);
#42731=ORIENTED_EDGE('',*,*,#29967,.F.);
#42732=ORIENTED_EDGE('',*,*,#29896,.T.);
#42733=ORIENTED_EDGE('',*,*,#29968,.T.);
#42734=ORIENTED_EDGE('',*,*,#30453,.T.);
#42735=ORIENTED_EDGE('',*,*,#30305,.T.);
#42736=ORIENTED_EDGE('',*,*,#30269,.T.);
#42737=ORIENTED_EDGE('',*,*,#30309,.F.);
#42738=ORIENTED_EDGE('',*,*,#30452,.F.);
#42739=ORIENTED_EDGE('',*,*,#29964,.F.);
#42740=ORIENTED_EDGE('',*,*,#30307,.T.);
#42741=ORIENTED_EDGE('',*,*,#29703,.F.);
#42742=ORIENTED_EDGE('',*,*,#29975,.T.);
#42743=ORIENTED_EDGE('',*,*,#29608,.T.);
#42744=ORIENTED_EDGE('',*,*,#29610,.F.);
#42745=ORIENTED_EDGE('',*,*,#29974,.F.);
#42746=ORIENTED_EDGE('',*,*,#30454,.T.);
#42747=ORIENTED_EDGE('',*,*,#30313,.T.);
#42748=ORIENTED_EDGE('',*,*,#29701,.F.);
#42749=ORIENTED_EDGE('',*,*,#30311,.T.);
#42750=ORIENTED_EDGE('',*,*,#30455,.F.);
#42751=ORIENTED_EDGE('',*,*,#29976,.F.);
#42752=ORIENTED_EDGE('',*,*,#29892,.T.);
#42753=ORIENTED_EDGE('',*,*,#29977,.T.);
#42754=ORIENTED_EDGE('',*,*,#30455,.T.);
#42755=ORIENTED_EDGE('',*,*,#30310,.T.);
#42756=ORIENTED_EDGE('',*,*,#30267,.T.);
#42757=ORIENTED_EDGE('',*,*,#30314,.F.);
#42758=ORIENTED_EDGE('',*,*,#30454,.F.);
#42759=ORIENTED_EDGE('',*,*,#29973,.F.);
#42760=ORIENTED_EDGE('',*,*,#30312,.T.);
#42761=ORIENTED_EDGE('',*,*,#29699,.F.);
#42762=ORIENTED_EDGE('',*,*,#29984,.T.);
#42763=ORIENTED_EDGE('',*,*,#29612,.T.);
#42764=ORIENTED_EDGE('',*,*,#29614,.F.);
#42765=ORIENTED_EDGE('',*,*,#29983,.F.);
#42766=ORIENTED_EDGE('',*,*,#30456,.T.);
#42767=ORIENTED_EDGE('',*,*,#30318,.T.);
#42768=ORIENTED_EDGE('',*,*,#29697,.F.);
#42769=ORIENTED_EDGE('',*,*,#30316,.T.);
#42770=ORIENTED_EDGE('',*,*,#30457,.F.);
#42771=ORIENTED_EDGE('',*,*,#29985,.F.);
#42772=ORIENTED_EDGE('',*,*,#29888,.T.);
#42773=ORIENTED_EDGE('',*,*,#29986,.T.);
#42774=ORIENTED_EDGE('',*,*,#30457,.T.);
#42775=ORIENTED_EDGE('',*,*,#30315,.T.);
#42776=ORIENTED_EDGE('',*,*,#30265,.T.);
#42777=ORIENTED_EDGE('',*,*,#30319,.F.);
#42778=ORIENTED_EDGE('',*,*,#30456,.F.);
#42779=ORIENTED_EDGE('',*,*,#29982,.F.);
#42780=ORIENTED_EDGE('',*,*,#30317,.T.);
#42781=ORIENTED_EDGE('',*,*,#29695,.F.);
#42782=ORIENTED_EDGE('',*,*,#29993,.T.);
#42783=ORIENTED_EDGE('',*,*,#29616,.T.);
#42784=ORIENTED_EDGE('',*,*,#29618,.F.);
#42785=ORIENTED_EDGE('',*,*,#29992,.F.);
#42786=ORIENTED_EDGE('',*,*,#30458,.T.);
#42787=ORIENTED_EDGE('',*,*,#30323,.T.);
#42788=ORIENTED_EDGE('',*,*,#29693,.F.);
#42789=ORIENTED_EDGE('',*,*,#30321,.T.);
#42790=ORIENTED_EDGE('',*,*,#30459,.F.);
#42791=ORIENTED_EDGE('',*,*,#29994,.F.);
#42792=ORIENTED_EDGE('',*,*,#29884,.T.);
#42793=ORIENTED_EDGE('',*,*,#29995,.T.);
#42794=ORIENTED_EDGE('',*,*,#30459,.T.);
#42795=ORIENTED_EDGE('',*,*,#30320,.T.);
#42796=ORIENTED_EDGE('',*,*,#30263,.T.);
#42797=ORIENTED_EDGE('',*,*,#30324,.F.);
#42798=ORIENTED_EDGE('',*,*,#30458,.F.);
#42799=ORIENTED_EDGE('',*,*,#29991,.F.);
#42800=ORIENTED_EDGE('',*,*,#30322,.T.);
#42801=ORIENTED_EDGE('',*,*,#29691,.F.);
#42802=ORIENTED_EDGE('',*,*,#30002,.T.);
#42803=ORIENTED_EDGE('',*,*,#29620,.T.);
#42804=ORIENTED_EDGE('',*,*,#29622,.F.);
#42805=ORIENTED_EDGE('',*,*,#30001,.F.);
#42806=ORIENTED_EDGE('',*,*,#30460,.T.);
#42807=ORIENTED_EDGE('',*,*,#30328,.T.);
#42808=ORIENTED_EDGE('',*,*,#29689,.F.);
#42809=ORIENTED_EDGE('',*,*,#30326,.T.);
#42810=ORIENTED_EDGE('',*,*,#30461,.F.);
#42811=ORIENTED_EDGE('',*,*,#30003,.F.);
#42812=ORIENTED_EDGE('',*,*,#29880,.T.);
#42813=ORIENTED_EDGE('',*,*,#30004,.T.);
#42814=ORIENTED_EDGE('',*,*,#30461,.T.);
#42815=ORIENTED_EDGE('',*,*,#30325,.T.);
#42816=ORIENTED_EDGE('',*,*,#30261,.T.);
#42817=ORIENTED_EDGE('',*,*,#30329,.F.);
#42818=ORIENTED_EDGE('',*,*,#30460,.F.);
#42819=ORIENTED_EDGE('',*,*,#30000,.F.);
#42820=ORIENTED_EDGE('',*,*,#30327,.T.);
#42821=ORIENTED_EDGE('',*,*,#29687,.F.);
#42822=ORIENTED_EDGE('',*,*,#30011,.T.);
#42823=ORIENTED_EDGE('',*,*,#29624,.T.);
#42824=ORIENTED_EDGE('',*,*,#29626,.F.);
#42825=ORIENTED_EDGE('',*,*,#30010,.F.);
#42826=ORIENTED_EDGE('',*,*,#30462,.T.);
#42827=ORIENTED_EDGE('',*,*,#30332,.T.);
#42828=ORIENTED_EDGE('',*,*,#29685,.F.);
#42829=ORIENTED_EDGE('',*,*,#30331,.T.);
#42830=ORIENTED_EDGE('',*,*,#30463,.F.);
#42831=ORIENTED_EDGE('',*,*,#30012,.F.);
#42832=ORIENTED_EDGE('',*,*,#29876,.T.);
#42833=ORIENTED_EDGE('',*,*,#30013,.T.);
#42834=ORIENTED_EDGE('',*,*,#30463,.T.);
#42835=ORIENTED_EDGE('',*,*,#30330,.T.);
#42836=ORIENTED_EDGE('',*,*,#30259,.T.);
#42837=ORIENTED_EDGE('',*,*,#30333,.F.);
#42838=ORIENTED_EDGE('',*,*,#30462,.F.);
#42839=ORIENTED_EDGE('',*,*,#30009,.F.);
#42840=ORIENTED_EDGE('',*,*,#29470,.T.);
#42841=ORIENTED_EDGE('',*,*,#29526,.F.);
#42842=ORIENTED_EDGE('',*,*,#30020,.T.);
#42843=ORIENTED_EDGE('',*,*,#29537,.T.);
#42844=ORIENTED_EDGE('',*,*,#29539,.F.);
#42845=ORIENTED_EDGE('',*,*,#30019,.F.);
#42846=ORIENTED_EDGE('',*,*,#30464,.T.);
#42847=ORIENTED_EDGE('',*,*,#30337,.T.);
#42848=ORIENTED_EDGE('',*,*,#29524,.F.);
#42849=ORIENTED_EDGE('',*,*,#30335,.T.);
#42850=ORIENTED_EDGE('',*,*,#30465,.F.);
#42851=ORIENTED_EDGE('',*,*,#30021,.F.);
#42852=ORIENTED_EDGE('',*,*,#29872,.T.);
#42853=ORIENTED_EDGE('',*,*,#30022,.T.);
#42854=ORIENTED_EDGE('',*,*,#30465,.T.);
#42855=ORIENTED_EDGE('',*,*,#30334,.T.);
#42856=ORIENTED_EDGE('',*,*,#30257,.T.);
#42857=ORIENTED_EDGE('',*,*,#30338,.F.);
#42858=ORIENTED_EDGE('',*,*,#30464,.F.);
#42859=ORIENTED_EDGE('',*,*,#30018,.F.);
#42860=ORIENTED_EDGE('',*,*,#30336,.T.);
#42861=ORIENTED_EDGE('',*,*,#29522,.F.);
#42862=ORIENTED_EDGE('',*,*,#30029,.T.);
#42863=ORIENTED_EDGE('',*,*,#29541,.T.);
#42864=ORIENTED_EDGE('',*,*,#29543,.F.);
#42865=ORIENTED_EDGE('',*,*,#30028,.F.);
#42866=ORIENTED_EDGE('',*,*,#30466,.T.);
#42867=ORIENTED_EDGE('',*,*,#30342,.T.);
#42868=ORIENTED_EDGE('',*,*,#29520,.F.);
#42869=ORIENTED_EDGE('',*,*,#30340,.T.);
#42870=ORIENTED_EDGE('',*,*,#30467,.F.);
#42871=ORIENTED_EDGE('',*,*,#30030,.F.);
#42872=ORIENTED_EDGE('',*,*,#29868,.T.);
#42873=ORIENTED_EDGE('',*,*,#30031,.T.);
#42874=ORIENTED_EDGE('',*,*,#30467,.T.);
#42875=ORIENTED_EDGE('',*,*,#30339,.T.);
#42876=ORIENTED_EDGE('',*,*,#30255,.T.);
#42877=ORIENTED_EDGE('',*,*,#30343,.F.);
#42878=ORIENTED_EDGE('',*,*,#30466,.F.);
#42879=ORIENTED_EDGE('',*,*,#30027,.F.);
#42880=ORIENTED_EDGE('',*,*,#30341,.T.);
#42881=ORIENTED_EDGE('',*,*,#29518,.F.);
#42882=ORIENTED_EDGE('',*,*,#30038,.T.);
#42883=ORIENTED_EDGE('',*,*,#29545,.T.);
#42884=ORIENTED_EDGE('',*,*,#29547,.F.);
#42885=ORIENTED_EDGE('',*,*,#30037,.F.);
#42886=ORIENTED_EDGE('',*,*,#30468,.T.);
#42887=ORIENTED_EDGE('',*,*,#30347,.T.);
#42888=ORIENTED_EDGE('',*,*,#29516,.F.);
#42889=ORIENTED_EDGE('',*,*,#30345,.T.);
#42890=ORIENTED_EDGE('',*,*,#30469,.F.);
#42891=ORIENTED_EDGE('',*,*,#30039,.F.);
#42892=ORIENTED_EDGE('',*,*,#29864,.T.);
#42893=ORIENTED_EDGE('',*,*,#30040,.T.);
#42894=ORIENTED_EDGE('',*,*,#30469,.T.);
#42895=ORIENTED_EDGE('',*,*,#30344,.T.);
#42896=ORIENTED_EDGE('',*,*,#30253,.T.);
#42897=ORIENTED_EDGE('',*,*,#30348,.F.);
#42898=ORIENTED_EDGE('',*,*,#30468,.F.);
#42899=ORIENTED_EDGE('',*,*,#30036,.F.);
#42900=ORIENTED_EDGE('',*,*,#30346,.T.);
#42901=ORIENTED_EDGE('',*,*,#29514,.F.);
#42902=ORIENTED_EDGE('',*,*,#30047,.T.);
#42903=ORIENTED_EDGE('',*,*,#29549,.T.);
#42904=ORIENTED_EDGE('',*,*,#29551,.F.);
#42905=ORIENTED_EDGE('',*,*,#30046,.F.);
#42906=ORIENTED_EDGE('',*,*,#30470,.T.);
#42907=ORIENTED_EDGE('',*,*,#30352,.T.);
#42908=ORIENTED_EDGE('',*,*,#29512,.F.);
#42909=ORIENTED_EDGE('',*,*,#30350,.T.);
#42910=ORIENTED_EDGE('',*,*,#30471,.F.);
#42911=ORIENTED_EDGE('',*,*,#30048,.F.);
#42912=ORIENTED_EDGE('',*,*,#29860,.T.);
#42913=ORIENTED_EDGE('',*,*,#30049,.T.);
#42914=ORIENTED_EDGE('',*,*,#30471,.T.);
#42915=ORIENTED_EDGE('',*,*,#30349,.T.);
#42916=ORIENTED_EDGE('',*,*,#30251,.T.);
#42917=ORIENTED_EDGE('',*,*,#30353,.F.);
#42918=ORIENTED_EDGE('',*,*,#30470,.F.);
#42919=ORIENTED_EDGE('',*,*,#30045,.F.);
#42920=ORIENTED_EDGE('',*,*,#30351,.T.);
#42921=ORIENTED_EDGE('',*,*,#29510,.F.);
#42922=ORIENTED_EDGE('',*,*,#30056,.T.);
#42923=ORIENTED_EDGE('',*,*,#29553,.T.);
#42924=ORIENTED_EDGE('',*,*,#29555,.F.);
#42925=ORIENTED_EDGE('',*,*,#30055,.F.);
#42926=ORIENTED_EDGE('',*,*,#30472,.T.);
#42927=ORIENTED_EDGE('',*,*,#30357,.T.);
#42928=ORIENTED_EDGE('',*,*,#29508,.F.);
#42929=ORIENTED_EDGE('',*,*,#30355,.T.);
#42930=ORIENTED_EDGE('',*,*,#30473,.F.);
#42931=ORIENTED_EDGE('',*,*,#30057,.F.);
#42932=ORIENTED_EDGE('',*,*,#29856,.T.);
#42933=ORIENTED_EDGE('',*,*,#30058,.T.);
#42934=ORIENTED_EDGE('',*,*,#30473,.T.);
#42935=ORIENTED_EDGE('',*,*,#30354,.T.);
#42936=ORIENTED_EDGE('',*,*,#30249,.T.);
#42937=ORIENTED_EDGE('',*,*,#30358,.F.);
#42938=ORIENTED_EDGE('',*,*,#30472,.F.);
#42939=ORIENTED_EDGE('',*,*,#30054,.F.);
#42940=ORIENTED_EDGE('',*,*,#30356,.T.);
#42941=ORIENTED_EDGE('',*,*,#29506,.F.);
#42942=ORIENTED_EDGE('',*,*,#30065,.T.);
#42943=ORIENTED_EDGE('',*,*,#29557,.T.);
#42944=ORIENTED_EDGE('',*,*,#29559,.F.);
#42945=ORIENTED_EDGE('',*,*,#30064,.F.);
#42946=ORIENTED_EDGE('',*,*,#30474,.T.);
#42947=ORIENTED_EDGE('',*,*,#30362,.T.);
#42948=ORIENTED_EDGE('',*,*,#29504,.F.);
#42949=ORIENTED_EDGE('',*,*,#30360,.T.);
#42950=ORIENTED_EDGE('',*,*,#30475,.F.);
#42951=ORIENTED_EDGE('',*,*,#30066,.F.);
#42952=ORIENTED_EDGE('',*,*,#29852,.T.);
#42953=ORIENTED_EDGE('',*,*,#30067,.T.);
#42954=ORIENTED_EDGE('',*,*,#30475,.T.);
#42955=ORIENTED_EDGE('',*,*,#30359,.T.);
#42956=ORIENTED_EDGE('',*,*,#30247,.T.);
#42957=ORIENTED_EDGE('',*,*,#30363,.F.);
#42958=ORIENTED_EDGE('',*,*,#30474,.F.);
#42959=ORIENTED_EDGE('',*,*,#30063,.F.);
#42960=ORIENTED_EDGE('',*,*,#30361,.T.);
#42961=ORIENTED_EDGE('',*,*,#29502,.F.);
#42962=ORIENTED_EDGE('',*,*,#30074,.T.);
#42963=ORIENTED_EDGE('',*,*,#29561,.T.);
#42964=ORIENTED_EDGE('',*,*,#29563,.F.);
#42965=ORIENTED_EDGE('',*,*,#30073,.F.);
#42966=ORIENTED_EDGE('',*,*,#30476,.T.);
#42967=ORIENTED_EDGE('',*,*,#30367,.T.);
#42968=ORIENTED_EDGE('',*,*,#29500,.F.);
#42969=ORIENTED_EDGE('',*,*,#30365,.T.);
#42970=ORIENTED_EDGE('',*,*,#30477,.F.);
#42971=ORIENTED_EDGE('',*,*,#30075,.F.);
#42972=ORIENTED_EDGE('',*,*,#29848,.T.);
#42973=ORIENTED_EDGE('',*,*,#30076,.T.);
#42974=ORIENTED_EDGE('',*,*,#30477,.T.);
#42975=ORIENTED_EDGE('',*,*,#30364,.T.);
#42976=ORIENTED_EDGE('',*,*,#30245,.T.);
#42977=ORIENTED_EDGE('',*,*,#30368,.F.);
#42978=ORIENTED_EDGE('',*,*,#30476,.F.);
#42979=ORIENTED_EDGE('',*,*,#30072,.F.);
#42980=ORIENTED_EDGE('',*,*,#30366,.T.);
#42981=ORIENTED_EDGE('',*,*,#29498,.F.);
#42982=ORIENTED_EDGE('',*,*,#30083,.T.);
#42983=ORIENTED_EDGE('',*,*,#29565,.T.);
#42984=ORIENTED_EDGE('',*,*,#29567,.F.);
#42985=ORIENTED_EDGE('',*,*,#30082,.F.);
#42986=ORIENTED_EDGE('',*,*,#30478,.T.);
#42987=ORIENTED_EDGE('',*,*,#30372,.T.);
#42988=ORIENTED_EDGE('',*,*,#29496,.F.);
#42989=ORIENTED_EDGE('',*,*,#30370,.T.);
#42990=ORIENTED_EDGE('',*,*,#30479,.F.);
#42991=ORIENTED_EDGE('',*,*,#30084,.F.);
#42992=ORIENTED_EDGE('',*,*,#29844,.T.);
#42993=ORIENTED_EDGE('',*,*,#30085,.T.);
#42994=ORIENTED_EDGE('',*,*,#30479,.T.);
#42995=ORIENTED_EDGE('',*,*,#30369,.T.);
#42996=ORIENTED_EDGE('',*,*,#30243,.T.);
#42997=ORIENTED_EDGE('',*,*,#30373,.F.);
#42998=ORIENTED_EDGE('',*,*,#30478,.F.);
#42999=ORIENTED_EDGE('',*,*,#30081,.F.);
#43000=ORIENTED_EDGE('',*,*,#30371,.T.);
#43001=ORIENTED_EDGE('',*,*,#29494,.F.);
#43002=ORIENTED_EDGE('',*,*,#30092,.T.);
#43003=ORIENTED_EDGE('',*,*,#29569,.T.);
#43004=ORIENTED_EDGE('',*,*,#29571,.F.);
#43005=ORIENTED_EDGE('',*,*,#30091,.F.);
#43006=ORIENTED_EDGE('',*,*,#30480,.T.);
#43007=ORIENTED_EDGE('',*,*,#30377,.T.);
#43008=ORIENTED_EDGE('',*,*,#29492,.F.);
#43009=ORIENTED_EDGE('',*,*,#30375,.T.);
#43010=ORIENTED_EDGE('',*,*,#30481,.F.);
#43011=ORIENTED_EDGE('',*,*,#30093,.F.);
#43012=ORIENTED_EDGE('',*,*,#29840,.T.);
#43013=ORIENTED_EDGE('',*,*,#30094,.T.);
#43014=ORIENTED_EDGE('',*,*,#30481,.T.);
#43015=ORIENTED_EDGE('',*,*,#30374,.T.);
#43016=ORIENTED_EDGE('',*,*,#30241,.T.);
#43017=ORIENTED_EDGE('',*,*,#30378,.F.);
#43018=ORIENTED_EDGE('',*,*,#30480,.F.);
#43019=ORIENTED_EDGE('',*,*,#30090,.F.);
#43020=ORIENTED_EDGE('',*,*,#30376,.T.);
#43021=ORIENTED_EDGE('',*,*,#29490,.F.);
#43022=ORIENTED_EDGE('',*,*,#30101,.T.);
#43023=ORIENTED_EDGE('',*,*,#29573,.T.);
#43024=ORIENTED_EDGE('',*,*,#29575,.F.);
#43025=ORIENTED_EDGE('',*,*,#30100,.F.);
#43026=ORIENTED_EDGE('',*,*,#30482,.T.);
#43027=ORIENTED_EDGE('',*,*,#30382,.T.);
#43028=ORIENTED_EDGE('',*,*,#29488,.F.);
#43029=ORIENTED_EDGE('',*,*,#30380,.T.);
#43030=ORIENTED_EDGE('',*,*,#30483,.F.);
#43031=ORIENTED_EDGE('',*,*,#30102,.F.);
#43032=ORIENTED_EDGE('',*,*,#29836,.T.);
#43033=ORIENTED_EDGE('',*,*,#30103,.T.);
#43034=ORIENTED_EDGE('',*,*,#30483,.T.);
#43035=ORIENTED_EDGE('',*,*,#30379,.T.);
#43036=ORIENTED_EDGE('',*,*,#30239,.T.);
#43037=ORIENTED_EDGE('',*,*,#30383,.F.);
#43038=ORIENTED_EDGE('',*,*,#30482,.F.);
#43039=ORIENTED_EDGE('',*,*,#30099,.F.);
#43040=ORIENTED_EDGE('',*,*,#30381,.T.);
#43041=ORIENTED_EDGE('',*,*,#29486,.F.);
#43042=ORIENTED_EDGE('',*,*,#30110,.T.);
#43043=ORIENTED_EDGE('',*,*,#29577,.T.);
#43044=ORIENTED_EDGE('',*,*,#29579,.F.);
#43045=ORIENTED_EDGE('',*,*,#30109,.F.);
#43046=ORIENTED_EDGE('',*,*,#30484,.T.);
#43047=ORIENTED_EDGE('',*,*,#30386,.T.);
#43048=ORIENTED_EDGE('',*,*,#29484,.F.);
#43049=ORIENTED_EDGE('',*,*,#30385,.T.);
#43050=ORIENTED_EDGE('',*,*,#30485,.F.);
#43051=ORIENTED_EDGE('',*,*,#30111,.F.);
#43052=ORIENTED_EDGE('',*,*,#29832,.T.);
#43053=ORIENTED_EDGE('',*,*,#30112,.T.);
#43054=ORIENTED_EDGE('',*,*,#30485,.T.);
#43055=ORIENTED_EDGE('',*,*,#30384,.T.);
#43056=ORIENTED_EDGE('',*,*,#30237,.T.);
#43057=ORIENTED_EDGE('',*,*,#30387,.F.);
#43058=ORIENTED_EDGE('',*,*,#30484,.F.);
#43059=ORIENTED_EDGE('',*,*,#30108,.F.);
#43060=ORIENTED_EDGE('',*,*,#29632,.T.);
#43061=ORIENTED_EDGE('',*,*,#29683,.F.);
#43062=ORIENTED_EDGE('',*,*,#30119,.T.);
#43063=ORIENTED_EDGE('',*,*,#29731,.T.);
#43064=ORIENTED_EDGE('',*,*,#29733,.F.);
#43065=ORIENTED_EDGE('',*,*,#30118,.F.);
#43066=ORIENTED_EDGE('',*,*,#30486,.T.);
#43067=ORIENTED_EDGE('',*,*,#30391,.T.);
#43068=ORIENTED_EDGE('',*,*,#29681,.F.);
#43069=ORIENTED_EDGE('',*,*,#30389,.T.);
#43070=ORIENTED_EDGE('',*,*,#30487,.F.);
#43071=ORIENTED_EDGE('',*,*,#30120,.F.);
#43072=ORIENTED_EDGE('',*,*,#29828,.T.);
#43073=ORIENTED_EDGE('',*,*,#30121,.T.);
#43074=ORIENTED_EDGE('',*,*,#30487,.T.);
#43075=ORIENTED_EDGE('',*,*,#30388,.T.);
#43076=ORIENTED_EDGE('',*,*,#30235,.T.);
#43077=ORIENTED_EDGE('',*,*,#30392,.F.);
#43078=ORIENTED_EDGE('',*,*,#30486,.F.);
#43079=ORIENTED_EDGE('',*,*,#30117,.F.);
#43080=ORIENTED_EDGE('',*,*,#30390,.T.);
#43081=ORIENTED_EDGE('',*,*,#29679,.F.);
#43082=ORIENTED_EDGE('',*,*,#30128,.T.);
#43083=ORIENTED_EDGE('',*,*,#29735,.T.);
#43084=ORIENTED_EDGE('',*,*,#29737,.F.);
#43085=ORIENTED_EDGE('',*,*,#30127,.F.);
#43086=ORIENTED_EDGE('',*,*,#30488,.T.);
#43087=ORIENTED_EDGE('',*,*,#30396,.T.);
#43088=ORIENTED_EDGE('',*,*,#29677,.F.);
#43089=ORIENTED_EDGE('',*,*,#30394,.T.);
#43090=ORIENTED_EDGE('',*,*,#30489,.F.);
#43091=ORIENTED_EDGE('',*,*,#30129,.F.);
#43092=ORIENTED_EDGE('',*,*,#29824,.T.);
#43093=ORIENTED_EDGE('',*,*,#30130,.T.);
#43094=ORIENTED_EDGE('',*,*,#30489,.T.);
#43095=ORIENTED_EDGE('',*,*,#30393,.T.);
#43096=ORIENTED_EDGE('',*,*,#30233,.T.);
#43097=ORIENTED_EDGE('',*,*,#30397,.F.);
#43098=ORIENTED_EDGE('',*,*,#30488,.F.);
#43099=ORIENTED_EDGE('',*,*,#30126,.F.);
#43100=ORIENTED_EDGE('',*,*,#30395,.T.);
#43101=ORIENTED_EDGE('',*,*,#29675,.F.);
#43102=ORIENTED_EDGE('',*,*,#30137,.T.);
#43103=ORIENTED_EDGE('',*,*,#29739,.T.);
#43104=ORIENTED_EDGE('',*,*,#29741,.F.);
#43105=ORIENTED_EDGE('',*,*,#30136,.F.);
#43106=ORIENTED_EDGE('',*,*,#30490,.T.);
#43107=ORIENTED_EDGE('',*,*,#30401,.T.);
#43108=ORIENTED_EDGE('',*,*,#29673,.F.);
#43109=ORIENTED_EDGE('',*,*,#30399,.T.);
#43110=ORIENTED_EDGE('',*,*,#30491,.F.);
#43111=ORIENTED_EDGE('',*,*,#30138,.F.);
#43112=ORIENTED_EDGE('',*,*,#29820,.T.);
#43113=ORIENTED_EDGE('',*,*,#30139,.T.);
#43114=ORIENTED_EDGE('',*,*,#30491,.T.);
#43115=ORIENTED_EDGE('',*,*,#30398,.T.);
#43116=ORIENTED_EDGE('',*,*,#30231,.T.);
#43117=ORIENTED_EDGE('',*,*,#30402,.F.);
#43118=ORIENTED_EDGE('',*,*,#30490,.F.);
#43119=ORIENTED_EDGE('',*,*,#30135,.F.);
#43120=ORIENTED_EDGE('',*,*,#30400,.T.);
#43121=ORIENTED_EDGE('',*,*,#29671,.F.);
#43122=ORIENTED_EDGE('',*,*,#30146,.T.);
#43123=ORIENTED_EDGE('',*,*,#29743,.T.);
#43124=ORIENTED_EDGE('',*,*,#29745,.F.);
#43125=ORIENTED_EDGE('',*,*,#30145,.F.);
#43126=ORIENTED_EDGE('',*,*,#30492,.T.);
#43127=ORIENTED_EDGE('',*,*,#30406,.T.);
#43128=ORIENTED_EDGE('',*,*,#29669,.F.);
#43129=ORIENTED_EDGE('',*,*,#30404,.T.);
#43130=ORIENTED_EDGE('',*,*,#30493,.F.);
#43131=ORIENTED_EDGE('',*,*,#30147,.F.);
#43132=ORIENTED_EDGE('',*,*,#29816,.T.);
#43133=ORIENTED_EDGE('',*,*,#30148,.T.);
#43134=ORIENTED_EDGE('',*,*,#30493,.T.);
#43135=ORIENTED_EDGE('',*,*,#30403,.T.);
#43136=ORIENTED_EDGE('',*,*,#30229,.T.);
#43137=ORIENTED_EDGE('',*,*,#30407,.F.);
#43138=ORIENTED_EDGE('',*,*,#30492,.F.);
#43139=ORIENTED_EDGE('',*,*,#30144,.F.);
#43140=ORIENTED_EDGE('',*,*,#30405,.T.);
#43141=ORIENTED_EDGE('',*,*,#29667,.F.);
#43142=ORIENTED_EDGE('',*,*,#30155,.T.);
#43143=ORIENTED_EDGE('',*,*,#29747,.T.);
#43144=ORIENTED_EDGE('',*,*,#29749,.F.);
#43145=ORIENTED_EDGE('',*,*,#30154,.F.);
#43146=ORIENTED_EDGE('',*,*,#30494,.T.);
#43147=ORIENTED_EDGE('',*,*,#30411,.T.);
#43148=ORIENTED_EDGE('',*,*,#29665,.F.);
#43149=ORIENTED_EDGE('',*,*,#30409,.T.);
#43150=ORIENTED_EDGE('',*,*,#30495,.F.);
#43151=ORIENTED_EDGE('',*,*,#30156,.F.);
#43152=ORIENTED_EDGE('',*,*,#29812,.T.);
#43153=ORIENTED_EDGE('',*,*,#30157,.T.);
#43154=ORIENTED_EDGE('',*,*,#30495,.T.);
#43155=ORIENTED_EDGE('',*,*,#30408,.T.);
#43156=ORIENTED_EDGE('',*,*,#30227,.T.);
#43157=ORIENTED_EDGE('',*,*,#30412,.F.);
#43158=ORIENTED_EDGE('',*,*,#30494,.F.);
#43159=ORIENTED_EDGE('',*,*,#30153,.F.);
#43160=ORIENTED_EDGE('',*,*,#30410,.T.);
#43161=ORIENTED_EDGE('',*,*,#29663,.F.);
#43162=ORIENTED_EDGE('',*,*,#30164,.T.);
#43163=ORIENTED_EDGE('',*,*,#29751,.T.);
#43164=ORIENTED_EDGE('',*,*,#29753,.F.);
#43165=ORIENTED_EDGE('',*,*,#30163,.F.);
#43166=ORIENTED_EDGE('',*,*,#30496,.T.);
#43167=ORIENTED_EDGE('',*,*,#30416,.T.);
#43168=ORIENTED_EDGE('',*,*,#29661,.F.);
#43169=ORIENTED_EDGE('',*,*,#30414,.T.);
#43170=ORIENTED_EDGE('',*,*,#30497,.F.);
#43171=ORIENTED_EDGE('',*,*,#30165,.F.);
#43172=ORIENTED_EDGE('',*,*,#29808,.T.);
#43173=ORIENTED_EDGE('',*,*,#30166,.T.);
#43174=ORIENTED_EDGE('',*,*,#30497,.T.);
#43175=ORIENTED_EDGE('',*,*,#30413,.T.);
#43176=ORIENTED_EDGE('',*,*,#30225,.T.);
#43177=ORIENTED_EDGE('',*,*,#30417,.F.);
#43178=ORIENTED_EDGE('',*,*,#30496,.F.);
#43179=ORIENTED_EDGE('',*,*,#30162,.F.);
#43180=ORIENTED_EDGE('',*,*,#30415,.T.);
#43181=ORIENTED_EDGE('',*,*,#29659,.F.);
#43182=ORIENTED_EDGE('',*,*,#30173,.T.);
#43183=ORIENTED_EDGE('',*,*,#29755,.T.);
#43184=ORIENTED_EDGE('',*,*,#29757,.F.);
#43185=ORIENTED_EDGE('',*,*,#30172,.F.);
#43186=ORIENTED_EDGE('',*,*,#30498,.T.);
#43187=ORIENTED_EDGE('',*,*,#30421,.T.);
#43188=ORIENTED_EDGE('',*,*,#29657,.F.);
#43189=ORIENTED_EDGE('',*,*,#30419,.T.);
#43190=ORIENTED_EDGE('',*,*,#30499,.F.);
#43191=ORIENTED_EDGE('',*,*,#30174,.F.);
#43192=ORIENTED_EDGE('',*,*,#29804,.T.);
#43193=ORIENTED_EDGE('',*,*,#30175,.T.);
#43194=ORIENTED_EDGE('',*,*,#30499,.T.);
#43195=ORIENTED_EDGE('',*,*,#30418,.T.);
#43196=ORIENTED_EDGE('',*,*,#30223,.T.);
#43197=ORIENTED_EDGE('',*,*,#30422,.F.);
#43198=ORIENTED_EDGE('',*,*,#30498,.F.);
#43199=ORIENTED_EDGE('',*,*,#30171,.F.);
#43200=ORIENTED_EDGE('',*,*,#30420,.T.);
#43201=ORIENTED_EDGE('',*,*,#29655,.F.);
#43202=ORIENTED_EDGE('',*,*,#30182,.T.);
#43203=ORIENTED_EDGE('',*,*,#29759,.T.);
#43204=ORIENTED_EDGE('',*,*,#29761,.F.);
#43205=ORIENTED_EDGE('',*,*,#30181,.F.);
#43206=ORIENTED_EDGE('',*,*,#30500,.T.);
#43207=ORIENTED_EDGE('',*,*,#30426,.T.);
#43208=ORIENTED_EDGE('',*,*,#29653,.F.);
#43209=ORIENTED_EDGE('',*,*,#30424,.T.);
#43210=ORIENTED_EDGE('',*,*,#30501,.F.);
#43211=ORIENTED_EDGE('',*,*,#30183,.F.);
#43212=ORIENTED_EDGE('',*,*,#29800,.T.);
#43213=ORIENTED_EDGE('',*,*,#30184,.T.);
#43214=ORIENTED_EDGE('',*,*,#30501,.T.);
#43215=ORIENTED_EDGE('',*,*,#30423,.T.);
#43216=ORIENTED_EDGE('',*,*,#30221,.T.);
#43217=ORIENTED_EDGE('',*,*,#30427,.F.);
#43218=ORIENTED_EDGE('',*,*,#30500,.F.);
#43219=ORIENTED_EDGE('',*,*,#30180,.F.);
#43220=ORIENTED_EDGE('',*,*,#30425,.T.);
#43221=ORIENTED_EDGE('',*,*,#29651,.F.);
#43222=ORIENTED_EDGE('',*,*,#30191,.T.);
#43223=ORIENTED_EDGE('',*,*,#29763,.T.);
#43224=ORIENTED_EDGE('',*,*,#29765,.F.);
#43225=ORIENTED_EDGE('',*,*,#30190,.F.);
#43226=ORIENTED_EDGE('',*,*,#30502,.T.);
#43227=ORIENTED_EDGE('',*,*,#30431,.T.);
#43228=ORIENTED_EDGE('',*,*,#29649,.F.);
#43229=ORIENTED_EDGE('',*,*,#30429,.T.);
#43230=ORIENTED_EDGE('',*,*,#30503,.F.);
#43231=ORIENTED_EDGE('',*,*,#30192,.F.);
#43232=ORIENTED_EDGE('',*,*,#29796,.T.);
#43233=ORIENTED_EDGE('',*,*,#30193,.T.);
#43234=ORIENTED_EDGE('',*,*,#30503,.T.);
#43235=ORIENTED_EDGE('',*,*,#30428,.T.);
#43236=ORIENTED_EDGE('',*,*,#30219,.T.);
#43237=ORIENTED_EDGE('',*,*,#30432,.F.);
#43238=ORIENTED_EDGE('',*,*,#30502,.F.);
#43239=ORIENTED_EDGE('',*,*,#30189,.F.);
#43240=ORIENTED_EDGE('',*,*,#30430,.T.);
#43241=ORIENTED_EDGE('',*,*,#29647,.F.);
#43242=ORIENTED_EDGE('',*,*,#30200,.T.);
#43243=ORIENTED_EDGE('',*,*,#29767,.T.);
#43244=ORIENTED_EDGE('',*,*,#29769,.F.);
#43245=ORIENTED_EDGE('',*,*,#30199,.F.);
#43246=ORIENTED_EDGE('',*,*,#30504,.T.);
#43247=ORIENTED_EDGE('',*,*,#30436,.T.);
#43248=ORIENTED_EDGE('',*,*,#29645,.F.);
#43249=ORIENTED_EDGE('',*,*,#30434,.T.);
#43250=ORIENTED_EDGE('',*,*,#30505,.F.);
#43251=ORIENTED_EDGE('',*,*,#30201,.F.);
#43252=ORIENTED_EDGE('',*,*,#29792,.T.);
#43253=ORIENTED_EDGE('',*,*,#30202,.T.);
#43254=ORIENTED_EDGE('',*,*,#30505,.T.);
#43255=ORIENTED_EDGE('',*,*,#30433,.T.);
#43256=ORIENTED_EDGE('',*,*,#30217,.T.);
#43257=ORIENTED_EDGE('',*,*,#30437,.F.);
#43258=ORIENTED_EDGE('',*,*,#30504,.F.);
#43259=ORIENTED_EDGE('',*,*,#30198,.F.);
#43260=ORIENTED_EDGE('',*,*,#30435,.T.);
#43261=ORIENTED_EDGE('',*,*,#29643,.F.);
#43262=ORIENTED_EDGE('',*,*,#30209,.T.);
#43263=ORIENTED_EDGE('',*,*,#29771,.T.);
#43264=ORIENTED_EDGE('',*,*,#29773,.F.);
#43265=ORIENTED_EDGE('',*,*,#30208,.F.);
#43266=ORIENTED_EDGE('',*,*,#30506,.T.);
#43267=ORIENTED_EDGE('',*,*,#30440,.T.);
#43268=ORIENTED_EDGE('',*,*,#29641,.F.);
#43269=ORIENTED_EDGE('',*,*,#30439,.T.);
#43270=ORIENTED_EDGE('',*,*,#30507,.F.);
#43271=ORIENTED_EDGE('',*,*,#30210,.F.);
#43272=ORIENTED_EDGE('',*,*,#29788,.T.);
#43273=ORIENTED_EDGE('',*,*,#30211,.T.);
#43274=ORIENTED_EDGE('',*,*,#30507,.T.);
#43275=ORIENTED_EDGE('',*,*,#30438,.T.);
#43276=ORIENTED_EDGE('',*,*,#30215,.T.);
#43277=ORIENTED_EDGE('',*,*,#30441,.F.);
#43278=ORIENTED_EDGE('',*,*,#30506,.F.);
#43279=ORIENTED_EDGE('',*,*,#30207,.F.);
#43280=ORIENTED_EDGE('',*,*,#30508,.T.);
#43281=ORIENTED_EDGE('',*,*,#30509,.T.);
#43282=ORIENTED_EDGE('',*,*,#30510,.T.);
#43283=ORIENTED_EDGE('',*,*,#30509,.F.);
#43284=ORIENTED_EDGE('',*,*,#30511,.T.);
#43285=ORIENTED_EDGE('',*,*,#30510,.F.);
#43286=ORIENTED_EDGE('',*,*,#30512,.F.);
#43287=ORIENTED_EDGE('',*,*,#30513,.T.);
#43288=ORIENTED_EDGE('',*,*,#30514,.T.);
#43289=ORIENTED_EDGE('',*,*,#30511,.F.);
#43290=ORIENTED_EDGE('',*,*,#30508,.F.);
#43291=ORIENTED_EDGE('',*,*,#30514,.F.);
#43292=ORIENTED_EDGE('',*,*,#30515,.T.);
#43293=ORIENTED_EDGE('',*,*,#30516,.T.);
#43294=ORIENTED_EDGE('',*,*,#30517,.T.);
#43295=ORIENTED_EDGE('',*,*,#30518,.T.);
#43296=ORIENTED_EDGE('',*,*,#30516,.F.);
#43297=ORIENTED_EDGE('',*,*,#30515,.F.);
#43298=ORIENTED_EDGE('',*,*,#30519,.F.);
#43299=ORIENTED_EDGE('',*,*,#30517,.F.);
#43300=ORIENTED_EDGE('',*,*,#30518,.F.);
#43301=ORIENTED_EDGE('',*,*,#30520,.T.);
#43302=ORIENTED_EDGE('',*,*,#29536,.F.);
#43303=ORIENTED_EDGE('',*,*,#30520,.F.);
#43304=ORIENTED_EDGE('',*,*,#30512,.T.);
#43305=ORIENTED_EDGE('',*,*,#30521,.T.);
#43306=ORIENTED_EDGE('',*,*,#30522,.T.);
#43307=ORIENTED_EDGE('',*,*,#30523,.T.);
#43308=ORIENTED_EDGE('',*,*,#30521,.F.);
#43309=ORIENTED_EDGE('',*,*,#30524,.F.);
#43310=ORIENTED_EDGE('',*,*,#30525,.T.);
#43311=ORIENTED_EDGE('',*,*,#30522,.F.);
#43312=ORIENTED_EDGE('',*,*,#30523,.F.);
#43313=ORIENTED_EDGE('',*,*,#30525,.F.);
#43314=ORIENTED_EDGE('',*,*,#30526,.T.);
#43315=ORIENTED_EDGE('',*,*,#30527,.T.);
#43316=ORIENTED_EDGE('',*,*,#30519,.T.);
#43317=ORIENTED_EDGE('',*,*,#30527,.F.);
#43318=ORIENTED_EDGE('',*,*,#30528,.T.);
#43319=ORIENTED_EDGE('',*,*,#30526,.F.);
#43320=ORIENTED_EDGE('',*,*,#30529,.T.);
#43321=ORIENTED_EDGE('',*,*,#30530,.T.);
#43322=ORIENTED_EDGE('',*,*,#30529,.F.);
#43323=ORIENTED_EDGE('',*,*,#30528,.F.);
#43324=ORIENTED_EDGE('',*,*,#30531,.T.);
#43325=ORIENTED_EDGE('',*,*,#30532,.T.);
#43326=ORIENTED_EDGE('',*,*,#30533,.F.);
#43327=ORIENTED_EDGE('',*,*,#30532,.F.);
#43328=ORIENTED_EDGE('',*,*,#30533,.T.);
#43329=ORIENTED_EDGE('',*,*,#30534,.T.);
#43330=ORIENTED_EDGE('',*,*,#30535,.F.);
#43331=ORIENTED_EDGE('',*,*,#30534,.F.);
#43332=ORIENTED_EDGE('',*,*,#30530,.F.);
#43333=ORIENTED_EDGE('',*,*,#30535,.T.);
#43334=ORIENTED_EDGE('',*,*,#29464,.T.);
#43335=ORIENTED_EDGE('',*,*,#29729,.T.);
#43336=ORIENTED_EDGE('',*,*,#29782,.T.);
#43337=ORIENTED_EDGE('',*,*,#29783,.T.);
#43338=ORIENTED_EDGE('',*,*,#29777,.T.);
#43339=ORIENTED_EDGE('',*,*,#29637,.T.);
#43340=ORIENTED_EDGE('',*,*,#29635,.T.);
#43341=ORIENTED_EDGE('',*,*,#29636,.T.);
#43342=ORIENTED_EDGE('',*,*,#29628,.T.);
#43343=ORIENTED_EDGE('',*,*,#29480,.T.);
#43344=ORIENTED_EDGE('',*,*,#29474,.T.);
#43345=ORIENTED_EDGE('',*,*,#29476,.T.);
#43346=ORIENTED_EDGE('',*,*,#30513,.F.);
#43347=ORIENTED_EDGE('',*,*,#30524,.T.);
#43348=ORIENTED_EDGE('',*,*,#30536,.F.);
#43349=ORIENTED_EDGE('',*,*,#30536,.T.);
#43350=ORIENTED_EDGE('',*,*,#30537,.T.);
#43351=ORIENTED_EDGE('',*,*,#30531,.F.);
#43352=ORIENTED_EDGE('',*,*,#30537,.F.);
#48194=CONICAL_SURFACE('',#53615,37.55,0.785398163397448);
#48195=CONICAL_SURFACE('',#53634,37.55,0.785398163397451);
#48196=CONICAL_SURFACE('',#53647,37.55,0.785398163397451);
#48197=CONICAL_SURFACE('',#53662,37.55,0.785398163397448);
#48198=CONICAL_SURFACE('',#53676,37.55,0.785398163397448);
#48199=CONICAL_SURFACE('',#53690,37.55,0.785398163397451);
#48200=CONICAL_SURFACE('',#53707,41.85,0.750929062397939);
#48201=CONICAL_SURFACE('',#53709,41.85,0.750929062397939);
#48202=CONICAL_SURFACE('',#53711,41.85,0.750929062397939);
#48203=CONICAL_SURFACE('',#53713,41.85,0.750929062397939);
#48204=CONICAL_SURFACE('',#53715,41.85,0.750929062397939);
#48205=CONICAL_SURFACE('',#53717,41.85,0.750929062397939);
#48206=CONICAL_SURFACE('',#53719,41.85,0.750929062397939);
#48207=CONICAL_SURFACE('',#53721,41.85,0.750929062397939);
#48208=CONICAL_SURFACE('',#53723,41.85,0.750929062397939);
#48209=CONICAL_SURFACE('',#53725,41.85,0.750929062397939);
#48210=CONICAL_SURFACE('',#53727,41.85,0.750929062397939);
#48211=CONICAL_SURFACE('',#53729,41.85,0.750929062397939);
#48212=CONICAL_SURFACE('',#53731,41.85,0.750929062397939);
#48213=CONICAL_SURFACE('',#53733,41.85,0.750929062397939);
#48214=CONICAL_SURFACE('',#53735,41.85,0.750929062397939);
#48215=CONICAL_SURFACE('',#53737,41.85,0.750929062397939);
#48216=CONICAL_SURFACE('',#53739,41.85,0.750929062397939);
#48217=CONICAL_SURFACE('',#53741,41.85,0.750929062397939);
#48218=CONICAL_SURFACE('',#53743,41.85,0.750929062397939);
#48219=CONICAL_SURFACE('',#53745,41.85,0.750929062397939);
#48220=CONICAL_SURFACE('',#53747,41.85,0.750929062397939);
#48221=CONICAL_SURFACE('',#53749,41.85,0.750929062397939);
#48222=CONICAL_SURFACE('',#53751,41.85,0.750929062397939);
#48223=CONICAL_SURFACE('',#53753,41.85,0.750929062397939);
#48224=CONICAL_SURFACE('',#53755,41.85,0.750929062397939);
#48225=CONICAL_SURFACE('',#53757,41.85,0.750929062397939);
#48226=CONICAL_SURFACE('',#53759,41.85,0.750929062397939);
#48227=CONICAL_SURFACE('',#53761,41.85,0.750929062397939);
#48228=CONICAL_SURFACE('',#53763,41.85,0.750929062397939);
#48229=CONICAL_SURFACE('',#53765,41.85,0.750929062397939);
#48230=CONICAL_SURFACE('',#53767,41.85,0.750929062397939);
#48231=CONICAL_SURFACE('',#53769,41.85,0.750929062397939);
#48232=CONICAL_SURFACE('',#53771,41.85,0.750929062397939);
#48233=CONICAL_SURFACE('',#53839,41.85,0.750929062397939);
#48234=CONICAL_SURFACE('',#53841,41.85,0.750929062397939);
#48235=CONICAL_SURFACE('',#53843,41.85,0.750929062397939);
#48236=CONICAL_SURFACE('',#53845,41.85,0.750929062397939);
#48237=CONICAL_SURFACE('',#53847,41.85,0.750929062397939);
#48238=CONICAL_SURFACE('',#53849,41.85,0.750929062397939);
#48239=CONICAL_SURFACE('',#53851,41.85,0.750929062397939);
#48240=CONICAL_SURFACE('',#53853,41.85,0.750929062397939);
#48241=CONICAL_SURFACE('',#53855,41.85,0.750929062397939);
#48242=CONICAL_SURFACE('',#53857,41.85,0.750929062397939);
#48243=CONICAL_SURFACE('',#53859,41.85,0.750929062397939);
#48244=CONICAL_SURFACE('',#53861,41.85,0.750929062397939);
#48245=CONICAL_SURFACE('',#53863,41.85,0.750929062397939);
#48246=CONICAL_SURFACE('',#53865,41.85,0.750929062397939);
#48247=CONICAL_SURFACE('',#53867,41.85,0.750929062397939);
#48248=CONICAL_SURFACE('',#53869,41.85,0.750929062397939);
#48249=CONICAL_SURFACE('',#53871,41.85,0.750929062397939);
#48250=CONICAL_SURFACE('',#53873,41.85,0.750929062397939);
#48251=CONICAL_SURFACE('',#53875,41.85,0.750929062397939);
#48252=CONICAL_SURFACE('',#53877,41.85,0.750929062397939);
#48253=CONICAL_SURFACE('',#53879,41.85,0.750929062397939);
#48254=CONICAL_SURFACE('',#53881,41.85,0.750929062397939);
#48255=CONICAL_SURFACE('',#53883,41.85,0.750929062397939);
#48256=CONICAL_SURFACE('',#53885,41.85,0.750929062397939);
#48257=CONICAL_SURFACE('',#53887,41.85,0.750929062397939);
#48258=CONICAL_SURFACE('',#53889,41.85,0.750929062397939);
#48259=CONICAL_SURFACE('',#53891,41.85,0.750929062397939);
#48260=CONICAL_SURFACE('',#53893,41.85,0.750929062397939);
#48261=CONICAL_SURFACE('',#53895,41.85,0.750929062397939);
#48262=CONICAL_SURFACE('',#53897,41.85,0.750929062397939);
#48263=CONICAL_SURFACE('',#53899,41.85,0.750929062397939);
#48264=CONICAL_SURFACE('',#53901,41.85,0.750929062397939);
#48265=CONICAL_SURFACE('',#53903,41.85,0.750929062397939);
#48266=CONICAL_SURFACE('',#54135,15.41,0.785398163397449);
#48267=CONICAL_SURFACE('',#54141,15.41,0.785398163397448);
#49722=ADVANCED_FACE('',(#14635),#12480,.F.);
#49723=ADVANCED_FACE('',(#14636),#12481,.F.);
#49724=ADVANCED_FACE('',(#14637),#12482,.F.);
#49725=ADVANCED_FACE('',(#14638),#1084,.T.);
#49726=ADVANCED_FACE('',(#14639),#48194,.T.);
#49727=ADVANCED_FACE('',(#14640,#963),#12483,.T.);
#49728=ADVANCED_FACE('',(#14641),#48195,.T.);
#49729=ADVANCED_FACE('',(#14642),#48196,.T.);
#49730=ADVANCED_FACE('',(#14643),#12484,.F.);
#49731=ADVANCED_FACE('',(#14644),#12485,.F.);
#49732=ADVANCED_FACE('',(#14645),#12486,.F.);
#49733=ADVANCED_FACE('',(#14646),#48197,.T.);
#49734=ADVANCED_FACE('',(#14647),#48198,.T.);
#49735=ADVANCED_FACE('',(#14648),#1085,.T.);
#49736=ADVANCED_FACE('',(#14649),#48199,.T.);
#49737=ADVANCED_FACE('',(#14650),#12487,.F.);
#49738=ADVANCED_FACE('',(#14651),#12488,.F.);
#49739=ADVANCED_FACE('',(#14652),#12489,.F.);
#49740=ADVANCED_FACE('',(#14653),#1086,.T.);
#49741=ADVANCED_FACE('',(#14654),#48200,.T.);
#49742=ADVANCED_FACE('',(#14655),#48201,.T.);
#49743=ADVANCED_FACE('',(#14656),#48202,.T.);
#49744=ADVANCED_FACE('',(#14657),#48203,.T.);
#49745=ADVANCED_FACE('',(#14658),#48204,.T.);
#49746=ADVANCED_FACE('',(#14659),#48205,.T.);
#49747=ADVANCED_FACE('',(#14660),#48206,.T.);
#49748=ADVANCED_FACE('',(#14661),#48207,.T.);
#49749=ADVANCED_FACE('',(#14662),#48208,.T.);
#49750=ADVANCED_FACE('',(#14663),#48209,.T.);
#49751=ADVANCED_FACE('',(#14664),#48210,.T.);
#49752=ADVANCED_FACE('',(#14665),#48211,.T.);
#49753=ADVANCED_FACE('',(#14666),#48212,.T.);
#49754=ADVANCED_FACE('',(#14667),#48213,.T.);
#49755=ADVANCED_FACE('',(#14668),#48214,.T.);
#49756=ADVANCED_FACE('',(#14669),#48215,.T.);
#49757=ADVANCED_FACE('',(#14670),#48216,.T.);
#49758=ADVANCED_FACE('',(#14671),#48217,.T.);
#49759=ADVANCED_FACE('',(#14672),#48218,.T.);
#49760=ADVANCED_FACE('',(#14673),#48219,.T.);
#49761=ADVANCED_FACE('',(#14674),#48220,.T.);
#49762=ADVANCED_FACE('',(#14675),#48221,.T.);
#49763=ADVANCED_FACE('',(#14676),#48222,.T.);
#49764=ADVANCED_FACE('',(#14677),#48223,.T.);
#49765=ADVANCED_FACE('',(#14678),#48224,.T.);
#49766=ADVANCED_FACE('',(#14679),#48225,.T.);
#49767=ADVANCED_FACE('',(#14680),#48226,.T.);
#49768=ADVANCED_FACE('',(#14681),#48227,.T.);
#49769=ADVANCED_FACE('',(#14682),#48228,.T.);
#49770=ADVANCED_FACE('',(#14683),#48229,.T.);
#49771=ADVANCED_FACE('',(#14684),#48230,.T.);
#49772=ADVANCED_FACE('',(#14685),#48231,.T.);
#49773=ADVANCED_FACE('',(#14686),#48232,.T.);
#49774=ADVANCED_FACE('',(#14687),#12490,.T.);
#49775=ADVANCED_FACE('',(#14688),#12491,.T.);
#49776=ADVANCED_FACE('',(#14689),#12492,.T.);
#49777=ADVANCED_FACE('',(#14690),#12493,.T.);
#49778=ADVANCED_FACE('',(#14691),#12494,.T.);
#49779=ADVANCED_FACE('',(#14692),#12495,.T.);
#49780=ADVANCED_FACE('',(#14693),#12496,.T.);
#49781=ADVANCED_FACE('',(#14694),#12497,.T.);
#49782=ADVANCED_FACE('',(#14695),#12498,.T.);
#49783=ADVANCED_FACE('',(#14696),#12499,.T.);
#49784=ADVANCED_FACE('',(#14697),#12500,.T.);
#49785=ADVANCED_FACE('',(#14698),#12501,.T.);
#49786=ADVANCED_FACE('',(#14699),#12502,.T.);
#49787=ADVANCED_FACE('',(#14700),#12503,.T.);
#49788=ADVANCED_FACE('',(#14701),#12504,.T.);
#49789=ADVANCED_FACE('',(#14702),#12505,.T.);
#49790=ADVANCED_FACE('',(#14703),#12506,.T.);
#49791=ADVANCED_FACE('',(#14704),#12507,.T.);
#49792=ADVANCED_FACE('',(#14705),#12508,.T.);
#49793=ADVANCED_FACE('',(#14706),#12509,.T.);
#49794=ADVANCED_FACE('',(#14707),#12510,.T.);
#49795=ADVANCED_FACE('',(#14708),#12511,.T.);
#49796=ADVANCED_FACE('',(#14709),#12512,.T.);
#49797=ADVANCED_FACE('',(#14710),#12513,.T.);
#49798=ADVANCED_FACE('',(#14711),#12514,.T.);
#49799=ADVANCED_FACE('',(#14712),#12515,.T.);
#49800=ADVANCED_FACE('',(#14713),#12516,.T.);
#49801=ADVANCED_FACE('',(#14714),#12517,.T.);
#49802=ADVANCED_FACE('',(#14715),#12518,.T.);
#49803=ADVANCED_FACE('',(#14716),#12519,.T.);
#49804=ADVANCED_FACE('',(#14717),#12520,.T.);
#49805=ADVANCED_FACE('',(#14718),#12521,.T.);
#49806=ADVANCED_FACE('',(#14719),#12522,.T.);
#49807=ADVANCED_FACE('',(#14720),#12523,.T.);
#49808=ADVANCED_FACE('',(#14721),#12524,.T.);
#49809=ADVANCED_FACE('',(#14722),#12525,.T.);
#49810=ADVANCED_FACE('',(#14723),#12526,.T.);
#49811=ADVANCED_FACE('',(#14724),#12527,.T.);
#49812=ADVANCED_FACE('',(#14725),#12528,.T.);
#49813=ADVANCED_FACE('',(#14726),#12529,.T.);
#49814=ADVANCED_FACE('',(#14727),#12530,.T.);
#49815=ADVANCED_FACE('',(#14728),#12531,.T.);
#49816=ADVANCED_FACE('',(#14729),#12532,.T.);
#49817=ADVANCED_FACE('',(#14730),#12533,.T.);
#49818=ADVANCED_FACE('',(#14731),#12534,.T.);
#49819=ADVANCED_FACE('',(#14732),#12535,.T.);
#49820=ADVANCED_FACE('',(#14733),#12536,.T.);
#49821=ADVANCED_FACE('',(#14734),#12537,.T.);
#49822=ADVANCED_FACE('',(#14735),#12538,.T.);
#49823=ADVANCED_FACE('',(#14736),#12539,.T.);
#49824=ADVANCED_FACE('',(#14737),#12540,.T.);
#49825=ADVANCED_FACE('',(#14738),#12541,.T.);
#49826=ADVANCED_FACE('',(#14739),#12542,.T.);
#49827=ADVANCED_FACE('',(#14740),#12543,.T.);
#49828=ADVANCED_FACE('',(#14741),#12544,.T.);
#49829=ADVANCED_FACE('',(#14742),#12545,.T.);
#49830=ADVANCED_FACE('',(#14743),#12546,.T.);
#49831=ADVANCED_FACE('',(#14744),#12547,.T.);
#49832=ADVANCED_FACE('',(#14745),#12548,.T.);
#49833=ADVANCED_FACE('',(#14746),#12549,.T.);
#49834=ADVANCED_FACE('',(#14747),#12550,.T.);
#49835=ADVANCED_FACE('',(#14748),#12551,.T.);
#49836=ADVANCED_FACE('',(#14749),#12552,.T.);
#49837=ADVANCED_FACE('',(#14750),#12553,.T.);
#49838=ADVANCED_FACE('',(#14751),#12554,.T.);
#49839=ADVANCED_FACE('',(#14752),#12555,.T.);
#49840=ADVANCED_FACE('',(#14753),#48233,.T.);
#49841=ADVANCED_FACE('',(#14754),#48234,.T.);
#49842=ADVANCED_FACE('',(#14755),#48235,.T.);
#49843=ADVANCED_FACE('',(#14756),#48236,.T.);
#49844=ADVANCED_FACE('',(#14757),#48237,.T.);
#49845=ADVANCED_FACE('',(#14758),#48238,.T.);
#49846=ADVANCED_FACE('',(#14759),#48239,.T.);
#49847=ADVANCED_FACE('',(#14760),#48240,.T.);
#49848=ADVANCED_FACE('',(#14761),#48241,.T.);
#49849=ADVANCED_FACE('',(#14762),#48242,.T.);
#49850=ADVANCED_FACE('',(#14763),#48243,.T.);
#49851=ADVANCED_FACE('',(#14764),#48244,.T.);
#49852=ADVANCED_FACE('',(#14765),#48245,.T.);
#49853=ADVANCED_FACE('',(#14766),#48246,.T.);
#49854=ADVANCED_FACE('',(#14767),#48247,.T.);
#49855=ADVANCED_FACE('',(#14768),#48248,.T.);
#49856=ADVANCED_FACE('',(#14769),#48249,.T.);
#49857=ADVANCED_FACE('',(#14770),#48250,.T.);
#49858=ADVANCED_FACE('',(#14771),#48251,.T.);
#49859=ADVANCED_FACE('',(#14772),#48252,.T.);
#49860=ADVANCED_FACE('',(#14773),#48253,.T.);
#49861=ADVANCED_FACE('',(#14774),#48254,.T.);
#49862=ADVANCED_FACE('',(#14775),#48255,.T.);
#49863=ADVANCED_FACE('',(#14776),#48256,.T.);
#49864=ADVANCED_FACE('',(#14777),#48257,.T.);
#49865=ADVANCED_FACE('',(#14778),#48258,.T.);
#49866=ADVANCED_FACE('',(#14779),#48259,.T.);
#49867=ADVANCED_FACE('',(#14780),#48260,.T.);
#49868=ADVANCED_FACE('',(#14781),#48261,.T.);
#49869=ADVANCED_FACE('',(#14782),#48262,.T.);
#49870=ADVANCED_FACE('',(#14783),#48263,.T.);
#49871=ADVANCED_FACE('',(#14784),#48264,.T.);
#49872=ADVANCED_FACE('',(#14785),#48265,.T.);
#49873=ADVANCED_FACE('',(#14786),#12556,.T.);
#49874=ADVANCED_FACE('',(#14787),#12557,.T.);
#49875=ADVANCED_FACE('',(#14788),#12558,.T.);
#49876=ADVANCED_FACE('',(#14789),#12559,.T.);
#49877=ADVANCED_FACE('',(#14790),#12560,.T.);
#49878=ADVANCED_FACE('',(#14791),#12561,.T.);
#49879=ADVANCED_FACE('',(#14792),#12562,.T.);
#49880=ADVANCED_FACE('',(#14793),#12563,.T.);
#49881=ADVANCED_FACE('',(#14794),#12564,.T.);
#49882=ADVANCED_FACE('',(#14795),#12565,.T.);
#49883=ADVANCED_FACE('',(#14796),#12566,.T.);
#49884=ADVANCED_FACE('',(#14797),#12567,.T.);
#49885=ADVANCED_FACE('',(#14798),#12568,.T.);
#49886=ADVANCED_FACE('',(#14799),#12569,.T.);
#49887=ADVANCED_FACE('',(#14800),#12570,.T.);
#49888=ADVANCED_FACE('',(#14801),#12571,.T.);
#49889=ADVANCED_FACE('',(#14802),#12572,.T.);
#49890=ADVANCED_FACE('',(#14803),#12573,.T.);
#49891=ADVANCED_FACE('',(#14804),#12574,.T.);
#49892=ADVANCED_FACE('',(#14805),#12575,.T.);
#49893=ADVANCED_FACE('',(#14806),#12576,.T.);
#49894=ADVANCED_FACE('',(#14807),#12577,.T.);
#49895=ADVANCED_FACE('',(#14808),#12578,.T.);
#49896=ADVANCED_FACE('',(#14809),#12579,.T.);
#49897=ADVANCED_FACE('',(#14810),#12580,.T.);
#49898=ADVANCED_FACE('',(#14811),#12581,.T.);
#49899=ADVANCED_FACE('',(#14812),#12582,.T.);
#49900=ADVANCED_FACE('',(#14813),#12583,.T.);
#49901=ADVANCED_FACE('',(#14814),#12584,.T.);
#49902=ADVANCED_FACE('',(#14815),#12585,.T.);
#49903=ADVANCED_FACE('',(#14816),#12586,.T.);
#49904=ADVANCED_FACE('',(#14817),#12587,.T.);
#49905=ADVANCED_FACE('',(#14818),#12588,.T.);
#49906=ADVANCED_FACE('',(#14819),#12589,.T.);
#49907=ADVANCED_FACE('',(#14820),#12590,.T.);
#49908=ADVANCED_FACE('',(#14821),#12591,.T.);
#49909=ADVANCED_FACE('',(#14822),#12592,.F.);
#49910=ADVANCED_FACE('',(#14823),#1087,.T.);
#49911=ADVANCED_FACE('',(#14824),#1088,.T.);
#49912=ADVANCED_FACE('',(#14825),#12593,.T.);
#49913=ADVANCED_FACE('',(#14826),#12594,.T.);
#49914=ADVANCED_FACE('',(#14827),#12595,.T.);
#49915=ADVANCED_FACE('',(#14828),#12596,.F.);
#49916=ADVANCED_FACE('',(#14829),#1089,.T.);
#49917=ADVANCED_FACE('',(#14830),#12597,.T.);
#49918=ADVANCED_FACE('',(#14831),#12598,.T.);
#49919=ADVANCED_FACE('',(#14832),#12599,.T.);
#49920=ADVANCED_FACE('',(#14833),#12600,.F.);
#49921=ADVANCED_FACE('',(#14834),#1090,.T.);
#49922=ADVANCED_FACE('',(#14835),#12601,.T.);
#49923=ADVANCED_FACE('',(#14836),#12602,.T.);
#49924=ADVANCED_FACE('',(#14837),#12603,.T.);
#49925=ADVANCED_FACE('',(#14838),#12604,.F.);
#49926=ADVANCED_FACE('',(#14839),#1091,.T.);
#49927=ADVANCED_FACE('',(#14840),#12605,.T.);
#49928=ADVANCED_FACE('',(#14841),#12606,.T.);
#49929=ADVANCED_FACE('',(#14842),#12607,.T.);
#49930=ADVANCED_FACE('',(#14843),#12608,.F.);
#49931=ADVANCED_FACE('',(#14844),#1092,.T.);
#49932=ADVANCED_FACE('',(#14845),#12609,.T.);
#49933=ADVANCED_FACE('',(#14846),#12610,.T.);
#49934=ADVANCED_FACE('',(#14847),#12611,.T.);
#49935=ADVANCED_FACE('',(#14848),#12612,.F.);
#49936=ADVANCED_FACE('',(#14849),#1093,.T.);
#49937=ADVANCED_FACE('',(#14850),#12613,.T.);
#49938=ADVANCED_FACE('',(#14851),#12614,.T.);
#49939=ADVANCED_FACE('',(#14852),#12615,.T.);
#49940=ADVANCED_FACE('',(#14853),#12616,.F.);
#49941=ADVANCED_FACE('',(#14854),#1094,.T.);
#49942=ADVANCED_FACE('',(#14855),#12617,.T.);
#49943=ADVANCED_FACE('',(#14856),#12618,.T.);
#49944=ADVANCED_FACE('',(#14857),#12619,.T.);
#49945=ADVANCED_FACE('',(#14858),#12620,.F.);
#49946=ADVANCED_FACE('',(#14859),#1095,.T.);
#49947=ADVANCED_FACE('',(#14860),#12621,.T.);
#49948=ADVANCED_FACE('',(#14861),#12622,.T.);
#49949=ADVANCED_FACE('',(#14862),#12623,.T.);
#49950=ADVANCED_FACE('',(#14863),#12624,.F.);
#49951=ADVANCED_FACE('',(#14864),#1096,.T.);
#49952=ADVANCED_FACE('',(#14865),#12625,.T.);
#49953=ADVANCED_FACE('',(#14866),#12626,.T.);
#49954=ADVANCED_FACE('',(#14867),#12627,.T.);
#49955=ADVANCED_FACE('',(#14868),#12628,.F.);
#49956=ADVANCED_FACE('',(#14869),#1097,.T.);
#49957=ADVANCED_FACE('',(#14870),#12629,.T.);
#49958=ADVANCED_FACE('',(#14871),#12630,.T.);
#49959=ADVANCED_FACE('',(#14872),#12631,.T.);
#49960=ADVANCED_FACE('',(#14873),#12632,.F.);
#49961=ADVANCED_FACE('',(#14874),#1098,.T.);
#49962=ADVANCED_FACE('',(#14875),#12633,.T.);
#49963=ADVANCED_FACE('',(#14876),#12634,.T.);
#49964=ADVANCED_FACE('',(#14877),#12635,.T.);
#49965=ADVANCED_FACE('',(#14878),#12636,.F.);
#49966=ADVANCED_FACE('',(#14879),#1099,.T.);
#49967=ADVANCED_FACE('',(#14880),#12637,.T.);
#49968=ADVANCED_FACE('',(#14881),#12638,.T.);
#49969=ADVANCED_FACE('',(#14882),#12639,.T.);
#49970=ADVANCED_FACE('',(#14883),#12640,.F.);
#49971=ADVANCED_FACE('',(#14884),#1100,.T.);
#49972=ADVANCED_FACE('',(#14885),#12641,.T.);
#49973=ADVANCED_FACE('',(#14886),#12642,.T.);
#49974=ADVANCED_FACE('',(#14887),#12643,.T.);
#49975=ADVANCED_FACE('',(#14888),#12644,.F.);
#49976=ADVANCED_FACE('',(#14889),#1101,.T.);
#49977=ADVANCED_FACE('',(#14890),#12645,.T.);
#49978=ADVANCED_FACE('',(#14891),#12646,.T.);
#49979=ADVANCED_FACE('',(#14892),#12647,.T.);
#49980=ADVANCED_FACE('',(#14893),#12648,.F.);
#49981=ADVANCED_FACE('',(#14894),#1102,.T.);
#49982=ADVANCED_FACE('',(#14895),#12649,.T.);
#49983=ADVANCED_FACE('',(#14896),#12650,.T.);
#49984=ADVANCED_FACE('',(#14897),#12651,.T.);
#49985=ADVANCED_FACE('',(#14898),#12652,.F.);
#49986=ADVANCED_FACE('',(#14899),#1103,.T.);
#49987=ADVANCED_FACE('',(#14900),#12653,.T.);
#49988=ADVANCED_FACE('',(#14901),#12654,.T.);
#49989=ADVANCED_FACE('',(#14902),#12655,.T.);
#49990=ADVANCED_FACE('',(#14903),#12656,.F.);
#49991=ADVANCED_FACE('',(#14904),#1104,.T.);
#49992=ADVANCED_FACE('',(#14905),#12657,.T.);
#49993=ADVANCED_FACE('',(#14906),#12658,.T.);
#49994=ADVANCED_FACE('',(#14907),#12659,.T.);
#49995=ADVANCED_FACE('',(#14908),#12660,.F.);
#49996=ADVANCED_FACE('',(#14909),#1105,.T.);
#49997=ADVANCED_FACE('',(#14910),#12661,.T.);
#49998=ADVANCED_FACE('',(#14911),#12662,.T.);
#49999=ADVANCED_FACE('',(#14912),#12663,.T.);
#50000=ADVANCED_FACE('',(#14913),#12664,.F.);
#50001=ADVANCED_FACE('',(#14914),#1106,.T.);
#50002=ADVANCED_FACE('',(#14915),#12665,.T.);
#50003=ADVANCED_FACE('',(#14916),#12666,.T.);
#50004=ADVANCED_FACE('',(#14917),#12667,.T.);
#50005=ADVANCED_FACE('',(#14918),#12668,.F.);
#50006=ADVANCED_FACE('',(#14919),#1107,.T.);
#50007=ADVANCED_FACE('',(#14920),#12669,.T.);
#50008=ADVANCED_FACE('',(#14921),#12670,.T.);
#50009=ADVANCED_FACE('',(#14922),#12671,.T.);
#50010=ADVANCED_FACE('',(#14923),#12672,.F.);
#50011=ADVANCED_FACE('',(#14924),#1108,.T.);
#50012=ADVANCED_FACE('',(#14925),#12673,.T.);
#50013=ADVANCED_FACE('',(#14926),#12674,.T.);
#50014=ADVANCED_FACE('',(#14927),#12675,.T.);
#50015=ADVANCED_FACE('',(#14928),#12676,.F.);
#50016=ADVANCED_FACE('',(#14929),#1109,.T.);
#50017=ADVANCED_FACE('',(#14930),#12677,.T.);
#50018=ADVANCED_FACE('',(#14931),#12678,.T.);
#50019=ADVANCED_FACE('',(#14932),#12679,.T.);
#50020=ADVANCED_FACE('',(#14933),#12680,.F.);
#50021=ADVANCED_FACE('',(#14934),#1110,.T.);
#50022=ADVANCED_FACE('',(#14935),#12681,.T.);
#50023=ADVANCED_FACE('',(#14936),#12682,.T.);
#50024=ADVANCED_FACE('',(#14937),#12683,.T.);
#50025=ADVANCED_FACE('',(#14938),#12684,.F.);
#50026=ADVANCED_FACE('',(#14939),#1111,.T.);
#50027=ADVANCED_FACE('',(#14940),#12685,.T.);
#50028=ADVANCED_FACE('',(#14941),#12686,.T.);
#50029=ADVANCED_FACE('',(#14942),#12687,.T.);
#50030=ADVANCED_FACE('',(#14943),#12688,.F.);
#50031=ADVANCED_FACE('',(#14944),#1112,.T.);
#50032=ADVANCED_FACE('',(#14945),#12689,.T.);
#50033=ADVANCED_FACE('',(#14946),#12690,.T.);
#50034=ADVANCED_FACE('',(#14947),#12691,.T.);
#50035=ADVANCED_FACE('',(#14948),#12692,.F.);
#50036=ADVANCED_FACE('',(#14949),#1113,.T.);
#50037=ADVANCED_FACE('',(#14950),#12693,.T.);
#50038=ADVANCED_FACE('',(#14951),#12694,.T.);
#50039=ADVANCED_FACE('',(#14952),#12695,.T.);
#50040=ADVANCED_FACE('',(#14953),#12696,.F.);
#50041=ADVANCED_FACE('',(#14954),#1114,.T.);
#50042=ADVANCED_FACE('',(#14955),#12697,.T.);
#50043=ADVANCED_FACE('',(#14956),#12698,.T.);
#50044=ADVANCED_FACE('',(#14957),#12699,.T.);
#50045=ADVANCED_FACE('',(#14958),#12700,.F.);
#50046=ADVANCED_FACE('',(#14959),#1115,.T.);
#50047=ADVANCED_FACE('',(#14960),#12701,.T.);
#50048=ADVANCED_FACE('',(#14961),#12702,.T.);
#50049=ADVANCED_FACE('',(#14962),#12703,.T.);
#50050=ADVANCED_FACE('',(#14963),#12704,.F.);
#50051=ADVANCED_FACE('',(#14964),#1116,.T.);
#50052=ADVANCED_FACE('',(#14965),#12705,.T.);
#50053=ADVANCED_FACE('',(#14966),#12706,.T.);
#50054=ADVANCED_FACE('',(#14967),#12707,.T.);
#50055=ADVANCED_FACE('',(#14968),#12708,.F.);
#50056=ADVANCED_FACE('',(#14969),#1117,.T.);
#50057=ADVANCED_FACE('',(#14970),#12709,.T.);
#50058=ADVANCED_FACE('',(#14971),#12710,.T.);
#50059=ADVANCED_FACE('',(#14972),#12711,.T.);
#50060=ADVANCED_FACE('',(#14973),#12712,.F.);
#50061=ADVANCED_FACE('',(#14974),#1118,.T.);
#50062=ADVANCED_FACE('',(#14975),#12713,.T.);
#50063=ADVANCED_FACE('',(#14976),#12714,.T.);
#50064=ADVANCED_FACE('',(#14977),#12715,.T.);
#50065=ADVANCED_FACE('',(#14978),#12716,.F.);
#50066=ADVANCED_FACE('',(#14979),#1119,.T.);
#50067=ADVANCED_FACE('',(#14980),#12717,.T.);
#50068=ADVANCED_FACE('',(#14981),#12718,.T.);
#50069=ADVANCED_FACE('',(#14982),#12719,.T.);
#50070=ADVANCED_FACE('',(#14983),#12720,.F.);
#50071=ADVANCED_FACE('',(#14984),#950,.F.);
#50072=ADVANCED_FACE('',(#14985,#964),#12721,.T.);
#50073=ADVANCED_FACE('',(#14986),#1120,.F.);
#50074=ADVANCED_FACE('',(#14987),#951,.F.);
#50075=ADVANCED_FACE('',(#14988,#965),#12722,.T.);
#50076=ADVANCED_FACE('',(#14989),#1121,.F.);
#50077=ADVANCED_FACE('',(#14990),#952,.F.);
#50078=ADVANCED_FACE('',(#14991),#1122,.T.);
#50079=ADVANCED_FACE('',(#14992),#953,.F.);
#50080=ADVANCED_FACE('',(#14993),#1123,.T.);
#50081=ADVANCED_FACE('',(#14994),#1124,.F.);
#50082=ADVANCED_FACE('',(#14995),#48266,.F.);
#50083=ADVANCED_FACE('',(#14996,#966),#12723,.T.);
#50084=ADVANCED_FACE('',(#14997,#967),#12724,.T.);
#50085=ADVANCED_FACE('',(#14998,#968),#12725,.T.);
#50086=ADVANCED_FACE('',(#14999),#48267,.F.);
#51019=CLOSED_SHELL('',(#49722,#49723,#49724,#49725,#49726,#49727,#49728,
#49729,#49730,#49731,#49732,#49733,#49734,#49735,#49736,#49737,#49738,#49739,
#49740,#49741,#49742,#49743,#49744,#49745,#49746,#49747,#49748,#49749,#49750,
#49751,#49752,#49753,#49754,#49755,#49756,#49757,#49758,#49759,#49760,#49761,
#49762,#49763,#49764,#49765,#49766,#49767,#49768,#49769,#49770,#49771,#49772,
#49773,#49774,#49775,#49776,#49777,#49778,#49779,#49780,#49781,#49782,#49783,
#49784,#49785,#49786,#49787,#49788,#49789,#49790,#49791,#49792,#49793,#49794,
#49795,#49796,#49797,#49798,#49799,#49800,#49801,#49802,#49803,#49804,#49805,
#49806,#49807,#49808,#49809,#49810,#49811,#49812,#49813,#49814,#49815,#49816,
#49817,#49818,#49819,#49820,#49821,#49822,#49823,#49824,#49825,#49826,#49827,
#49828,#49829,#49830,#49831,#49832,#49833,#49834,#49835,#49836,#49837,#49838,
#49839,#49840,#49841,#49842,#49843,#49844,#49845,#49846,#49847,#49848,#49849,
#49850,#49851,#49852,#49853,#49854,#49855,#49856,#49857,#49858,#49859,#49860,
#49861,#49862,#49863,#49864,#49865,#49866,#49867,#49868,#49869,#49870,#49871,
#49872,#49873,#49874,#49875,#49876,#49877,#49878,#49879,#49880,#49881,#49882,
#49883,#49884,#49885,#49886,#49887,#49888,#49889,#49890,#49891,#49892,#49893,
#49894,#49895,#49896,#49897,#49898,#49899,#49900,#49901,#49902,#49903,#49904,
#49905,#49906,#49907,#49908,#49909,#49910,#49911,#49912,#49913,#49914,#49915,
#49916,#49917,#49918,#49919,#49920,#49921,#49922,#49923,#49924,#49925,#49926,
#49927,#49928,#49929,#49930,#49931,#49932,#49933,#49934,#49935,#49936,#49937,
#49938,#49939,#49940,#49941,#49942,#49943,#49944,#49945,#49946,#49947,#49948,
#49949,#49950,#49951,#49952,#49953,#49954,#49955,#49956,#49957,#49958,#49959,
#49960,#49961,#49962,#49963,#49964,#49965,#49966,#49967,#49968,#49969,#49970,
#49971,#49972,#49973,#49974,#49975,#49976,#49977,#49978,#49979,#49980,#49981,
#49982,#49983,#49984,#49985,#49986,#49987,#49988,#49989,#49990,#49991,#49992,
#49993,#49994,#49995,#49996,#49997,#49998,#49999,#50000,#50001,#50002,#50003,
#50004,#50005,#50006,#50007,#50008,#50009,#50010,#50011,#50012,#50013,#50014,
#50015,#50016,#50017,#50018,#50019,#50020,#50021,#50022,#50023,#50024,#50025,
#50026,#50027,#50028,#50029,#50030,#50031,#50032,#50033,#50034,#50035,#50036,
#50037,#50038,#50039,#50040,#50041,#50042,#50043,#50044,#50045,#50046,#50047,
#50048,#50049,#50050,#50051,#50052,#50053,#50054,#50055,#50056,#50057,#50058,
#50059,#50060,#50061,#50062,#50063,#50064,#50065,#50066,#50067,#50068,#50069,
#50070,#50071,#50072,#50073,#50074,#50075,#50076,#50077,#50078,#50079,#50080,
#50081,#50082,#50083,#50084,#50085,#50086));
#53608=AXIS2_PLACEMENT_3D('',#77416,#62885,#62886);
#53609=AXIS2_PLACEMENT_3D('',#77417,#62887,#62888);
#53610=AXIS2_PLACEMENT_3D('',#77434,#62893,#62894);
#53611=AXIS2_PLACEMENT_3D('',#77451,#62899,#62900);
#53612=AXIS2_PLACEMENT_3D('',#77454,#62903,#62904);
#53613=AXIS2_PLACEMENT_3D('',#77456,#62905,#62906);
#53614=AXIS2_PLACEMENT_3D('',#77459,#62908,#62909);
#53615=AXIS2_PLACEMENT_3D('',#77460,#62910,#62911);
#53616=AXIS2_PLACEMENT_3D('',#77462,#62912,#62913);
#53617=AXIS2_PLACEMENT_3D('',#77468,#62914,#62915);
#53618=AXIS2_PLACEMENT_3D('',#77482,#62916,#62917);
#53619=AXIS2_PLACEMENT_3D('',#77496,#62918,#62919);
#53620=AXIS2_PLACEMENT_3D('',#77510,#62920,#62921);
#53621=AXIS2_PLACEMENT_3D('',#77524,#62922,#62923);
#53622=AXIS2_PLACEMENT_3D('',#77538,#62924,#62925);
#53623=AXIS2_PLACEMENT_3D('',#77552,#62926,#62927);
#53624=AXIS2_PLACEMENT_3D('',#77566,#62928,#62929);
#53625=AXIS2_PLACEMENT_3D('',#77580,#62930,#62931);
#53626=AXIS2_PLACEMENT_3D('',#77594,#62932,#62933);
#53627=AXIS2_PLACEMENT_3D('',#77608,#62934,#62935);
#53628=AXIS2_PLACEMENT_3D('',#77621,#62936,#62937);
#53629=AXIS2_PLACEMENT_3D('',#77622,#62938,#62939);
#53630=AXIS2_PLACEMENT_3D('',#77624,#62940,#62941);
#53631=AXIS2_PLACEMENT_3D('',#77632,#62945,#62946);
#53632=AXIS2_PLACEMENT_3D('',#77639,#62950,#62951);
#53633=AXIS2_PLACEMENT_3D('',#77641,#62952,#62953);
#53634=AXIS2_PLACEMENT_3D('',#77642,#62954,#62955);
#53635=AXIS2_PLACEMENT_3D('',#77644,#62956,#62957);
#53636=AXIS2_PLACEMENT_3D('',#77658,#62958,#62959);
#53637=AXIS2_PLACEMENT_3D('',#77672,#62960,#62961);
#53638=AXIS2_PLACEMENT_3D('',#77686,#62962,#62963);
#53639=AXIS2_PLACEMENT_3D('',#77700,#62964,#62965);
#53640=AXIS2_PLACEMENT_3D('',#77714,#62966,#62967);
#53641=AXIS2_PLACEMENT_3D('',#77728,#62968,#62969);
#53642=AXIS2_PLACEMENT_3D('',#77742,#62970,#62971);
#53643=AXIS2_PLACEMENT_3D('',#77756,#62972,#62973);
#53644=AXIS2_PLACEMENT_3D('',#77770,#62974,#62975);
#53645=AXIS2_PLACEMENT_3D('',#77784,#62976,#62977);
#53646=AXIS2_PLACEMENT_3D('',#77798,#62978,#62979);
#53647=AXIS2_PLACEMENT_3D('',#77802,#62980,#62981);
#53648=AXIS2_PLACEMENT_3D('',#77808,#62982,#62983);
#53649=AXIS2_PLACEMENT_3D('',#77822,#62984,#62985);
#53650=AXIS2_PLACEMENT_3D('',#77836,#62986,#62987);
#53651=AXIS2_PLACEMENT_3D('',#77850,#62988,#62989);
#53652=AXIS2_PLACEMENT_3D('',#77864,#62990,#62991);
#53653=AXIS2_PLACEMENT_3D('',#77878,#62992,#62993);
#53654=AXIS2_PLACEMENT_3D('',#77892,#62994,#62995);
#53655=AXIS2_PLACEMENT_3D('',#77906,#62996,#62997);
#53656=AXIS2_PLACEMENT_3D('',#77920,#62998,#62999);
#53657=AXIS2_PLACEMENT_3D('',#77934,#63000,#63001);
#53658=AXIS2_PLACEMENT_3D('',#77948,#63002,#63003);
#53659=AXIS2_PLACEMENT_3D('',#77960,#63004,#63005);
#53660=AXIS2_PLACEMENT_3D('',#77965,#63009,#63010);
#53661=AXIS2_PLACEMENT_3D('',#77979,#63014,#63015);
#53662=AXIS2_PLACEMENT_3D('',#77981,#63017,#63018);
#53663=AXIS2_PLACEMENT_3D('',#77983,#63019,#63020);
#53664=AXIS2_PLACEMENT_3D('',#77989,#63021,#63022);
#53665=AXIS2_PLACEMENT_3D('',#78003,#63023,#63024);
#53666=AXIS2_PLACEMENT_3D('',#78017,#63025,#63026);
#53667=AXIS2_PLACEMENT_3D('',#78031,#63027,#63028);
#53668=AXIS2_PLACEMENT_3D('',#78045,#63029,#63030);
#53669=AXIS2_PLACEMENT_3D('',#78059,#63031,#63032);
#53670=AXIS2_PLACEMENT_3D('',#78073,#63033,#63034);
#53671=AXIS2_PLACEMENT_3D('',#78087,#63035,#63036);
#53672=AXIS2_PLACEMENT_3D('',#78101,#63037,#63038);
#53673=AXIS2_PLACEMENT_3D('',#78115,#63039,#63040);
#53674=AXIS2_PLACEMENT_3D('',#78129,#63041,#63042);
#53675=AXIS2_PLACEMENT_3D('',#78142,#63043,#63044);
#53676=AXIS2_PLACEMENT_3D('',#78143,#63045,#63046);
#53677=AXIS2_PLACEMENT_3D('',#78157,#63047,#63048);
#53678=AXIS2_PLACEMENT_3D('',#78171,#63049,#63050);
#53679=AXIS2_PLACEMENT_3D('',#78185,#63051,#63052);
#53680=AXIS2_PLACEMENT_3D('',#78199,#63053,#63054);
#53681=AXIS2_PLACEMENT_3D('',#78213,#63055,#63056);
#53682=AXIS2_PLACEMENT_3D('',#78227,#63057,#63058);
#53683=AXIS2_PLACEMENT_3D('',#78241,#63059,#63060);
#53684=AXIS2_PLACEMENT_3D('',#78255,#63061,#63062);
#53685=AXIS2_PLACEMENT_3D('',#78269,#63063,#63064);
#53686=AXIS2_PLACEMENT_3D('',#78283,#63065,#63066);
#53687=AXIS2_PLACEMENT_3D('',#78297,#63067,#63068);
#53688=AXIS2_PLACEMENT_3D('',#78302,#63069,#63070);
#53689=AXIS2_PLACEMENT_3D('',#78303,#63071,#63072);
#53690=AXIS2_PLACEMENT_3D('',#78305,#63074,#63075);
#53691=AXIS2_PLACEMENT_3D('',#78307,#63076,#63077);
#53692=AXIS2_PLACEMENT_3D('',#78321,#63078,#63079);
#53693=AXIS2_PLACEMENT_3D('',#78335,#63080,#63081);
#53694=AXIS2_PLACEMENT_3D('',#78349,#63082,#63083);
#53695=AXIS2_PLACEMENT_3D('',#78363,#63084,#63085);
#53696=AXIS2_PLACEMENT_3D('',#78377,#63086,#63087);
#53697=AXIS2_PLACEMENT_3D('',#78391,#63088,#63089);
#53698=AXIS2_PLACEMENT_3D('',#78405,#63090,#63091);
#53699=AXIS2_PLACEMENT_3D('',#78419,#63092,#63093);
#53700=AXIS2_PLACEMENT_3D('',#78433,#63094,#63095);
#53701=AXIS2_PLACEMENT_3D('',#78447,#63096,#63097);
#53702=AXIS2_PLACEMENT_3D('',#78461,#63098,#63099);
#53703=AXIS2_PLACEMENT_3D('',#78465,#63100,#63101);
#53704=AXIS2_PLACEMENT_3D('',#78470,#63105,#63106);
#53705=AXIS2_PLACEMENT_3D('',#78475,#63110,#63111);
#53706=AXIS2_PLACEMENT_3D('',#78477,#63113,#63114);
#53707=AXIS2_PLACEMENT_3D('',#78479,#63116,#63117);
#53708=AXIS2_PLACEMENT_3D('',#78493,#63118,#63119);
#53709=AXIS2_PLACEMENT_3D('',#78494,#63120,#63121);
#53710=AXIS2_PLACEMENT_3D('',#78508,#63122,#63123);
#53711=AXIS2_PLACEMENT_3D('',#78509,#63124,#63125);
#53712=AXIS2_PLACEMENT_3D('',#78523,#63126,#63127);
#53713=AXIS2_PLACEMENT_3D('',#78524,#63128,#63129);
#53714=AXIS2_PLACEMENT_3D('',#78538,#63130,#63131);
#53715=AXIS2_PLACEMENT_3D('',#78539,#63132,#63133);
#53716=AXIS2_PLACEMENT_3D('',#78553,#63134,#63135);
#53717=AXIS2_PLACEMENT_3D('',#78554,#63136,#63137);
#53718=AXIS2_PLACEMENT_3D('',#78568,#63138,#63139);
#53719=AXIS2_PLACEMENT_3D('',#78569,#63140,#63141);
#53720=AXIS2_PLACEMENT_3D('',#78583,#63142,#63143);
#53721=AXIS2_PLACEMENT_3D('',#78584,#63144,#63145);
#53722=AXIS2_PLACEMENT_3D('',#78598,#63146,#63147);
#53723=AXIS2_PLACEMENT_3D('',#78599,#63148,#63149);
#53724=AXIS2_PLACEMENT_3D('',#78613,#63150,#63151);
#53725=AXIS2_PLACEMENT_3D('',#78614,#63152,#63153);
#53726=AXIS2_PLACEMENT_3D('',#78628,#63154,#63155);
#53727=AXIS2_PLACEMENT_3D('',#78629,#63156,#63157);
#53728=AXIS2_PLACEMENT_3D('',#78643,#63158,#63159);
#53729=AXIS2_PLACEMENT_3D('',#78644,#63160,#63161);
#53730=AXIS2_PLACEMENT_3D('',#78658,#63162,#63163);
#53731=AXIS2_PLACEMENT_3D('',#78659,#63164,#63165);
#53732=AXIS2_PLACEMENT_3D('',#78673,#63166,#63167);
#53733=AXIS2_PLACEMENT_3D('',#78674,#63168,#63169);
#53734=AXIS2_PLACEMENT_3D('',#78688,#63170,#63171);
#53735=AXIS2_PLACEMENT_3D('',#78689,#63172,#63173);
#53736=AXIS2_PLACEMENT_3D('',#78703,#63174,#63175);
#53737=AXIS2_PLACEMENT_3D('',#78704,#63176,#63177);
#53738=AXIS2_PLACEMENT_3D('',#78718,#63178,#63179);
#53739=AXIS2_PLACEMENT_3D('',#78719,#63180,#63181);
#53740=AXIS2_PLACEMENT_3D('',#78733,#63182,#63183);
#53741=AXIS2_PLACEMENT_3D('',#78734,#63184,#63185);
#53742=AXIS2_PLACEMENT_3D('',#78748,#63186,#63187);
#53743=AXIS2_PLACEMENT_3D('',#78749,#63188,#63189);
#53744=AXIS2_PLACEMENT_3D('',#78763,#63190,#63191);
#53745=AXIS2_PLACEMENT_3D('',#78764,#63192,#63193);
#53746=AXIS2_PLACEMENT_3D('',#78778,#63194,#63195);
#53747=AXIS2_PLACEMENT_3D('',#78779,#63196,#63197);
#53748=AXIS2_PLACEMENT_3D('',#78793,#63198,#63199);
#53749=AXIS2_PLACEMENT_3D('',#78794,#63200,#63201);
#53750=AXIS2_PLACEMENT_3D('',#78808,#63202,#63203);
#53751=AXIS2_PLACEMENT_3D('',#78809,#63204,#63205);
#53752=AXIS2_PLACEMENT_3D('',#78823,#63206,#63207);
#53753=AXIS2_PLACEMENT_3D('',#78824,#63208,#63209);
#53754=AXIS2_PLACEMENT_3D('',#78838,#63210,#63211);
#53755=AXIS2_PLACEMENT_3D('',#78839,#63212,#63213);
#53756=AXIS2_PLACEMENT_3D('',#78853,#63214,#63215);
#53757=AXIS2_PLACEMENT_3D('',#78854,#63216,#63217);
#53758=AXIS2_PLACEMENT_3D('',#78868,#63218,#63219);
#53759=AXIS2_PLACEMENT_3D('',#78869,#63220,#63221);
#53760=AXIS2_PLACEMENT_3D('',#78883,#63222,#63223);
#53761=AXIS2_PLACEMENT_3D('',#78884,#63224,#63225);
#53762=AXIS2_PLACEMENT_3D('',#78898,#63226,#63227);
#53763=AXIS2_PLACEMENT_3D('',#78899,#63228,#63229);
#53764=AXIS2_PLACEMENT_3D('',#78913,#63230,#63231);
#53765=AXIS2_PLACEMENT_3D('',#78914,#63232,#63233);
#53766=AXIS2_PLACEMENT_3D('',#78928,#63234,#63235);
#53767=AXIS2_PLACEMENT_3D('',#78929,#63236,#63237);
#53768=AXIS2_PLACEMENT_3D('',#78943,#63238,#63239);
#53769=AXIS2_PLACEMENT_3D('',#78944,#63240,#63241);
#53770=AXIS2_PLACEMENT_3D('',#78958,#63242,#63243);
#53771=AXIS2_PLACEMENT_3D('',#78959,#63244,#63245);
#53772=AXIS2_PLACEMENT_3D('',#78973,#63246,#63247);
#53773=AXIS2_PLACEMENT_3D('',#78974,#63248,#63249);
#53774=AXIS2_PLACEMENT_3D('',#78988,#63256,#63257);
#53775=AXIS2_PLACEMENT_3D('',#78994,#63259,#63260);
#53776=AXIS2_PLACEMENT_3D('',#79008,#63267,#63268);
#53777=AXIS2_PLACEMENT_3D('',#79014,#63270,#63271);
#53778=AXIS2_PLACEMENT_3D('',#79028,#63278,#63279);
#53779=AXIS2_PLACEMENT_3D('',#79034,#63281,#63282);
#53780=AXIS2_PLACEMENT_3D('',#79048,#63289,#63290);
#53781=AXIS2_PLACEMENT_3D('',#79054,#63292,#63293);
#53782=AXIS2_PLACEMENT_3D('',#79068,#63300,#63301);
#53783=AXIS2_PLACEMENT_3D('',#79074,#63303,#63304);
#53784=AXIS2_PLACEMENT_3D('',#79088,#63311,#63312);
#53785=AXIS2_PLACEMENT_3D('',#79094,#63314,#63315);
#53786=AXIS2_PLACEMENT_3D('',#79108,#63322,#63323);
#53787=AXIS2_PLACEMENT_3D('',#79114,#63325,#63326);
#53788=AXIS2_PLACEMENT_3D('',#79128,#63333,#63334);
#53789=AXIS2_PLACEMENT_3D('',#79134,#63336,#63337);
#53790=AXIS2_PLACEMENT_3D('',#79148,#63344,#63345);
#53791=AXIS2_PLACEMENT_3D('',#79154,#63347,#63348);
#53792=AXIS2_PLACEMENT_3D('',#79168,#63355,#63356);
#53793=AXIS2_PLACEMENT_3D('',#79174,#63358,#63359);
#53794=AXIS2_PLACEMENT_3D('',#79188,#63366,#63367);
#53795=AXIS2_PLACEMENT_3D('',#79194,#63369,#63370);
#53796=AXIS2_PLACEMENT_3D('',#79208,#63377,#63378);
#53797=AXIS2_PLACEMENT_3D('',#79214,#63380,#63381);
#53798=AXIS2_PLACEMENT_3D('',#79228,#63388,#63389);
#53799=AXIS2_PLACEMENT_3D('',#79234,#63391,#63392);
#53800=AXIS2_PLACEMENT_3D('',#79248,#63399,#63400);
#53801=AXIS2_PLACEMENT_3D('',#79254,#63402,#63403);
#53802=AXIS2_PLACEMENT_3D('',#79268,#63410,#63411);
#53803=AXIS2_PLACEMENT_3D('',#79274,#63413,#63414);
#53804=AXIS2_PLACEMENT_3D('',#79288,#63421,#63422);
#53805=AXIS2_PLACEMENT_3D('',#79294,#63424,#63425);
#53806=AXIS2_PLACEMENT_3D('',#79308,#63432,#63433);
#53807=AXIS2_PLACEMENT_3D('',#79314,#63435,#63436);
#53808=AXIS2_PLACEMENT_3D('',#79328,#63443,#63444);
#53809=AXIS2_PLACEMENT_3D('',#79334,#63446,#63447);
#53810=AXIS2_PLACEMENT_3D('',#79348,#63454,#63455);
#53811=AXIS2_PLACEMENT_3D('',#79354,#63457,#63458);
#53812=AXIS2_PLACEMENT_3D('',#79368,#63465,#63466);
#53813=AXIS2_PLACEMENT_3D('',#79374,#63468,#63469);
#53814=AXIS2_PLACEMENT_3D('',#79388,#63476,#63477);
#53815=AXIS2_PLACEMENT_3D('',#79394,#63479,#63480);
#53816=AXIS2_PLACEMENT_3D('',#79408,#63487,#63488);
#53817=AXIS2_PLACEMENT_3D('',#79414,#63490,#63491);
#53818=AXIS2_PLACEMENT_3D('',#79428,#63498,#63499);
#53819=AXIS2_PLACEMENT_3D('',#79434,#63501,#63502);
#53820=AXIS2_PLACEMENT_3D('',#79448,#63509,#63510);
#53821=AXIS2_PLACEMENT_3D('',#79454,#63512,#63513);
#53822=AXIS2_PLACEMENT_3D('',#79468,#63520,#63521);
#53823=AXIS2_PLACEMENT_3D('',#79474,#63523,#63524);
#53824=AXIS2_PLACEMENT_3D('',#79488,#63531,#63532);
#53825=AXIS2_PLACEMENT_3D('',#79494,#63534,#63535);
#53826=AXIS2_PLACEMENT_3D('',#79508,#63542,#63543);
#53827=AXIS2_PLACEMENT_3D('',#79514,#63545,#63546);
#53828=AXIS2_PLACEMENT_3D('',#79528,#63553,#63554);
#53829=AXIS2_PLACEMENT_3D('',#79534,#63556,#63557);
#53830=AXIS2_PLACEMENT_3D('',#79548,#63564,#63565);
#53831=AXIS2_PLACEMENT_3D('',#79554,#63567,#63568);
#53832=AXIS2_PLACEMENT_3D('',#79568,#63575,#63576);
#53833=AXIS2_PLACEMENT_3D('',#79574,#63578,#63579);
#53834=AXIS2_PLACEMENT_3D('',#79588,#63586,#63587);
#53835=AXIS2_PLACEMENT_3D('',#79594,#63589,#63590);
#53836=AXIS2_PLACEMENT_3D('',#79608,#63597,#63598);
#53837=AXIS2_PLACEMENT_3D('',#79614,#63600,#63601);
#53838=AXIS2_PLACEMENT_3D('',#79628,#63608,#63609);
#53839=AXIS2_PLACEMENT_3D('',#79634,#63611,#63612);
#53840=AXIS2_PLACEMENT_3D('',#79639,#63613,#63614);
#53841=AXIS2_PLACEMENT_3D('',#79640,#63615,#63616);
#53842=AXIS2_PLACEMENT_3D('',#79645,#63617,#63618);
#53843=AXIS2_PLACEMENT_3D('',#79646,#63619,#63620);
#53844=AXIS2_PLACEMENT_3D('',#79651,#63621,#63622);
#53845=AXIS2_PLACEMENT_3D('',#79652,#63623,#63624);
#53846=AXIS2_PLACEMENT_3D('',#79657,#63625,#63626);
#53847=AXIS2_PLACEMENT_3D('',#79658,#63627,#63628);
#53848=AXIS2_PLACEMENT_3D('',#79663,#63629,#63630);
#53849=AXIS2_PLACEMENT_3D('',#79664,#63631,#63632);
#53850=AXIS2_PLACEMENT_3D('',#79669,#63633,#63634);
#53851=AXIS2_PLACEMENT_3D('',#79670,#63635,#63636);
#53852=AXIS2_PLACEMENT_3D('',#79675,#63637,#63638);
#53853=AXIS2_PLACEMENT_3D('',#79676,#63639,#63640);
#53854=AXIS2_PLACEMENT_3D('',#79681,#63641,#63642);
#53855=AXIS2_PLACEMENT_3D('',#79682,#63643,#63644);
#53856=AXIS2_PLACEMENT_3D('',#79687,#63645,#63646);
#53857=AXIS2_PLACEMENT_3D('',#79688,#63647,#63648);
#53858=AXIS2_PLACEMENT_3D('',#79693,#63649,#63650);
#53859=AXIS2_PLACEMENT_3D('',#79694,#63651,#63652);
#53860=AXIS2_PLACEMENT_3D('',#79699,#63653,#63654);
#53861=AXIS2_PLACEMENT_3D('',#79700,#63655,#63656);
#53862=AXIS2_PLACEMENT_3D('',#79705,#63657,#63658);
#53863=AXIS2_PLACEMENT_3D('',#79706,#63659,#63660);
#53864=AXIS2_PLACEMENT_3D('',#79711,#63661,#63662);
#53865=AXIS2_PLACEMENT_3D('',#79712,#63663,#63664);
#53866=AXIS2_PLACEMENT_3D('',#79717,#63665,#63666);
#53867=AXIS2_PLACEMENT_3D('',#79718,#63667,#63668);
#53868=AXIS2_PLACEMENT_3D('',#79723,#63669,#63670);
#53869=AXIS2_PLACEMENT_3D('',#79724,#63671,#63672);
#53870=AXIS2_PLACEMENT_3D('',#79729,#63673,#63674);
#53871=AXIS2_PLACEMENT_3D('',#79730,#63675,#63676);
#53872=AXIS2_PLACEMENT_3D('',#79735,#63677,#63678);
#53873=AXIS2_PLACEMENT_3D('',#79736,#63679,#63680);
#53874=AXIS2_PLACEMENT_3D('',#79741,#63681,#63682);
#53875=AXIS2_PLACEMENT_3D('',#79742,#63683,#63684);
#53876=AXIS2_PLACEMENT_3D('',#79747,#63685,#63686);
#53877=AXIS2_PLACEMENT_3D('',#79748,#63687,#63688);
#53878=AXIS2_PLACEMENT_3D('',#79753,#63689,#63690);
#53879=AXIS2_PLACEMENT_3D('',#79754,#63691,#63692);
#53880=AXIS2_PLACEMENT_3D('',#79759,#63693,#63694);
#53881=AXIS2_PLACEMENT_3D('',#79760,#63695,#63696);
#53882=AXIS2_PLACEMENT_3D('',#79765,#63697,#63698);
#53883=AXIS2_PLACEMENT_3D('',#79766,#63699,#63700);
#53884=AXIS2_PLACEMENT_3D('',#79771,#63701,#63702);
#53885=AXIS2_PLACEMENT_3D('',#79772,#63703,#63704);
#53886=AXIS2_PLACEMENT_3D('',#79777,#63705,#63706);
#53887=AXIS2_PLACEMENT_3D('',#79778,#63707,#63708);
#53888=AXIS2_PLACEMENT_3D('',#79783,#63709,#63710);
#53889=AXIS2_PLACEMENT_3D('',#79784,#63711,#63712);
#53890=AXIS2_PLACEMENT_3D('',#79789,#63713,#63714);
#53891=AXIS2_PLACEMENT_3D('',#79790,#63715,#63716);
#53892=AXIS2_PLACEMENT_3D('',#79795,#63717,#63718);
#53893=AXIS2_PLACEMENT_3D('',#79796,#63719,#63720);
#53894=AXIS2_PLACEMENT_3D('',#79801,#63721,#63722);
#53895=AXIS2_PLACEMENT_3D('',#79802,#63723,#63724);
#53896=AXIS2_PLACEMENT_3D('',#79807,#63725,#63726);
#53897=AXIS2_PLACEMENT_3D('',#79808,#63727,#63728);
#53898=AXIS2_PLACEMENT_3D('',#79813,#63729,#63730);
#53899=AXIS2_PLACEMENT_3D('',#79814,#63731,#63732);
#53900=AXIS2_PLACEMENT_3D('',#79819,#63733,#63734);
#53901=AXIS2_PLACEMENT_3D('',#79820,#63735,#63736);
#53902=AXIS2_PLACEMENT_3D('',#79825,#63737,#63738);
#53903=AXIS2_PLACEMENT_3D('',#79826,#63739,#63740);
#53904=AXIS2_PLACEMENT_3D('',#79831,#63741,#63742);
#53905=AXIS2_PLACEMENT_3D('',#79832,#63743,#63744);
#53906=AXIS2_PLACEMENT_3D('',#79840,#63750,#63751);
#53907=AXIS2_PLACEMENT_3D('',#79848,#63757,#63758);
#53908=AXIS2_PLACEMENT_3D('',#79856,#63764,#63765);
#53909=AXIS2_PLACEMENT_3D('',#79864,#63771,#63772);
#53910=AXIS2_PLACEMENT_3D('',#79872,#63778,#63779);
#53911=AXIS2_PLACEMENT_3D('',#79880,#63785,#63786);
#53912=AXIS2_PLACEMENT_3D('',#79888,#63792,#63793);
#53913=AXIS2_PLACEMENT_3D('',#79896,#63799,#63800);
#53914=AXIS2_PLACEMENT_3D('',#79904,#63806,#63807);
#53915=AXIS2_PLACEMENT_3D('',#79912,#63813,#63814);
#53916=AXIS2_PLACEMENT_3D('',#79919,#63819,#63820);
#53917=AXIS2_PLACEMENT_3D('',#79927,#63826,#63827);
#53918=AXIS2_PLACEMENT_3D('',#79935,#63833,#63834);
#53919=AXIS2_PLACEMENT_3D('',#79943,#63840,#63841);
#53920=AXIS2_PLACEMENT_3D('',#79951,#63847,#63848);
#53921=AXIS2_PLACEMENT_3D('',#79959,#63854,#63855);
#53922=AXIS2_PLACEMENT_3D('',#79967,#63861,#63862);
#53923=AXIS2_PLACEMENT_3D('',#79975,#63868,#63869);
#53924=AXIS2_PLACEMENT_3D('',#79983,#63875,#63876);
#53925=AXIS2_PLACEMENT_3D('',#79991,#63882,#63883);
#53926=AXIS2_PLACEMENT_3D('',#79999,#63889,#63890);
#53927=AXIS2_PLACEMENT_3D('',#80006,#63895,#63896);
#53928=AXIS2_PLACEMENT_3D('',#80014,#63902,#63903);
#53929=AXIS2_PLACEMENT_3D('',#80022,#63909,#63910);
#53930=AXIS2_PLACEMENT_3D('',#80030,#63916,#63917);
#53931=AXIS2_PLACEMENT_3D('',#80038,#63923,#63924);
#53932=AXIS2_PLACEMENT_3D('',#80046,#63930,#63931);
#53933=AXIS2_PLACEMENT_3D('',#80054,#63937,#63938);
#53934=AXIS2_PLACEMENT_3D('',#80062,#63944,#63945);
#53935=AXIS2_PLACEMENT_3D('',#80070,#63951,#63952);
#53936=AXIS2_PLACEMENT_3D('',#80078,#63958,#63959);
#53937=AXIS2_PLACEMENT_3D('',#80086,#63965,#63966);
#53938=AXIS2_PLACEMENT_3D('',#80093,#63971,#63972);
#53939=AXIS2_PLACEMENT_3D('',#80095,#63974,#63975);
#53940=AXIS2_PLACEMENT_3D('',#80097,#63977,#63978);
#53941=AXIS2_PLACEMENT_3D('',#80098,#63979,#63980);
#53942=AXIS2_PLACEMENT_3D('',#80099,#63981,#63982);
#53943=AXIS2_PLACEMENT_3D('',#80100,#63983,#63984);
#53944=AXIS2_PLACEMENT_3D('',#80101,#63985,#63986);
#53945=AXIS2_PLACEMENT_3D('',#80103,#63988,#63989);
#53946=AXIS2_PLACEMENT_3D('',#80105,#63991,#63992);
#53947=AXIS2_PLACEMENT_3D('',#80106,#63993,#63994);
#53948=AXIS2_PLACEMENT_3D('',#80107,#63995,#63996);
#53949=AXIS2_PLACEMENT_3D('',#80108,#63997,#63998);
#53950=AXIS2_PLACEMENT_3D('',#80110,#64000,#64001);
#53951=AXIS2_PLACEMENT_3D('',#80112,#64003,#64004);
#53952=AXIS2_PLACEMENT_3D('',#80113,#64005,#64006);
#53953=AXIS2_PLACEMENT_3D('',#80114,#64007,#64008);
#53954=AXIS2_PLACEMENT_3D('',#80115,#64009,#64010);
#53955=AXIS2_PLACEMENT_3D('',#80117,#64012,#64013);
#53956=AXIS2_PLACEMENT_3D('',#80119,#64015,#64016);
#53957=AXIS2_PLACEMENT_3D('',#80120,#64017,#64018);
#53958=AXIS2_PLACEMENT_3D('',#80121,#64019,#64020);
#53959=AXIS2_PLACEMENT_3D('',#80122,#64021,#64022);
#53960=AXIS2_PLACEMENT_3D('',#80124,#64024,#64025);
#53961=AXIS2_PLACEMENT_3D('',#80126,#64027,#64028);
#53962=AXIS2_PLACEMENT_3D('',#80127,#64029,#64030);
#53963=AXIS2_PLACEMENT_3D('',#80128,#64031,#64032);
#53964=AXIS2_PLACEMENT_3D('',#80129,#64033,#64034);
#53965=AXIS2_PLACEMENT_3D('',#80131,#64036,#64037);
#53966=AXIS2_PLACEMENT_3D('',#80133,#64039,#64040);
#53967=AXIS2_PLACEMENT_3D('',#80134,#64041,#64042);
#53968=AXIS2_PLACEMENT_3D('',#80135,#64043,#64044);
#53969=AXIS2_PLACEMENT_3D('',#80136,#64045,#64046);
#53970=AXIS2_PLACEMENT_3D('',#80138,#64048,#64049);
#53971=AXIS2_PLACEMENT_3D('',#80140,#64051,#64052);
#53972=AXIS2_PLACEMENT_3D('',#80141,#64053,#64054);
#53973=AXIS2_PLACEMENT_3D('',#80142,#64055,#64056);
#53974=AXIS2_PLACEMENT_3D('',#80143,#64057,#64058);
#53975=AXIS2_PLACEMENT_3D('',#80145,#64060,#64061);
#53976=AXIS2_PLACEMENT_3D('',#80147,#64063,#64064);
#53977=AXIS2_PLACEMENT_3D('',#80148,#64065,#64066);
#53978=AXIS2_PLACEMENT_3D('',#80149,#64067,#64068);
#53979=AXIS2_PLACEMENT_3D('',#80150,#64069,#64070);
#53980=AXIS2_PLACEMENT_3D('',#80152,#64072,#64073);
#53981=AXIS2_PLACEMENT_3D('',#80154,#64075,#64076);
#53982=AXIS2_PLACEMENT_3D('',#80155,#64077,#64078);
#53983=AXIS2_PLACEMENT_3D('',#80156,#64079,#64080);
#53984=AXIS2_PLACEMENT_3D('',#80157,#64081,#64082);
#53985=AXIS2_PLACEMENT_3D('',#80159,#64084,#64085);
#53986=AXIS2_PLACEMENT_3D('',#80161,#64087,#64088);
#53987=AXIS2_PLACEMENT_3D('',#80162,#64089,#64090);
#53988=AXIS2_PLACEMENT_3D('',#80163,#64091,#64092);
#53989=AXIS2_PLACEMENT_3D('',#80164,#64093,#64094);
#53990=AXIS2_PLACEMENT_3D('',#80166,#64096,#64097);
#53991=AXIS2_PLACEMENT_3D('',#80168,#64099,#64100);
#53992=AXIS2_PLACEMENT_3D('',#80169,#64101,#64102);
#53993=AXIS2_PLACEMENT_3D('',#80170,#64103,#64104);
#53994=AXIS2_PLACEMENT_3D('',#80171,#64105,#64106);
#53995=AXIS2_PLACEMENT_3D('',#80173,#64108,#64109);
#53996=AXIS2_PLACEMENT_3D('',#80175,#64111,#64112);
#53997=AXIS2_PLACEMENT_3D('',#80176,#64113,#64114);
#53998=AXIS2_PLACEMENT_3D('',#80177,#64115,#64116);
#53999=AXIS2_PLACEMENT_3D('',#80178,#64117,#64118);
#54000=AXIS2_PLACEMENT_3D('',#80180,#64120,#64121);
#54001=AXIS2_PLACEMENT_3D('',#80182,#64123,#64124);
#54002=AXIS2_PLACEMENT_3D('',#80183,#64125,#64126);
#54003=AXIS2_PLACEMENT_3D('',#80184,#64127,#64128);
#54004=AXIS2_PLACEMENT_3D('',#80185,#64129,#64130);
#54005=AXIS2_PLACEMENT_3D('',#80187,#64132,#64133);
#54006=AXIS2_PLACEMENT_3D('',#80189,#64135,#64136);
#54007=AXIS2_PLACEMENT_3D('',#80190,#64137,#64138);
#54008=AXIS2_PLACEMENT_3D('',#80191,#64139,#64140);
#54009=AXIS2_PLACEMENT_3D('',#80192,#64141,#64142);
#54010=AXIS2_PLACEMENT_3D('',#80194,#64144,#64145);
#54011=AXIS2_PLACEMENT_3D('',#80196,#64147,#64148);
#54012=AXIS2_PLACEMENT_3D('',#80197,#64149,#64150);
#54013=AXIS2_PLACEMENT_3D('',#80198,#64151,#64152);
#54014=AXIS2_PLACEMENT_3D('',#80199,#64153,#64154);
#54015=AXIS2_PLACEMENT_3D('',#80201,#64156,#64157);
#54016=AXIS2_PLACEMENT_3D('',#80203,#64159,#64160);
#54017=AXIS2_PLACEMENT_3D('',#80204,#64161,#64162);
#54018=AXIS2_PLACEMENT_3D('',#80205,#64163,#64164);
#54019=AXIS2_PLACEMENT_3D('',#80206,#64165,#64166);
#54020=AXIS2_PLACEMENT_3D('',#80208,#64168,#64169);
#54021=AXIS2_PLACEMENT_3D('',#80210,#64171,#64172);
#54022=AXIS2_PLACEMENT_3D('',#80211,#64173,#64174);
#54023=AXIS2_PLACEMENT_3D('',#80212,#64175,#64176);
#54024=AXIS2_PLACEMENT_3D('',#80213,#64177,#64178);
#54025=AXIS2_PLACEMENT_3D('',#80215,#64180,#64181);
#54026=AXIS2_PLACEMENT_3D('',#80217,#64183,#64184);
#54027=AXIS2_PLACEMENT_3D('',#80218,#64185,#64186);
#54028=AXIS2_PLACEMENT_3D('',#80219,#64187,#64188);
#54029=AXIS2_PLACEMENT_3D('',#80220,#64189,#64190);
#54030=AXIS2_PLACEMENT_3D('',#80222,#64192,#64193);
#54031=AXIS2_PLACEMENT_3D('',#80224,#64195,#64196);
#54032=AXIS2_PLACEMENT_3D('',#80225,#64197,#64198);
#54033=AXIS2_PLACEMENT_3D('',#80226,#64199,#64200);
#54034=AXIS2_PLACEMENT_3D('',#80227,#64201,#64202);
#54035=AXIS2_PLACEMENT_3D('',#80229,#64204,#64205);
#54036=AXIS2_PLACEMENT_3D('',#80231,#64207,#64208);
#54037=AXIS2_PLACEMENT_3D('',#80232,#64209,#64210);
#54038=AXIS2_PLACEMENT_3D('',#80233,#64211,#64212);
#54039=AXIS2_PLACEMENT_3D('',#80234,#64213,#64214);
#54040=AXIS2_PLACEMENT_3D('',#80236,#64216,#64217);
#54041=AXIS2_PLACEMENT_3D('',#80238,#64219,#64220);
#54042=AXIS2_PLACEMENT_3D('',#80239,#64221,#64222);
#54043=AXIS2_PLACEMENT_3D('',#80240,#64223,#64224);
#54044=AXIS2_PLACEMENT_3D('',#80241,#64225,#64226);
#54045=AXIS2_PLACEMENT_3D('',#80243,#64228,#64229);
#54046=AXIS2_PLACEMENT_3D('',#80245,#64231,#64232);
#54047=AXIS2_PLACEMENT_3D('',#80246,#64233,#64234);
#54048=AXIS2_PLACEMENT_3D('',#80247,#64235,#64236);
#54049=AXIS2_PLACEMENT_3D('',#80248,#64237,#64238);
#54050=AXIS2_PLACEMENT_3D('',#80250,#64240,#64241);
#54051=AXIS2_PLACEMENT_3D('',#80252,#64243,#64244);
#54052=AXIS2_PLACEMENT_3D('',#80253,#64245,#64246);
#54053=AXIS2_PLACEMENT_3D('',#80254,#64247,#64248);
#54054=AXIS2_PLACEMENT_3D('',#80255,#64249,#64250);
#54055=AXIS2_PLACEMENT_3D('',#80257,#64252,#64253);
#54056=AXIS2_PLACEMENT_3D('',#80259,#64255,#64256);
#54057=AXIS2_PLACEMENT_3D('',#80260,#64257,#64258);
#54058=AXIS2_PLACEMENT_3D('',#80261,#64259,#64260);
#54059=AXIS2_PLACEMENT_3D('',#80262,#64261,#64262);
#54060=AXIS2_PLACEMENT_3D('',#80264,#64264,#64265);
#54061=AXIS2_PLACEMENT_3D('',#80266,#64267,#64268);
#54062=AXIS2_PLACEMENT_3D('',#80267,#64269,#64270);
#54063=AXIS2_PLACEMENT_3D('',#80268,#64271,#64272);
#54064=AXIS2_PLACEMENT_3D('',#80269,#64273,#64274);
#54065=AXIS2_PLACEMENT_3D('',#80271,#64276,#64277);
#54066=AXIS2_PLACEMENT_3D('',#80273,#64279,#64280);
#54067=AXIS2_PLACEMENT_3D('',#80274,#64281,#64282);
#54068=AXIS2_PLACEMENT_3D('',#80275,#64283,#64284);
#54069=AXIS2_PLACEMENT_3D('',#80276,#64285,#64286);
#54070=AXIS2_PLACEMENT_3D('',#80278,#64288,#64289);
#54071=AXIS2_PLACEMENT_3D('',#80280,#64291,#64292);
#54072=AXIS2_PLACEMENT_3D('',#80281,#64293,#64294);
#54073=AXIS2_PLACEMENT_3D('',#80282,#64295,#64296);
#54074=AXIS2_PLACEMENT_3D('',#80283,#64297,#64298);
#54075=AXIS2_PLACEMENT_3D('',#80285,#64300,#64301);
#54076=AXIS2_PLACEMENT_3D('',#80287,#64303,#64304);
#54077=AXIS2_PLACEMENT_3D('',#80288,#64305,#64306);
#54078=AXIS2_PLACEMENT_3D('',#80289,#64307,#64308);
#54079=AXIS2_PLACEMENT_3D('',#80290,#64309,#64310);
#54080=AXIS2_PLACEMENT_3D('',#80292,#64312,#64313);
#54081=AXIS2_PLACEMENT_3D('',#80294,#64315,#64316);
#54082=AXIS2_PLACEMENT_3D('',#80295,#64317,#64318);
#54083=AXIS2_PLACEMENT_3D('',#80296,#64319,#64320);
#54084=AXIS2_PLACEMENT_3D('',#80297,#64321,#64322);
#54085=AXIS2_PLACEMENT_3D('',#80299,#64324,#64325);
#54086=AXIS2_PLACEMENT_3D('',#80301,#64327,#64328);
#54087=AXIS2_PLACEMENT_3D('',#80302,#64329,#64330);
#54088=AXIS2_PLACEMENT_3D('',#80303,#64331,#64332);
#54089=AXIS2_PLACEMENT_3D('',#80304,#64333,#64334);
#54090=AXIS2_PLACEMENT_3D('',#80306,#64336,#64337);
#54091=AXIS2_PLACEMENT_3D('',#80308,#64339,#64340);
#54092=AXIS2_PLACEMENT_3D('',#80309,#64341,#64342);
#54093=AXIS2_PLACEMENT_3D('',#80310,#64343,#64344);
#54094=AXIS2_PLACEMENT_3D('',#80311,#64345,#64346);
#54095=AXIS2_PLACEMENT_3D('',#80313,#64348,#64349);
#54096=AXIS2_PLACEMENT_3D('',#80315,#64351,#64352);
#54097=AXIS2_PLACEMENT_3D('',#80316,#64353,#64354);
#54098=AXIS2_PLACEMENT_3D('',#80317,#64355,#64356);
#54099=AXIS2_PLACEMENT_3D('',#80318,#64357,#64358);
#54100=AXIS2_PLACEMENT_3D('',#80320,#64360,#64361);
#54101=AXIS2_PLACEMENT_3D('',#80322,#64363,#64364);
#54102=AXIS2_PLACEMENT_3D('',#80323,#64365,#64366);
#54103=AXIS2_PLACEMENT_3D('',#80324,#64367,#64368);
#54104=AXIS2_PLACEMENT_3D('',#80327,#64369,#64370);
#54105=AXIS2_PLACEMENT_3D('',#80329,#64371,#64372);
#54106=AXIS2_PLACEMENT_3D('',#80330,#64373,#64374);
#54107=AXIS2_PLACEMENT_3D('',#80331,#64375,#64376);
#54108=AXIS2_PLACEMENT_3D('',#80332,#64377,#64378);
#54109=AXIS2_PLACEMENT_3D('',#80334,#64379,#64380);
#54110=AXIS2_PLACEMENT_3D('',#80335,#64381,#64382);
#54111=AXIS2_PLACEMENT_3D('',#80337,#64383,#64384);
#54112=AXIS2_PLACEMENT_3D('',#80339,#64386,#64387);
#54113=AXIS2_PLACEMENT_3D('',#80341,#64388,#64389);
#54114=AXIS2_PLACEMENT_3D('',#80343,#64390,#64391);
#54115=AXIS2_PLACEMENT_3D('',#80345,#64392,#64393);
#54116=AXIS2_PLACEMENT_3D('',#80346,#64394,#64395);
#54117=AXIS2_PLACEMENT_3D('',#80347,#64396,#64397);
#54118=AXIS2_PLACEMENT_3D('',#80349,#64398,#64399);
#54119=AXIS2_PLACEMENT_3D('',#80350,#64400,#64401);
#54120=AXIS2_PLACEMENT_3D('',#80352,#64403,#64404);
#54121=AXIS2_PLACEMENT_3D('',#80354,#64405,#64406);
#54122=AXIS2_PLACEMENT_3D('',#80356,#64407,#64408);
#54123=AXIS2_PLACEMENT_3D('',#80357,#64409,#64410);
#54124=AXIS2_PLACEMENT_3D('',#80358,#64411,#64412);
#54125=AXIS2_PLACEMENT_3D('',#80360,#64413,#64414);
#54126=AXIS2_PLACEMENT_3D('',#80362,#64416,#64417);
#54127=AXIS2_PLACEMENT_3D('',#80365,#64418,#64419);
#54128=AXIS2_PLACEMENT_3D('',#80366,#64420,#64421);
#54129=AXIS2_PLACEMENT_3D('',#80367,#64422,#64423);
#54130=AXIS2_PLACEMENT_3D('',#80368,#64424,#64425);
#54131=AXIS2_PLACEMENT_3D('',#80371,#64427,#64428);
#54132=AXIS2_PLACEMENT_3D('',#80372,#64429,#64430);
#54133=AXIS2_PLACEMENT_3D('',#80374,#64431,#64432);
#54134=AXIS2_PLACEMENT_3D('',#80377,#64434,#64435);
#54135=AXIS2_PLACEMENT_3D('',#80378,#64436,#64437);
#54136=AXIS2_PLACEMENT_3D('',#80381,#64439,#64440);
#54137=AXIS2_PLACEMENT_3D('',#80382,#64441,#64442);
#54138=AXIS2_PLACEMENT_3D('',#80383,#64443,#64444);
#54139=AXIS2_PLACEMENT_3D('',#80384,#64445,#64446);
#54140=AXIS2_PLACEMENT_3D('',#80386,#64447,#64448);
#54141=AXIS2_PLACEMENT_3D('',#80387,#64449,#64450);
#62885=DIRECTION('axis',(0.,0.,1.));
#62886=DIRECTION('refdir',(1.,0.,0.));
#62887=DIRECTION('center_axis',(0.,0.90630778703665,-0.4226182617407));
#62888=DIRECTION('ref_axis',(0.,0.4226182617407,0.90630778703665));
#62889=DIRECTION('',(0.,-0.4226182617407,-0.90630778703665));
#62890=DIRECTION('',(1.,0.,0.));
#62891=DIRECTION('',(0.,0.4226182617407,0.90630778703665));
#62892=DIRECTION('',(-1.,0.,0.));
#62893=DIRECTION('center_axis',(0.,-0.90630778703665,0.4226182617407));
#62894=DIRECTION('ref_axis',(0.,-0.4226182617407,-0.90630778703665));
#62895=DIRECTION('',(1.,0.,0.));
#62896=DIRECTION('',(0.,-0.4226182617407,-0.90630778703665));
#62897=DIRECTION('',(1.,0.,0.));
#62898=DIRECTION('',(0.,0.4226182617407,0.90630778703665));
#62899=DIRECTION('center_axis',(0.,0.4226182617407,0.90630778703665));
#62900=DIRECTION('ref_axis',(0.,-0.906307787036649,0.4226182617407));
#62901=DIRECTION('',(0.,-0.906307787036649,0.4226182617407));
#62902=DIRECTION('',(0.,0.906307787036649,-0.4226182617407));
#62903=DIRECTION('center_axis',(1.,0.,0.));
#62904=DIRECTION('ref_axis',(0.,1.,0.));
#62905=DIRECTION('center_axis',(1.,0.,0.));
#62906=DIRECTION('ref_axis',(0.,0.,-1.));
#62907=DIRECTION('',(1.,0.,0.));
#62908=DIRECTION('center_axis',(1.,0.,0.));
#62909=DIRECTION('ref_axis',(0.,0.,-1.));
#62910=DIRECTION('center_axis',(-1.,0.,0.));
#62911=DIRECTION('ref_axis',(0.,-0.996194698091746,-0.0871557427476573));
#62912=DIRECTION('center_axis',(1.,0.,0.));
#62913=DIRECTION('ref_axis',(0.,0.,-1.));
#62914=DIRECTION('center_axis',(1.,0.,0.));
#62915=DIRECTION('ref_axis',(0.,0.,-1.));
#62916=DIRECTION('center_axis',(1.,0.,0.));
#62917=DIRECTION('ref_axis',(0.,0.,-1.));
#62918=DIRECTION('center_axis',(1.,0.,0.));
#62919=DIRECTION('ref_axis',(0.,0.,-1.));
#62920=DIRECTION('center_axis',(1.,0.,0.));
#62921=DIRECTION('ref_axis',(0.,0.,-1.));
#62922=DIRECTION('center_axis',(1.,0.,0.));
#62923=DIRECTION('ref_axis',(0.,0.,-1.));
#62924=DIRECTION('center_axis',(1.,0.,0.));
#62925=DIRECTION('ref_axis',(0.,0.,-1.));
#62926=DIRECTION('center_axis',(1.,0.,0.));
#62927=DIRECTION('ref_axis',(0.,0.,-1.));
#62928=DIRECTION('center_axis',(1.,0.,0.));
#62929=DIRECTION('ref_axis',(0.,0.,-1.));
#62930=DIRECTION('center_axis',(1.,0.,0.));
#62931=DIRECTION('ref_axis',(0.,0.,-1.));
#62932=DIRECTION('center_axis',(1.,0.,0.));
#62933=DIRECTION('ref_axis',(0.,0.,-1.));
#62934=DIRECTION('center_axis',(1.,0.,0.));
#62935=DIRECTION('ref_axis',(0.,0.,-1.));
#62936=DIRECTION('center_axis',(1.,0.,0.));
#62937=DIRECTION('ref_axis',(0.,0.,-1.));
#62938=DIRECTION('center_axis',(-1.,0.,0.));
#62939=DIRECTION('ref_axis',(0.,0.,1.));
#62940=DIRECTION('center_axis',(1.,0.,0.));
#62941=DIRECTION('ref_axis',(0.,0.,-1.));
#62942=DIRECTION('',(0.,0.573576436351046,-0.819152044288992));
#62943=DIRECTION('',(0.,0.819152044288992,0.573576436351046));
#62944=DIRECTION('',(0.,-0.573576436351046,0.819152044288992));
#62945=DIRECTION('center_axis',(1.,0.,0.));
#62946=DIRECTION('ref_axis',(0.,0.,-1.));
#62947=DIRECTION('',(0.,-0.996194698091746,-0.0871557427476583));
#62948=DIRECTION('',(0.,0.0871557427476578,-0.996194698091746));
#62949=DIRECTION('',(0.,0.996194698091746,0.0871557427476582));
#62950=DIRECTION('center_axis',(1.,0.,0.));
#62951=DIRECTION('ref_axis',(0.,0.,-1.));
#62952=DIRECTION('center_axis',(1.,0.,0.));
#62953=DIRECTION('ref_axis',(0.,0.,-1.));
#62954=DIRECTION('center_axis',(1.,0.,0.));
#62955=DIRECTION('ref_axis',(0.,-0.996194698091746,-0.0871557427476573));
#62956=DIRECTION('center_axis',(1.,0.,0.));
#62957=DIRECTION('ref_axis',(0.,0.,-1.));
#62958=DIRECTION('center_axis',(1.,0.,0.));
#62959=DIRECTION('ref_axis',(0.,0.,-1.));
#62960=DIRECTION('center_axis',(1.,0.,0.));
#62961=DIRECTION('ref_axis',(0.,0.,-1.));
#62962=DIRECTION('center_axis',(1.,0.,0.));
#62963=DIRECTION('ref_axis',(0.,0.,-1.));
#62964=DIRECTION('center_axis',(1.,0.,0.));
#62965=DIRECTION('ref_axis',(0.,0.,-1.));
#62966=DIRECTION('center_axis',(1.,0.,0.));
#62967=DIRECTION('ref_axis',(0.,0.,-1.));
#62968=DIRECTION('center_axis',(1.,0.,0.));
#62969=DIRECTION('ref_axis',(0.,0.,-1.));
#62970=DIRECTION('center_axis',(1.,0.,0.));
#62971=DIRECTION('ref_axis',(0.,0.,-1.));
#62972=DIRECTION('center_axis',(1.,0.,0.));
#62973=DIRECTION('ref_axis',(0.,0.,-1.));
#62974=DIRECTION('center_axis',(1.,0.,0.));
#62975=DIRECTION('ref_axis',(0.,0.,-1.));
#62976=DIRECTION('center_axis',(1.,0.,0.));
#62977=DIRECTION('ref_axis',(0.,0.,-1.));
#62978=DIRECTION('center_axis',(1.,0.,0.));
#62979=DIRECTION('ref_axis',(0.,0.,-1.));
#62980=DIRECTION('center_axis',(1.,0.,0.));
#62981=DIRECTION('ref_axis',(0.,1.,0.));
#62982=DIRECTION('center_axis',(1.,0.,0.));
#62983=DIRECTION('ref_axis',(0.,0.,-1.));
#62984=DIRECTION('center_axis',(1.,0.,0.));
#62985=DIRECTION('ref_axis',(0.,0.,-1.));
#62986=DIRECTION('center_axis',(1.,0.,0.));
#62987=DIRECTION('ref_axis',(0.,0.,-1.));
#62988=DIRECTION('center_axis',(1.,0.,0.));
#62989=DIRECTION('ref_axis',(0.,0.,-1.));
#62990=DIRECTION('center_axis',(1.,0.,0.));
#62991=DIRECTION('ref_axis',(0.,0.,-1.));
#62992=DIRECTION('center_axis',(1.,0.,0.));
#62993=DIRECTION('ref_axis',(0.,0.,-1.));
#62994=DIRECTION('center_axis',(1.,0.,0.));
#62995=DIRECTION('ref_axis',(0.,0.,-1.));
#62996=DIRECTION('center_axis',(1.,0.,0.));
#62997=DIRECTION('ref_axis',(0.,0.,-1.));
#62998=DIRECTION('center_axis',(1.,0.,0.));
#62999=DIRECTION('ref_axis',(0.,0.,-1.));
#63000=DIRECTION('center_axis',(1.,0.,0.));
#63001=DIRECTION('ref_axis',(0.,0.,-1.));
#63002=DIRECTION('center_axis',(1.,0.,0.));
#63003=DIRECTION('ref_axis',(0.,0.,-1.));
#63004=DIRECTION('center_axis',(0.,-0.819152044288992,-0.573576436351046));
#63005=DIRECTION('ref_axis',(0.,0.573576436351046,-0.819152044288992));
#63006=DIRECTION('',(0.,-0.573576436351046,0.819152044288992));
#63007=DIRECTION('',(1.,0.,0.));
#63008=DIRECTION('',(-1.,0.,0.));
#63009=DIRECTION('center_axis',(0.,0.819152044288992,0.573576436351046));
#63010=DIRECTION('ref_axis',(0.,-0.573576436351046,0.819152044288992));
#63011=DIRECTION('',(1.,0.,0.));
#63012=DIRECTION('',(1.,0.,0.));
#63013=DIRECTION('',(0.,0.573576436351046,-0.819152044288992));
#63014=DIRECTION('center_axis',(0.,0.573576436351046,-0.819152044288992));
#63015=DIRECTION('ref_axis',(0.,0.819152044288992,0.573576436351045));
#63016=DIRECTION('',(0.,-0.819152044288992,-0.573576436351046));
#63017=DIRECTION('center_axis',(-1.,0.,0.));
#63018=DIRECTION('ref_axis',(0.,1.,0.));
#63019=DIRECTION('center_axis',(1.,0.,0.));
#63020=DIRECTION('ref_axis',(0.,0.,-1.));
#63021=DIRECTION('center_axis',(1.,0.,0.));
#63022=DIRECTION('ref_axis',(0.,0.,-1.));
#63023=DIRECTION('center_axis',(1.,0.,0.));
#63024=DIRECTION('ref_axis',(0.,0.,-1.));
#63025=DIRECTION('center_axis',(1.,0.,0.));
#63026=DIRECTION('ref_axis',(0.,0.,-1.));
#63027=DIRECTION('center_axis',(1.,0.,0.));
#63028=DIRECTION('ref_axis',(0.,0.,-1.));
#63029=DIRECTION('center_axis',(1.,0.,0.));
#63030=DIRECTION('ref_axis',(0.,0.,-1.));
#63031=DIRECTION('center_axis',(1.,0.,0.));
#63032=DIRECTION('ref_axis',(0.,0.,-1.));
#63033=DIRECTION('center_axis',(1.,0.,0.));
#63034=DIRECTION('ref_axis',(0.,0.,-1.));
#63035=DIRECTION('center_axis',(1.,0.,0.));
#63036=DIRECTION('ref_axis',(0.,0.,-1.));
#63037=DIRECTION('center_axis',(1.,0.,0.));
#63038=DIRECTION('ref_axis',(0.,0.,-1.));
#63039=DIRECTION('center_axis',(1.,0.,0.));
#63040=DIRECTION('ref_axis',(0.,0.,-1.));
#63041=DIRECTION('center_axis',(1.,0.,0.));
#63042=DIRECTION('ref_axis',(0.,0.,-1.));
#63043=DIRECTION('center_axis',(1.,0.,0.));
#63044=DIRECTION('ref_axis',(0.,0.,-1.));
#63045=DIRECTION('center_axis',(-1.,0.,0.));
#63046=DIRECTION('ref_axis',(0.,1.,0.));
#63047=DIRECTION('center_axis',(1.,0.,0.));
#63048=DIRECTION('ref_axis',(0.,0.,-1.));
#63049=DIRECTION('center_axis',(1.,0.,0.));
#63050=DIRECTION('ref_axis',(0.,0.,-1.));
#63051=DIRECTION('center_axis',(1.,0.,0.));
#63052=DIRECTION('ref_axis',(0.,0.,-1.));
#63053=DIRECTION('center_axis',(1.,0.,0.));
#63054=DIRECTION('ref_axis',(0.,0.,-1.));
#63055=DIRECTION('center_axis',(1.,0.,0.));
#63056=DIRECTION('ref_axis',(0.,0.,-1.));
#63057=DIRECTION('center_axis',(1.,0.,0.));
#63058=DIRECTION('ref_axis',(0.,0.,-1.));
#63059=DIRECTION('center_axis',(1.,0.,0.));
#63060=DIRECTION('ref_axis',(0.,0.,-1.));
#63061=DIRECTION('center_axis',(1.,0.,0.));
#63062=DIRECTION('ref_axis',(0.,0.,-1.));
#63063=DIRECTION('center_axis',(1.,0.,0.));
#63064=DIRECTION('ref_axis',(0.,0.,-1.));
#63065=DIRECTION('center_axis',(1.,0.,0.));
#63066=DIRECTION('ref_axis',(0.,0.,-1.));
#63067=DIRECTION('center_axis',(1.,0.,0.));
#63068=DIRECTION('ref_axis',(0.,0.,-1.));
#63069=DIRECTION('center_axis',(1.,0.,0.));
#63070=DIRECTION('ref_axis',(0.,0.,-1.));
#63071=DIRECTION('center_axis',(1.,0.,0.));
#63072=DIRECTION('ref_axis',(0.,1.,0.));
#63073=DIRECTION('',(1.,0.,0.));
#63074=DIRECTION('center_axis',(1.,0.,0.));
#63075=DIRECTION('ref_axis',(0.,1.,0.));
#63076=DIRECTION('center_axis',(1.,0.,0.));
#63077=DIRECTION('ref_axis',(0.,0.,-1.));
#63078=DIRECTION('center_axis',(1.,0.,0.));
#63079=DIRECTION('ref_axis',(0.,0.,-1.));
#63080=DIRECTION('center_axis',(1.,0.,0.));
#63081=DIRECTION('ref_axis',(0.,0.,-1.));
#63082=DIRECTION('center_axis',(1.,0.,0.));
#63083=DIRECTION('ref_axis',(0.,0.,-1.));
#63084=DIRECTION('center_axis',(1.,0.,0.));
#63085=DIRECTION('ref_axis',(0.,0.,-1.));
#63086=DIRECTION('center_axis',(1.,0.,0.));
#63087=DIRECTION('ref_axis',(0.,0.,-1.));
#63088=DIRECTION('center_axis',(1.,0.,0.));
#63089=DIRECTION('ref_axis',(0.,0.,-1.));
#63090=DIRECTION('center_axis',(1.,0.,0.));
#63091=DIRECTION('ref_axis',(0.,0.,-1.));
#63092=DIRECTION('center_axis',(1.,0.,0.));
#63093=DIRECTION('ref_axis',(0.,0.,-1.));
#63094=DIRECTION('center_axis',(1.,0.,0.));
#63095=DIRECTION('ref_axis',(0.,0.,-1.));
#63096=DIRECTION('center_axis',(1.,0.,0.));
#63097=DIRECTION('ref_axis',(0.,0.,-1.));
#63098=DIRECTION('center_axis',(1.,0.,0.));
#63099=DIRECTION('ref_axis',(0.,0.,-1.));
#63100=DIRECTION('center_axis',(0.,-0.0871557427476583,0.996194698091746));
#63101=DIRECTION('ref_axis',(0.,-0.996194698091746,-0.0871557427476583));
#63102=DIRECTION('',(0.,0.996194698091746,0.0871557427476583));
#63103=DIRECTION('',(1.,0.,0.));
#63104=DIRECTION('',(-1.,0.,0.));
#63105=DIRECTION('center_axis',(0.,0.0871557427476582,-0.996194698091746));
#63106=DIRECTION('ref_axis',(0.,0.996194698091746,0.0871557427476582));
#63107=DIRECTION('',(1.,0.,0.));
#63108=DIRECTION('',(1.,0.,0.));
#63109=DIRECTION('',(0.,-0.996194698091746,-0.0871557427476582));
#63110=DIRECTION('center_axis',(0.,-0.996194698091746,-0.0871557427476578));
#63111=DIRECTION('ref_axis',(0.,0.0871557427476578,-0.996194698091746));
#63112=DIRECTION('',(0.,-0.0871557427476578,0.996194698091746));
#63113=DIRECTION('center_axis',(1.,0.,0.));
#63114=DIRECTION('ref_axis',(0.,1.,0.));
#63115=DIRECTION('',(1.,0.,0.));
#63116=DIRECTION('center_axis',(-1.,0.,0.));
#63117=DIRECTION('ref_axis',(0.,1.,0.));
#63118=DIRECTION('center_axis',(1.,0.,0.));
#63119=DIRECTION('ref_axis',(0.,1.,0.));
#63120=DIRECTION('center_axis',(-1.,0.,0.));
#63121=DIRECTION('ref_axis',(0.,1.,0.));
#63122=DIRECTION('center_axis',(1.,0.,0.));
#63123=DIRECTION('ref_axis',(0.,1.,0.));
#63124=DIRECTION('center_axis',(-1.,0.,0.));
#63125=DIRECTION('ref_axis',(0.,1.,0.));
#63126=DIRECTION('center_axis',(1.,0.,0.));
#63127=DIRECTION('ref_axis',(0.,1.,0.));
#63128=DIRECTION('center_axis',(-1.,0.,0.));
#63129=DIRECTION('ref_axis',(0.,1.,0.));
#63130=DIRECTION('center_axis',(1.,0.,0.));
#63131=DIRECTION('ref_axis',(0.,1.,0.));
#63132=DIRECTION('center_axis',(-1.,0.,0.));
#63133=DIRECTION('ref_axis',(0.,1.,0.));
#63134=DIRECTION('center_axis',(1.,0.,0.));
#63135=DIRECTION('ref_axis',(0.,1.,0.));
#63136=DIRECTION('center_axis',(-1.,0.,0.));
#63137=DIRECTION('ref_axis',(0.,1.,0.));
#63138=DIRECTION('center_axis',(1.,0.,0.));
#63139=DIRECTION('ref_axis',(0.,1.,0.));
#63140=DIRECTION('center_axis',(-1.,0.,0.));
#63141=DIRECTION('ref_axis',(0.,1.,0.));
#63142=DIRECTION('center_axis',(1.,0.,0.));
#63143=DIRECTION('ref_axis',(0.,1.,0.));
#63144=DIRECTION('center_axis',(-1.,0.,0.));
#63145=DIRECTION('ref_axis',(0.,1.,0.));
#63146=DIRECTION('center_axis',(1.,0.,0.));
#63147=DIRECTION('ref_axis',(0.,1.,0.));
#63148=DIRECTION('center_axis',(-1.,0.,0.));
#63149=DIRECTION('ref_axis',(0.,1.,0.));
#63150=DIRECTION('center_axis',(1.,0.,0.));
#63151=DIRECTION('ref_axis',(0.,1.,0.));
#63152=DIRECTION('center_axis',(-1.,0.,0.));
#63153=DIRECTION('ref_axis',(0.,1.,0.));
#63154=DIRECTION('center_axis',(1.,0.,0.));
#63155=DIRECTION('ref_axis',(0.,1.,0.));
#63156=DIRECTION('center_axis',(-1.,0.,0.));
#63157=DIRECTION('ref_axis',(0.,1.,0.));
#63158=DIRECTION('center_axis',(1.,0.,0.));
#63159=DIRECTION('ref_axis',(0.,1.,0.));
#63160=DIRECTION('center_axis',(-1.,0.,0.));
#63161=DIRECTION('ref_axis',(0.,1.,0.));
#63162=DIRECTION('center_axis',(1.,0.,0.));
#63163=DIRECTION('ref_axis',(0.,1.,0.));
#63164=DIRECTION('center_axis',(-1.,0.,0.));
#63165=DIRECTION('ref_axis',(0.,1.,0.));
#63166=DIRECTION('center_axis',(1.,0.,0.));
#63167=DIRECTION('ref_axis',(0.,1.,0.));
#63168=DIRECTION('center_axis',(-1.,0.,0.));
#63169=DIRECTION('ref_axis',(0.,1.,0.));
#63170=DIRECTION('center_axis',(1.,0.,0.));
#63171=DIRECTION('ref_axis',(0.,1.,0.));
#63172=DIRECTION('center_axis',(-1.,0.,0.));
#63173=DIRECTION('ref_axis',(0.,1.,0.));
#63174=DIRECTION('center_axis',(1.,0.,0.));
#63175=DIRECTION('ref_axis',(0.,1.,0.));
#63176=DIRECTION('center_axis',(-1.,0.,0.));
#63177=DIRECTION('ref_axis',(0.,1.,0.));
#63178=DIRECTION('center_axis',(1.,0.,0.));
#63179=DIRECTION('ref_axis',(0.,1.,0.));
#63180=DIRECTION('center_axis',(-1.,0.,0.));
#63181=DIRECTION('ref_axis',(0.,1.,0.));
#63182=DIRECTION('center_axis',(1.,0.,0.));
#63183=DIRECTION('ref_axis',(0.,1.,0.));
#63184=DIRECTION('center_axis',(-1.,0.,0.));
#63185=DIRECTION('ref_axis',(0.,1.,0.));
#63186=DIRECTION('center_axis',(1.,0.,0.));
#63187=DIRECTION('ref_axis',(0.,1.,0.));
#63188=DIRECTION('center_axis',(-1.,0.,0.));
#63189=DIRECTION('ref_axis',(0.,1.,0.));
#63190=DIRECTION('center_axis',(1.,0.,0.));
#63191=DIRECTION('ref_axis',(0.,1.,0.));
#63192=DIRECTION('center_axis',(-1.,0.,0.));
#63193=DIRECTION('ref_axis',(0.,1.,0.));
#63194=DIRECTION('center_axis',(1.,0.,0.));
#63195=DIRECTION('ref_axis',(0.,1.,0.));
#63196=DIRECTION('center_axis',(-1.,0.,0.));
#63197=DIRECTION('ref_axis',(0.,1.,0.));
#63198=DIRECTION('center_axis',(1.,0.,0.));
#63199=DIRECTION('ref_axis',(0.,1.,0.));
#63200=DIRECTION('center_axis',(-1.,0.,0.));
#63201=DIRECTION('ref_axis',(0.,1.,0.));
#63202=DIRECTION('center_axis',(1.,0.,0.));
#63203=DIRECTION('ref_axis',(0.,1.,0.));
#63204=DIRECTION('center_axis',(-1.,0.,0.));
#63205=DIRECTION('ref_axis',(0.,1.,0.));
#63206=DIRECTION('center_axis',(1.,0.,0.));
#63207=DIRECTION('ref_axis',(0.,1.,0.));
#63208=DIRECTION('center_axis',(-1.,0.,0.));
#63209=DIRECTION('ref_axis',(0.,1.,0.));
#63210=DIRECTION('center_axis',(1.,0.,0.));
#63211=DIRECTION('ref_axis',(0.,1.,0.));
#63212=DIRECTION('center_axis',(-1.,0.,0.));
#63213=DIRECTION('ref_axis',(0.,1.,0.));
#63214=DIRECTION('center_axis',(1.,0.,0.));
#63215=DIRECTION('ref_axis',(0.,1.,0.));
#63216=DIRECTION('center_axis',(-1.,0.,0.));
#63217=DIRECTION('ref_axis',(0.,1.,0.));
#63218=DIRECTION('center_axis',(1.,0.,0.));
#63219=DIRECTION('ref_axis',(0.,1.,0.));
#63220=DIRECTION('center_axis',(-1.,0.,0.));
#63221=DIRECTION('ref_axis',(0.,1.,0.));
#63222=DIRECTION('center_axis',(1.,0.,0.));
#63223=DIRECTION('ref_axis',(0.,1.,0.));
#63224=DIRECTION('center_axis',(-1.,0.,0.));
#63225=DIRECTION('ref_axis',(0.,1.,0.));
#63226=DIRECTION('center_axis',(1.,0.,0.));
#63227=DIRECTION('ref_axis',(0.,1.,0.));
#63228=DIRECTION('center_axis',(-1.,0.,0.));
#63229=DIRECTION('ref_axis',(0.,1.,0.));
#63230=DIRECTION('center_axis',(1.,0.,0.));
#63231=DIRECTION('ref_axis',(0.,1.,0.));
#63232=DIRECTION('center_axis',(-1.,0.,0.));
#63233=DIRECTION('ref_axis',(0.,1.,0.));
#63234=DIRECTION('center_axis',(1.,0.,0.));
#63235=DIRECTION('ref_axis',(0.,1.,0.));
#63236=DIRECTION('center_axis',(-1.,0.,0.));
#63237=DIRECTION('ref_axis',(0.,1.,0.));
#63238=DIRECTION('center_axis',(1.,0.,0.));
#63239=DIRECTION('ref_axis',(0.,1.,0.));
#63240=DIRECTION('center_axis',(-1.,0.,0.));
#63241=DIRECTION('ref_axis',(0.,1.,0.));
#63242=DIRECTION('center_axis',(1.,0.,0.));
#63243=DIRECTION('ref_axis',(0.,1.,0.));
#63244=DIRECTION('center_axis',(-1.,0.,0.));
#63245=DIRECTION('ref_axis',(0.,1.,0.));
#63246=DIRECTION('center_axis',(1.,0.,0.));
#63247=DIRECTION('ref_axis',(0.,1.,0.));
#63248=DIRECTION('center_axis',(0.,0.139173100960065,0.99026806874157));
#63249=DIRECTION('ref_axis',(0.,-0.99026806874157,0.139173100960065));
#63250=DIRECTION('',(1.,0.,0.));
#63251=DIRECTION('',(0.,-0.99026806874157,0.139173100960065));
#63252=DIRECTION('',(1.,0.,0.));
#63253=DIRECTION('',(-1.,0.,0.));
#63254=DIRECTION('',(1.,0.,0.));
#63255=DIRECTION('',(0.,-0.99026806874157,0.139173100960065));
#63256=DIRECTION('center_axis',(0.,0.996194698091746,-0.0871557427476593));
#63257=DIRECTION('ref_axis',(0.,0.0871557427476593,0.996194698091746));
#63258=DIRECTION('',(1.,0.,0.));
#63259=DIRECTION('center_axis',(0.,0.309016994374948,0.951056516295153));
#63260=DIRECTION('ref_axis',(0.,-0.951056516295153,0.309016994374948));
#63261=DIRECTION('',(1.,0.,0.));
#63262=DIRECTION('',(0.,-0.951056516295153,0.309016994374948));
#63263=DIRECTION('',(1.,0.,0.));
#63264=DIRECTION('',(-1.,0.,0.));
#63265=DIRECTION('',(1.,0.,0.));
#63266=DIRECTION('',(0.,-0.951056516295153,0.309016994374948));
#63267=DIRECTION('center_axis',(0.,0.965925826289068,-0.258819045102523));
#63268=DIRECTION('ref_axis',(0.,0.258819045102523,0.965925826289068));
#63269=DIRECTION('',(1.,0.,0.));
#63270=DIRECTION('center_axis',(0.,0.469471562785891,0.882947592858927));
#63271=DIRECTION('ref_axis',(0.,-0.882947592858927,0.469471562785891));
#63272=DIRECTION('',(1.,0.,0.));
#63273=DIRECTION('',(0.,-0.882947592858927,0.469471562785891));
#63274=DIRECTION('',(1.,0.,0.));
#63275=DIRECTION('',(-1.,0.,0.));
#63276=DIRECTION('',(1.,0.,0.));
#63277=DIRECTION('',(0.,-0.882947592858927,0.469471562785891));
#63278=DIRECTION('center_axis',(0.,0.906307787036649,-0.422618261740701));
#63279=DIRECTION('ref_axis',(0.,0.422618261740701,0.906307787036649));
#63280=DIRECTION('',(1.,0.,0.));
#63281=DIRECTION('center_axis',(0.,0.615661475325659,0.788010753606722));
#63282=DIRECTION('ref_axis',(0.,-0.788010753606722,0.615661475325659));
#63283=DIRECTION('',(1.,0.,0.));
#63284=DIRECTION('',(0.,-0.788010753606722,0.615661475325659));
#63285=DIRECTION('',(1.,0.,0.));
#63286=DIRECTION('',(-1.,0.,0.));
#63287=DIRECTION('',(1.,0.,0.));
#63288=DIRECTION('',(0.,-0.788010753606722,0.615661475325659));
#63289=DIRECTION('center_axis',(0.,0.819152044288991,-0.573576436351047));
#63290=DIRECTION('ref_axis',(0.,0.573576436351047,0.819152044288991));
#63291=DIRECTION('',(1.,0.,0.));
#63292=DIRECTION('center_axis',(0.,0.743144825477394,0.669130606358858));
#63293=DIRECTION('ref_axis',(0.,-0.669130606358858,0.743144825477394));
#63294=DIRECTION('',(1.,0.,0.));
#63295=DIRECTION('',(0.,-0.669130606358858,0.743144825477394));
#63296=DIRECTION('',(1.,0.,0.));
#63297=DIRECTION('',(-1.,0.,0.));
#63298=DIRECTION('',(1.,0.,0.));
#63299=DIRECTION('',(0.,-0.669130606358858,0.743144825477394));
#63300=DIRECTION('center_axis',(0.,0.707106781186547,-0.707106781186548));
#63301=DIRECTION('ref_axis',(0.,0.707106781186548,0.707106781186547));
#63302=DIRECTION('',(1.,0.,0.));
#63303=DIRECTION('center_axis',(0.,0.848048096156426,0.529919264233205));
#63304=DIRECTION('ref_axis',(0.,-0.529919264233205,0.848048096156426));
#63305=DIRECTION('',(1.,0.,0.));
#63306=DIRECTION('',(0.,-0.529919264233205,0.848048096156426));
#63307=DIRECTION('',(1.,0.,0.));
#63308=DIRECTION('',(-1.,0.,0.));
#63309=DIRECTION('',(1.,0.,0.));
#63310=DIRECTION('',(0.,-0.529919264233205,0.848048096156426));
#63311=DIRECTION('center_axis',(0.,0.573576436351045,-0.819152044288992));
#63312=DIRECTION('ref_axis',(0.,0.819152044288992,0.573576436351045));
#63313=DIRECTION('',(1.,0.,0.));
#63314=DIRECTION('center_axis',(0.,0.927183854566788,0.374606593415912));
#63315=DIRECTION('ref_axis',(0.,-0.374606593415912,0.927183854566788));
#63316=DIRECTION('',(1.,0.,0.));
#63317=DIRECTION('',(0.,-0.374606593415912,0.927183854566788));
#63318=DIRECTION('',(1.,0.,0.));
#63319=DIRECTION('',(-1.,0.,0.));
#63320=DIRECTION('',(1.,0.,0.));
#63321=DIRECTION('',(0.,-0.374606593415912,0.927183854566788));
#63322=DIRECTION('center_axis',(0.,0.422618261740698,-0.906307787036651));
#63323=DIRECTION('ref_axis',(0.,0.906307787036651,0.422618261740698));
#63324=DIRECTION('',(1.,0.,0.));
#63325=DIRECTION('center_axis',(0.,0.978147600733806,0.207911690817759));
#63326=DIRECTION('ref_axis',(0.,-0.207911690817759,0.978147600733806));
#63327=DIRECTION('',(1.,0.,0.));
#63328=DIRECTION('',(0.,-0.207911690817759,0.978147600733806));
#63329=DIRECTION('',(1.,0.,0.));
#63330=DIRECTION('',(-1.,0.,0.));
#63331=DIRECTION('',(1.,0.,0.));
#63332=DIRECTION('',(0.,-0.207911690817759,0.978147600733806));
#63333=DIRECTION('center_axis',(0.,0.258819045102519,-0.965925826289069));
#63334=DIRECTION('ref_axis',(0.,0.965925826289069,0.258819045102519));
#63335=DIRECTION('',(1.,0.,0.));
#63336=DIRECTION('center_axis',(0.,0.999390827019096,0.0348994967025009));
#63337=DIRECTION('ref_axis',(0.,-0.0348994967025009,0.999390827019096));
#63338=DIRECTION('',(1.,0.,0.));
#63339=DIRECTION('',(0.,-0.0348994967025009,0.999390827019096));
#63340=DIRECTION('',(1.,0.,0.));
#63341=DIRECTION('',(-1.,0.,0.));
#63342=DIRECTION('',(1.,0.,0.));
#63343=DIRECTION('',(0.,-0.0348994967025009,0.999390827019096));
#63344=DIRECTION('center_axis',(0.,0.0871557427476569,-0.996194698091746));
#63345=DIRECTION('ref_axis',(0.,0.996194698091746,0.0871557427476569));
#63346=DIRECTION('',(1.,0.,0.));
#63347=DIRECTION('center_axis',(0.,0.99026806874157,-0.139173100960065));
#63348=DIRECTION('ref_axis',(0.,0.139173100960065,0.99026806874157));
#63349=DIRECTION('',(1.,0.,0.));
#63350=DIRECTION('',(0.,0.139173100960065,0.99026806874157));
#63351=DIRECTION('',(1.,0.,0.));
#63352=DIRECTION('',(-1.,0.,0.));
#63353=DIRECTION('',(1.,0.,0.));
#63354=DIRECTION('',(0.,0.139173100960065,0.99026806874157));
#63355=DIRECTION('center_axis',(0.,-0.0871557427476592,-0.996194698091746));
#63356=DIRECTION('ref_axis',(0.,0.996194698091746,-0.0871557427476592));
#63357=DIRECTION('',(1.,0.,0.));
#63358=DIRECTION('center_axis',(0.,0.951056516295153,-0.309016994374948));
#63359=DIRECTION('ref_axis',(0.,0.309016994374948,0.951056516295153));
#63360=DIRECTION('',(1.,0.,0.));
#63361=DIRECTION('',(0.,0.309016994374948,0.951056516295153));
#63362=DIRECTION('',(1.,0.,0.));
#63363=DIRECTION('',(-1.,0.,0.));
#63364=DIRECTION('',(1.,0.,0.));
#63365=DIRECTION('',(0.,0.309016994374948,0.951056516295153));
#63366=DIRECTION('center_axis',(0.,-0.258819045102522,-0.965925826289068));
#63367=DIRECTION('ref_axis',(0.,0.965925826289068,-0.258819045102522));
#63368=DIRECTION('',(1.,0.,0.));
#63369=DIRECTION('center_axis',(0.,0.788010753606722,-0.615661475325658));
#63370=DIRECTION('ref_axis',(0.,0.615661475325658,0.788010753606722));
#63371=DIRECTION('',(1.,0.,0.));
#63372=DIRECTION('',(0.,0.615661475325658,0.788010753606722));
#63373=DIRECTION('',(1.,0.,0.));
#63374=DIRECTION('',(-1.,0.,0.));
#63375=DIRECTION('',(1.,0.,0.));
#63376=DIRECTION('',(0.,0.615661475325658,0.788010753606722));
#63377=DIRECTION('center_axis',(0.,-0.573576436351047,-0.819152044288991));
#63378=DIRECTION('ref_axis',(0.,0.819152044288991,-0.573576436351047));
#63379=DIRECTION('',(1.,0.,0.));
#63380=DIRECTION('center_axis',(0.,0.669130606358858,-0.743144825477394));
#63381=DIRECTION('ref_axis',(0.,0.743144825477394,0.669130606358858));
#63382=DIRECTION('',(1.,0.,0.));
#63383=DIRECTION('',(0.,0.743144825477394,0.669130606358858));
#63384=DIRECTION('',(1.,0.,0.));
#63385=DIRECTION('',(-1.,0.,0.));
#63386=DIRECTION('',(1.,0.,0.));
#63387=DIRECTION('',(0.,0.743144825477394,0.669130606358858));
#63388=DIRECTION('center_axis',(0.,-0.707106781186548,-0.707106781186547));
#63389=DIRECTION('ref_axis',(0.,0.707106781186547,-0.707106781186548));
#63390=DIRECTION('',(1.,0.,0.));
#63391=DIRECTION('center_axis',(0.,0.529919264233205,-0.848048096156426));
#63392=DIRECTION('ref_axis',(0.,0.848048096156426,0.529919264233205));
#63393=DIRECTION('',(1.,0.,0.));
#63394=DIRECTION('',(0.,0.848048096156426,0.529919264233205));
#63395=DIRECTION('',(1.,0.,0.));
#63396=DIRECTION('',(-1.,0.,0.));
#63397=DIRECTION('',(1.,0.,0.));
#63398=DIRECTION('',(0.,0.848048096156426,0.529919264233205));
#63399=DIRECTION('center_axis',(0.,-0.819152044288993,-0.573576436351045));
#63400=DIRECTION('ref_axis',(0.,0.573576436351045,-0.819152044288993));
#63401=DIRECTION('',(1.,0.,0.));
#63402=DIRECTION('center_axis',(0.,0.374606593415912,-0.927183854566787));
#63403=DIRECTION('ref_axis',(0.,0.927183854566787,0.374606593415912));
#63404=DIRECTION('',(1.,0.,0.));
#63405=DIRECTION('',(0.,0.927183854566787,0.374606593415912));
#63406=DIRECTION('',(1.,0.,0.));
#63407=DIRECTION('',(-1.,0.,0.));
#63408=DIRECTION('',(1.,0.,0.));
#63409=DIRECTION('',(0.,0.927183854566787,0.374606593415912));
#63410=DIRECTION('center_axis',(0.,-0.90630778703665,-0.422618261740698));
#63411=DIRECTION('ref_axis',(0.,0.422618261740698,-0.90630778703665));
#63412=DIRECTION('',(1.,0.,0.));
#63413=DIRECTION('center_axis',(0.,0.207911690817759,-0.978147600733806));
#63414=DIRECTION('ref_axis',(0.,0.978147600733806,0.207911690817759));
#63415=DIRECTION('',(1.,0.,0.));
#63416=DIRECTION('',(0.,0.978147600733806,0.207911690817759));
#63417=DIRECTION('',(1.,0.,0.));
#63418=DIRECTION('',(-1.,0.,0.));
#63419=DIRECTION('',(1.,0.,0.));
#63420=DIRECTION('',(0.,0.978147600733806,0.207911690817759));
#63421=DIRECTION('center_axis',(0.,-0.965925826289069,-0.258819045102519));
#63422=DIRECTION('ref_axis',(0.,0.258819045102519,-0.965925826289069));
#63423=DIRECTION('',(1.,0.,0.));
#63424=DIRECTION('center_axis',(0.,0.0348994967025009,-0.999390827019096));
#63425=DIRECTION('ref_axis',(0.,0.999390827019096,0.0348994967025009));
#63426=DIRECTION('',(1.,0.,0.));
#63427=DIRECTION('',(0.,0.999390827019096,0.0348994967025009));
#63428=DIRECTION('',(1.,0.,0.));
#63429=DIRECTION('',(-1.,0.,0.));
#63430=DIRECTION('',(1.,0.,0.));
#63431=DIRECTION('',(0.,0.999390827019096,0.0348994967025009));
#63432=DIRECTION('center_axis',(0.,-0.996194698091746,-0.087155742747657));
#63433=DIRECTION('ref_axis',(0.,0.087155742747657,-0.996194698091746));
#63434=DIRECTION('',(1.,0.,0.));
#63435=DIRECTION('center_axis',(0.,-0.139173100960066,-0.99026806874157));
#63436=DIRECTION('ref_axis',(0.,0.99026806874157,-0.139173100960066));
#63437=DIRECTION('',(1.,0.,0.));
#63438=DIRECTION('',(0.,0.99026806874157,-0.139173100960066));
#63439=DIRECTION('',(1.,0.,0.));
#63440=DIRECTION('',(-1.,0.,0.));
#63441=DIRECTION('',(1.,0.,0.));
#63442=DIRECTION('',(0.,0.99026806874157,-0.139173100960066));
#63443=DIRECTION('center_axis',(0.,-0.996194698091745,0.0871557427476596));
#63444=DIRECTION('ref_axis',(0.,-0.0871557427476596,-0.996194698091745));
#63445=DIRECTION('',(1.,0.,0.));
#63446=DIRECTION('center_axis',(0.,-0.309016994374948,-0.951056516295154));
#63447=DIRECTION('ref_axis',(0.,0.951056516295154,-0.309016994374948));
#63448=DIRECTION('',(1.,0.,0.));
#63449=DIRECTION('',(0.,0.951056516295154,-0.309016994374948));
#63450=DIRECTION('',(1.,0.,0.));
#63451=DIRECTION('',(-1.,0.,0.));
#63452=DIRECTION('',(1.,0.,0.));
#63453=DIRECTION('',(0.,0.951056516295154,-0.309016994374948));
#63454=DIRECTION('center_axis',(0.,-0.965925826289068,0.258819045102522));
#63455=DIRECTION('ref_axis',(0.,-0.258819045102522,-0.965925826289068));
#63456=DIRECTION('',(1.,0.,0.));
#63457=DIRECTION('center_axis',(0.,-0.469471562785891,-0.882947592858927));
#63458=DIRECTION('ref_axis',(0.,0.882947592858927,-0.469471562785891));
#63459=DIRECTION('',(1.,0.,0.));
#63460=DIRECTION('',(0.,0.882947592858927,-0.469471562785891));
#63461=DIRECTION('',(1.,0.,0.));
#63462=DIRECTION('',(-1.,0.,0.));
#63463=DIRECTION('',(1.,0.,0.));
#63464=DIRECTION('',(0.,0.882947592858927,-0.469471562785891));
#63465=DIRECTION('center_axis',(0.,-0.90630778703665,0.4226182617407));
#63466=DIRECTION('ref_axis',(0.,-0.4226182617407,-0.906307787036649));
#63467=DIRECTION('',(1.,0.,0.));
#63468=DIRECTION('center_axis',(0.,-0.615661475325658,-0.788010753606722));
#63469=DIRECTION('ref_axis',(0.,0.788010753606722,-0.615661475325658));
#63470=DIRECTION('',(1.,0.,0.));
#63471=DIRECTION('',(0.,0.788010753606722,-0.615661475325658));
#63472=DIRECTION('',(1.,0.,0.));
#63473=DIRECTION('',(-1.,0.,0.));
#63474=DIRECTION('',(1.,0.,0.));
#63475=DIRECTION('',(0.,0.788010753606722,-0.615661475325658));
#63476=DIRECTION('center_axis',(0.,-0.819152044288991,0.573576436351047));
#63477=DIRECTION('ref_axis',(0.,-0.573576436351047,-0.819152044288991));
#63478=DIRECTION('',(1.,0.,0.));
#63479=DIRECTION('center_axis',(0.,-0.743144825477394,-0.669130606358858));
#63480=DIRECTION('ref_axis',(0.,0.669130606358858,-0.743144825477394));
#63481=DIRECTION('',(1.,0.,0.));
#63482=DIRECTION('',(0.,0.669130606358858,-0.743144825477394));
#63483=DIRECTION('',(1.,0.,0.));
#63484=DIRECTION('',(-1.,0.,0.));
#63485=DIRECTION('',(1.,0.,0.));
#63486=DIRECTION('',(0.,0.669130606358858,-0.743144825477394));
#63487=DIRECTION('center_axis',(0.,-0.707106781186547,0.707106781186548));
#63488=DIRECTION('ref_axis',(0.,-0.707106781186548,-0.707106781186547));
#63489=DIRECTION('',(1.,0.,0.));
#63490=DIRECTION('center_axis',(0.,-0.927183854566787,-0.374606593415912));
#63491=DIRECTION('ref_axis',(0.,0.374606593415912,-0.927183854566787));
#63492=DIRECTION('',(1.,0.,0.));
#63493=DIRECTION('',(0.,0.374606593415912,-0.927183854566787));
#63494=DIRECTION('',(1.,0.,0.));
#63495=DIRECTION('',(-1.,0.,0.));
#63496=DIRECTION('',(1.,0.,0.));
#63497=DIRECTION('',(0.,0.374606593415912,-0.927183854566787));
#63498=DIRECTION('center_axis',(0.,-0.422618261740698,0.90630778703665));
#63499=DIRECTION('ref_axis',(0.,-0.90630778703665,-0.422618261740698));
#63500=DIRECTION('',(1.,0.,0.));
#63501=DIRECTION('center_axis',(0.,-0.978147600733806,-0.207911690817759));
#63502=DIRECTION('ref_axis',(0.,0.207911690817759,-0.978147600733806));
#63503=DIRECTION('',(1.,0.,0.));
#63504=DIRECTION('',(0.,0.207911690817759,-0.978147600733806));
#63505=DIRECTION('',(1.,0.,0.));
#63506=DIRECTION('',(-1.,0.,0.));
#63507=DIRECTION('',(1.,0.,0.));
#63508=DIRECTION('',(0.,0.207911690817759,-0.978147600733806));
#63509=DIRECTION('center_axis',(0.,-0.25881904510252,0.965925826289069));
#63510=DIRECTION('ref_axis',(0.,-0.965925826289069,-0.25881904510252));
#63511=DIRECTION('',(1.,0.,0.));
#63512=DIRECTION('center_axis',(0.,-0.999390827019096,-0.034899496702501));
#63513=DIRECTION('ref_axis',(0.,0.034899496702501,-0.999390827019096));
#63514=DIRECTION('',(1.,0.,0.));
#63515=DIRECTION('',(0.,0.034899496702501,-0.999390827019096));
#63516=DIRECTION('',(1.,0.,0.));
#63517=DIRECTION('',(-1.,0.,0.));
#63518=DIRECTION('',(1.,0.,0.));
#63519=DIRECTION('',(0.,0.034899496702501,-0.999390827019096));
#63520=DIRECTION('center_axis',(0.,-0.0871557427476571,0.996194698091746));
#63521=DIRECTION('ref_axis',(0.,-0.996194698091746,-0.0871557427476571));
#63522=DIRECTION('',(1.,0.,0.));
#63523=DIRECTION('center_axis',(0.,-0.99026806874157,0.139173100960065));
#63524=DIRECTION('ref_axis',(0.,-0.139173100960065,-0.99026806874157));
#63525=DIRECTION('',(1.,0.,0.));
#63526=DIRECTION('',(0.,-0.139173100960065,-0.99026806874157));
#63527=DIRECTION('',(1.,0.,0.));
#63528=DIRECTION('',(-1.,0.,0.));
#63529=DIRECTION('',(1.,0.,0.));
#63530=DIRECTION('',(0.,-0.139173100960065,-0.99026806874157));
#63531=DIRECTION('center_axis',(0.,0.0871557427476593,0.996194698091746));
#63532=DIRECTION('ref_axis',(0.,-0.996194698091746,0.0871557427476593));
#63533=DIRECTION('',(1.,0.,0.));
#63534=DIRECTION('center_axis',(0.,-0.951056516295154,0.309016994374948));
#63535=DIRECTION('ref_axis',(0.,-0.309016994374948,-0.951056516295154));
#63536=DIRECTION('',(1.,0.,0.));
#63537=DIRECTION('',(0.,-0.309016994374948,-0.951056516295154));
#63538=DIRECTION('',(1.,0.,0.));
#63539=DIRECTION('',(-1.,0.,0.));
#63540=DIRECTION('',(1.,0.,0.));
#63541=DIRECTION('',(0.,-0.309016994374948,-0.951056516295154));
#63542=DIRECTION('center_axis',(0.,0.258819045102522,0.965925826289068));
#63543=DIRECTION('ref_axis',(0.,-0.965925826289068,0.258819045102522));
#63544=DIRECTION('',(1.,0.,0.));
#63545=DIRECTION('center_axis',(0.,-0.882947592858927,0.469471562785891));
#63546=DIRECTION('ref_axis',(0.,-0.469471562785891,-0.882947592858927));
#63547=DIRECTION('',(1.,0.,0.));
#63548=DIRECTION('',(0.,-0.469471562785891,-0.882947592858927));
#63549=DIRECTION('',(1.,0.,0.));
#63550=DIRECTION('',(-1.,0.,0.));
#63551=DIRECTION('',(1.,0.,0.));
#63552=DIRECTION('',(0.,-0.469471562785891,-0.882947592858927));
#63553=DIRECTION('center_axis',(0.,0.422618261740701,0.906307787036649));
#63554=DIRECTION('ref_axis',(0.,-0.906307787036649,0.4226182617407));
#63555=DIRECTION('',(1.,0.,0.));
#63556=DIRECTION('center_axis',(0.,-0.788010753606722,0.615661475325658));
#63557=DIRECTION('ref_axis',(0.,-0.615661475325658,-0.788010753606722));
#63558=DIRECTION('',(1.,0.,0.));
#63559=DIRECTION('',(0.,-0.615661475325658,-0.788010753606722));
#63560=DIRECTION('',(1.,0.,0.));
#63561=DIRECTION('',(-1.,0.,0.));
#63562=DIRECTION('',(1.,0.,0.));
#63563=DIRECTION('',(0.,-0.615661475325658,-0.788010753606722));
#63564=DIRECTION('center_axis',(0.,0.573576436351047,0.819152044288991));
#63565=DIRECTION('ref_axis',(0.,-0.819152044288991,0.573576436351047));
#63566=DIRECTION('',(1.,0.,0.));
#63567=DIRECTION('center_axis',(0.,-0.669130606358858,0.743144825477394));
#63568=DIRECTION('ref_axis',(0.,-0.743144825477394,-0.669130606358858));
#63569=DIRECTION('',(1.,0.,0.));
#63570=DIRECTION('',(0.,-0.743144825477394,-0.669130606358858));
#63571=DIRECTION('',(1.,0.,0.));
#63572=DIRECTION('',(-1.,0.,0.));
#63573=DIRECTION('',(1.,0.,0.));
#63574=DIRECTION('',(0.,-0.743144825477394,-0.669130606358858));
#63575=DIRECTION('center_axis',(0.,0.707106781186548,0.707106781186547));
#63576=DIRECTION('ref_axis',(0.,-0.707106781186547,0.707106781186548));
#63577=DIRECTION('',(1.,0.,0.));
#63578=DIRECTION('center_axis',(0.,-0.529919264233205,0.848048096156426));
#63579=DIRECTION('ref_axis',(0.,-0.848048096156426,-0.529919264233205));
#63580=DIRECTION('',(1.,0.,0.));
#63581=DIRECTION('',(0.,-0.848048096156426,-0.529919264233205));
#63582=DIRECTION('',(1.,0.,0.));
#63583=DIRECTION('',(-1.,0.,0.));
#63584=DIRECTION('',(1.,0.,0.));
#63585=DIRECTION('',(0.,-0.848048096156426,-0.529919264233205));
#63586=DIRECTION('center_axis',(0.,0.819152044288993,0.573576436351045));
#63587=DIRECTION('ref_axis',(0.,-0.573576436351045,0.819152044288992));
#63588=DIRECTION('',(1.,0.,0.));
#63589=DIRECTION('center_axis',(0.,-0.374606593415912,0.927183854566787));
#63590=DIRECTION('ref_axis',(0.,-0.927183854566787,-0.374606593415912));
#63591=DIRECTION('',(1.,0.,0.));
#63592=DIRECTION('',(0.,-0.927183854566787,-0.374606593415912));
#63593=DIRECTION('',(1.,0.,0.));
#63594=DIRECTION('',(-1.,0.,0.));
#63595=DIRECTION('',(1.,0.,0.));
#63596=DIRECTION('',(0.,-0.927183854566787,-0.374606593415912));
#63597=DIRECTION('center_axis',(0.,0.90630778703665,0.422618261740698));
#63598=DIRECTION('ref_axis',(0.,-0.422618261740698,0.90630778703665));
#63599=DIRECTION('',(1.,0.,0.));
#63600=DIRECTION('center_axis',(0.,-0.207911690817759,0.978147600733806));
#63601=DIRECTION('ref_axis',(0.,-0.978147600733806,-0.207911690817759));
#63602=DIRECTION('',(1.,0.,0.));
#63603=DIRECTION('',(0.,-0.978147600733806,-0.207911690817759));
#63604=DIRECTION('',(1.,0.,0.));
#63605=DIRECTION('',(-1.,0.,0.));
#63606=DIRECTION('',(1.,0.,0.));
#63607=DIRECTION('',(0.,-0.978147600733806,-0.207911690817759));
#63608=DIRECTION('center_axis',(0.,0.965925826289069,0.25881904510252));
#63609=DIRECTION('ref_axis',(0.,-0.25881904510252,0.965925826289069));
#63610=DIRECTION('',(1.,0.,0.));
#63611=DIRECTION('center_axis',(1.,0.,0.));
#63612=DIRECTION('ref_axis',(0.,1.,0.));
#63613=DIRECTION('center_axis',(-1.,0.,0.));
#63614=DIRECTION('ref_axis',(0.,1.,0.));
#63615=DIRECTION('center_axis',(1.,0.,0.));
#63616=DIRECTION('ref_axis',(0.,1.,0.));
#63617=DIRECTION('center_axis',(-1.,0.,0.));
#63618=DIRECTION('ref_axis',(0.,1.,0.));
#63619=DIRECTION('center_axis',(1.,0.,0.));
#63620=DIRECTION('ref_axis',(0.,1.,0.));
#63621=DIRECTION('center_axis',(-1.,0.,0.));
#63622=DIRECTION('ref_axis',(0.,1.,0.));
#63623=DIRECTION('center_axis',(1.,0.,0.));
#63624=DIRECTION('ref_axis',(0.,1.,0.));
#63625=DIRECTION('center_axis',(-1.,0.,0.));
#63626=DIRECTION('ref_axis',(0.,1.,0.));
#63627=DIRECTION('center_axis',(1.,0.,0.));
#63628=DIRECTION('ref_axis',(0.,1.,0.));
#63629=DIRECTION('center_axis',(-1.,0.,0.));
#63630=DIRECTION('ref_axis',(0.,1.,0.));
#63631=DIRECTION('center_axis',(1.,0.,0.));
#63632=DIRECTION('ref_axis',(0.,1.,0.));
#63633=DIRECTION('center_axis',(-1.,0.,0.));
#63634=DIRECTION('ref_axis',(0.,1.,0.));
#63635=DIRECTION('center_axis',(1.,0.,0.));
#63636=DIRECTION('ref_axis',(0.,1.,0.));
#63637=DIRECTION('center_axis',(-1.,0.,0.));
#63638=DIRECTION('ref_axis',(0.,1.,0.));
#63639=DIRECTION('center_axis',(1.,0.,0.));
#63640=DIRECTION('ref_axis',(0.,1.,0.));
#63641=DIRECTION('center_axis',(-1.,0.,0.));
#63642=DIRECTION('ref_axis',(0.,1.,0.));
#63643=DIRECTION('center_axis',(1.,0.,0.));
#63644=DIRECTION('ref_axis',(0.,1.,0.));
#63645=DIRECTION('center_axis',(-1.,0.,0.));
#63646=DIRECTION('ref_axis',(0.,1.,0.));
#63647=DIRECTION('center_axis',(1.,0.,0.));
#63648=DIRECTION('ref_axis',(0.,1.,0.));
#63649=DIRECTION('center_axis',(-1.,0.,0.));
#63650=DIRECTION('ref_axis',(0.,1.,0.));
#63651=DIRECTION('center_axis',(1.,0.,0.));
#63652=DIRECTION('ref_axis',(0.,1.,0.));
#63653=DIRECTION('center_axis',(-1.,0.,0.));
#63654=DIRECTION('ref_axis',(0.,1.,0.));
#63655=DIRECTION('center_axis',(1.,0.,0.));
#63656=DIRECTION('ref_axis',(0.,1.,0.));
#63657=DIRECTION('center_axis',(-1.,0.,0.));
#63658=DIRECTION('ref_axis',(0.,1.,0.));
#63659=DIRECTION('center_axis',(1.,0.,0.));
#63660=DIRECTION('ref_axis',(0.,1.,0.));
#63661=DIRECTION('center_axis',(-1.,0.,0.));
#63662=DIRECTION('ref_axis',(0.,1.,0.));
#63663=DIRECTION('center_axis',(1.,0.,0.));
#63664=DIRECTION('ref_axis',(0.,1.,0.));
#63665=DIRECTION('center_axis',(-1.,0.,0.));
#63666=DIRECTION('ref_axis',(0.,1.,0.));
#63667=DIRECTION('center_axis',(1.,0.,0.));
#63668=DIRECTION('ref_axis',(0.,1.,0.));
#63669=DIRECTION('center_axis',(-1.,0.,0.));
#63670=DIRECTION('ref_axis',(0.,1.,0.));
#63671=DIRECTION('center_axis',(1.,0.,0.));
#63672=DIRECTION('ref_axis',(0.,1.,0.));
#63673=DIRECTION('center_axis',(-1.,0.,0.));
#63674=DIRECTION('ref_axis',(0.,1.,0.));
#63675=DIRECTION('center_axis',(1.,0.,0.));
#63676=DIRECTION('ref_axis',(0.,1.,0.));
#63677=DIRECTION('center_axis',(-1.,0.,0.));
#63678=DIRECTION('ref_axis',(0.,1.,0.));
#63679=DIRECTION('center_axis',(1.,0.,0.));
#63680=DIRECTION('ref_axis',(0.,1.,0.));
#63681=DIRECTION('center_axis',(-1.,0.,0.));
#63682=DIRECTION('ref_axis',(0.,1.,0.));
#63683=DIRECTION('center_axis',(1.,0.,0.));
#63684=DIRECTION('ref_axis',(0.,1.,0.));
#63685=DIRECTION('center_axis',(-1.,0.,0.));
#63686=DIRECTION('ref_axis',(0.,1.,0.));
#63687=DIRECTION('center_axis',(1.,0.,0.));
#63688=DIRECTION('ref_axis',(0.,1.,0.));
#63689=DIRECTION('center_axis',(-1.,0.,0.));
#63690=DIRECTION('ref_axis',(0.,1.,0.));
#63691=DIRECTION('center_axis',(1.,0.,0.));
#63692=DIRECTION('ref_axis',(0.,1.,0.));
#63693=DIRECTION('center_axis',(-1.,0.,0.));
#63694=DIRECTION('ref_axis',(0.,1.,0.));
#63695=DIRECTION('center_axis',(1.,0.,0.));
#63696=DIRECTION('ref_axis',(0.,1.,0.));
#63697=DIRECTION('center_axis',(-1.,0.,0.));
#63698=DIRECTION('ref_axis',(0.,1.,0.));
#63699=DIRECTION('center_axis',(1.,0.,0.));
#63700=DIRECTION('ref_axis',(0.,1.,0.));
#63701=DIRECTION('center_axis',(-1.,0.,0.));
#63702=DIRECTION('ref_axis',(0.,1.,0.));
#63703=DIRECTION('center_axis',(1.,0.,0.));
#63704=DIRECTION('ref_axis',(0.,1.,0.));
#63705=DIRECTION('center_axis',(-1.,0.,0.));
#63706=DIRECTION('ref_axis',(0.,1.,0.));
#63707=DIRECTION('center_axis',(1.,0.,0.));
#63708=DIRECTION('ref_axis',(0.,1.,0.));
#63709=DIRECTION('center_axis',(-1.,0.,0.));
#63710=DIRECTION('ref_axis',(0.,1.,0.));
#63711=DIRECTION('center_axis',(1.,0.,0.));
#63712=DIRECTION('ref_axis',(0.,1.,0.));
#63713=DIRECTION('center_axis',(-1.,0.,0.));
#63714=DIRECTION('ref_axis',(0.,1.,0.));
#63715=DIRECTION('center_axis',(1.,0.,0.));
#63716=DIRECTION('ref_axis',(0.,1.,0.));
#63717=DIRECTION('center_axis',(-1.,0.,0.));
#63718=DIRECTION('ref_axis',(0.,1.,0.));
#63719=DIRECTION('center_axis',(1.,0.,0.));
#63720=DIRECTION('ref_axis',(0.,1.,0.));
#63721=DIRECTION('center_axis',(-1.,0.,0.));
#63722=DIRECTION('ref_axis',(0.,1.,0.));
#63723=DIRECTION('center_axis',(1.,0.,0.));
#63724=DIRECTION('ref_axis',(0.,1.,0.));
#63725=DIRECTION('center_axis',(-1.,0.,0.));
#63726=DIRECTION('ref_axis',(0.,1.,0.));
#63727=DIRECTION('center_axis',(1.,0.,0.));
#63728=DIRECTION('ref_axis',(0.,1.,0.));
#63729=DIRECTION('center_axis',(-1.,0.,0.));
#63730=DIRECTION('ref_axis',(0.,1.,0.));
#63731=DIRECTION('center_axis',(1.,0.,0.));
#63732=DIRECTION('ref_axis',(0.,1.,0.));
#63733=DIRECTION('center_axis',(-1.,0.,0.));
#63734=DIRECTION('ref_axis',(0.,1.,0.));
#63735=DIRECTION('center_axis',(1.,0.,0.));
#63736=DIRECTION('ref_axis',(0.,1.,0.));
#63737=DIRECTION('center_axis',(-1.,0.,0.));
#63738=DIRECTION('ref_axis',(0.,1.,0.));
#63739=DIRECTION('center_axis',(1.,0.,0.));
#63740=DIRECTION('ref_axis',(0.,1.,0.));
#63741=DIRECTION('center_axis',(-1.,0.,0.));
#63742=DIRECTION('ref_axis',(0.,1.,0.));
#63743=DIRECTION('center_axis',(0.,-0.0348994967025009,-0.999390827019096));
#63744=DIRECTION('ref_axis',(0.,0.999390827019096,-0.0348994967025009));
#63745=DIRECTION('',(0.,0.999390827019096,-0.0348994967025009));
#63746=DIRECTION('',(1.,0.,0.));
#63747=DIRECTION('',(1.,0.,0.));
#63748=DIRECTION('',(1.,0.,0.));
#63749=DIRECTION('',(0.,0.999390827019096,-0.0348994967025009));
#63750=DIRECTION('center_axis',(0.,-0.20791169081776,-0.978147600733805));
#63751=DIRECTION('ref_axis',(0.,0.978147600733805,-0.20791169081776));
#63752=DIRECTION('',(0.,0.978147600733805,-0.20791169081776));
#63753=DIRECTION('',(1.,0.,0.));
#63754=DIRECTION('',(1.,0.,0.));
#63755=DIRECTION('',(1.,0.,0.));
#63756=DIRECTION('',(0.,0.978147600733805,-0.20791169081776));
#63757=DIRECTION('center_axis',(0.,-0.374606593415912,-0.927183854566787));
#63758=DIRECTION('ref_axis',(0.,0.927183854566787,-0.374606593415912));
#63759=DIRECTION('',(0.,0.927183854566787,-0.374606593415912));
#63760=DIRECTION('',(1.,0.,0.));
#63761=DIRECTION('',(1.,0.,0.));
#63762=DIRECTION('',(1.,0.,0.));
#63763=DIRECTION('',(0.,0.927183854566787,-0.374606593415912));
#63764=DIRECTION('center_axis',(0.,-0.529919264233205,-0.848048096156426));
#63765=DIRECTION('ref_axis',(0.,0.848048096156426,-0.529919264233205));
#63766=DIRECTION('',(0.,0.848048096156426,-0.529919264233205));
#63767=DIRECTION('',(1.,0.,0.));
#63768=DIRECTION('',(1.,0.,0.));
#63769=DIRECTION('',(1.,0.,0.));
#63770=DIRECTION('',(0.,0.848048096156426,-0.529919264233205));
#63771=DIRECTION('center_axis',(0.,-0.669130606358858,-0.743144825477394));
#63772=DIRECTION('ref_axis',(0.,0.743144825477394,-0.669130606358858));
#63773=DIRECTION('',(0.,0.743144825477394,-0.669130606358858));
#63774=DIRECTION('',(1.,0.,0.));
#63775=DIRECTION('',(1.,0.,0.));
#63776=DIRECTION('',(1.,0.,0.));
#63777=DIRECTION('',(0.,0.743144825477394,-0.669130606358858));
#63778=DIRECTION('center_axis',(0.,-0.788010753606722,-0.615661475325659));
#63779=DIRECTION('ref_axis',(0.,0.615661475325658,-0.788010753606722));
#63780=DIRECTION('',(0.,0.615661475325658,-0.788010753606722));
#63781=DIRECTION('',(1.,0.,0.));
#63782=DIRECTION('',(1.,0.,0.));
#63783=DIRECTION('',(1.,0.,0.));
#63784=DIRECTION('',(0.,0.615661475325658,-0.788010753606722));
#63785=DIRECTION('center_axis',(0.,-0.882947592858927,-0.46947156278589));
#63786=DIRECTION('ref_axis',(0.,0.46947156278589,-0.882947592858927));
#63787=DIRECTION('',(0.,0.46947156278589,-0.882947592858927));
#63788=DIRECTION('',(1.,0.,0.));
#63789=DIRECTION('',(1.,0.,0.));
#63790=DIRECTION('',(1.,0.,0.));
#63791=DIRECTION('',(0.,0.46947156278589,-0.882947592858927));
#63792=DIRECTION('center_axis',(0.,-0.951056516295154,-0.309016994374947));
#63793=DIRECTION('ref_axis',(0.,0.309016994374947,-0.951056516295154));
#63794=DIRECTION('',(0.,0.309016994374947,-0.951056516295154));
#63795=DIRECTION('',(1.,0.,0.));
#63796=DIRECTION('',(1.,0.,0.));
#63797=DIRECTION('',(1.,0.,0.));
#63798=DIRECTION('',(0.,0.309016994374947,-0.951056516295154));
#63799=DIRECTION('center_axis',(0.,-0.99026806874157,-0.139173100960065));
#63800=DIRECTION('ref_axis',(0.,0.139173100960065,-0.99026806874157));
#63801=DIRECTION('',(0.,0.139173100960065,-0.99026806874157));
#63802=DIRECTION('',(1.,0.,0.));
#63803=DIRECTION('',(1.,0.,0.));
#63804=DIRECTION('',(1.,0.,0.));
#63805=DIRECTION('',(0.,0.139173100960065,-0.99026806874157));
#63806=DIRECTION('center_axis',(0.,-0.999390827019096,0.0348994967025009));
#63807=DIRECTION('ref_axis',(0.,-0.0348994967025009,-0.999390827019096));
#63808=DIRECTION('',(0.,-0.0348994967025009,-0.999390827019096));
#63809=DIRECTION('',(1.,0.,0.));
#63810=DIRECTION('',(1.,0.,0.));
#63811=DIRECTION('',(1.,0.,0.));
#63812=DIRECTION('',(0.,-0.0348994967025009,-0.999390827019096));
#63813=DIRECTION('center_axis',(0.,-0.978147600733806,0.20791169081776));
#63814=DIRECTION('ref_axis',(0.,-0.20791169081776,-0.978147600733805));
#63815=DIRECTION('',(0.,-0.20791169081776,-0.978147600733805));
#63816=DIRECTION('',(1.,0.,0.));
#63817=DIRECTION('',(1.,0.,0.));
#63818=DIRECTION('',(0.,-0.20791169081776,-0.978147600733805));
#63819=DIRECTION('center_axis',(0.,-0.848048096156426,0.529919264233205));
#63820=DIRECTION('ref_axis',(0.,-0.529919264233205,-0.848048096156426));
#63821=DIRECTION('',(0.,-0.529919264233205,-0.848048096156426));
#63822=DIRECTION('',(1.,0.,0.));
#63823=DIRECTION('',(1.,0.,0.));
#63824=DIRECTION('',(1.,0.,0.));
#63825=DIRECTION('',(0.,-0.529919264233205,-0.848048096156426));
#63826=DIRECTION('center_axis',(0.,-0.743144825477394,0.669130606358858));
#63827=DIRECTION('ref_axis',(0.,-0.669130606358858,-0.743144825477394));
#63828=DIRECTION('',(0.,-0.669130606358858,-0.743144825477394));
#63829=DIRECTION('',(1.,0.,0.));
#63830=DIRECTION('',(1.,0.,0.));
#63831=DIRECTION('',(1.,0.,0.));
#63832=DIRECTION('',(0.,-0.669130606358858,-0.743144825477394));
#63833=DIRECTION('center_axis',(0.,-0.615661475325658,0.788010753606722));
#63834=DIRECTION('ref_axis',(0.,-0.788010753606722,-0.615661475325658));
#63835=DIRECTION('',(0.,-0.788010753606722,-0.615661475325658));
#63836=DIRECTION('',(1.,0.,0.));
#63837=DIRECTION('',(1.,0.,0.));
#63838=DIRECTION('',(1.,0.,0.));
#63839=DIRECTION('',(0.,-0.788010753606722,-0.615661475325658));
#63840=DIRECTION('center_axis',(0.,-0.469471562785891,0.882947592858927));
#63841=DIRECTION('ref_axis',(0.,-0.882947592858927,-0.469471562785891));
#63842=DIRECTION('',(0.,-0.882947592858927,-0.469471562785891));
#63843=DIRECTION('',(1.,0.,0.));
#63844=DIRECTION('',(1.,0.,0.));
#63845=DIRECTION('',(1.,0.,0.));
#63846=DIRECTION('',(0.,-0.882947592858927,-0.469471562785891));
#63847=DIRECTION('center_axis',(0.,-0.309016994374947,0.951056516295154));
#63848=DIRECTION('ref_axis',(0.,-0.951056516295154,-0.309016994374947));
#63849=DIRECTION('',(0.,-0.951056516295154,-0.309016994374947));
#63850=DIRECTION('',(1.,0.,0.));
#63851=DIRECTION('',(1.,0.,0.));
#63852=DIRECTION('',(1.,0.,0.));
#63853=DIRECTION('',(0.,-0.951056516295154,-0.309016994374947));
#63854=DIRECTION('center_axis',(0.,-0.139173100960065,0.99026806874157));
#63855=DIRECTION('ref_axis',(0.,-0.99026806874157,-0.139173100960065));
#63856=DIRECTION('',(0.,-0.99026806874157,-0.139173100960065));
#63857=DIRECTION('',(1.,0.,0.));
#63858=DIRECTION('',(1.,0.,0.));
#63859=DIRECTION('',(1.,0.,0.));
#63860=DIRECTION('',(0.,-0.99026806874157,-0.139173100960065));
#63861=DIRECTION('center_axis',(0.,0.0348994967025012,0.999390827019096));
#63862=DIRECTION('ref_axis',(0.,-0.999390827019096,0.0348994967025012));
#63863=DIRECTION('',(0.,-0.999390827019096,0.0348994967025012));
#63864=DIRECTION('',(1.,0.,0.));
#63865=DIRECTION('',(1.,0.,0.));
#63866=DIRECTION('',(1.,0.,0.));
#63867=DIRECTION('',(0.,-0.999390827019096,0.0348994967025012));
#63868=DIRECTION('center_axis',(0.,0.207911690817759,0.978147600733806));
#63869=DIRECTION('ref_axis',(0.,-0.978147600733806,0.207911690817759));
#63870=DIRECTION('',(0.,-0.978147600733806,0.207911690817759));
#63871=DIRECTION('',(1.,0.,0.));
#63872=DIRECTION('',(1.,0.,0.));
#63873=DIRECTION('',(1.,0.,0.));
#63874=DIRECTION('',(0.,-0.978147600733806,0.207911690817759));
#63875=DIRECTION('center_axis',(0.,0.374606593415912,0.927183854566788));
#63876=DIRECTION('ref_axis',(0.,-0.927183854566787,0.374606593415912));
#63877=DIRECTION('',(0.,-0.927183854566787,0.374606593415912));
#63878=DIRECTION('',(1.,0.,0.));
#63879=DIRECTION('',(1.,0.,0.));
#63880=DIRECTION('',(1.,0.,0.));
#63881=DIRECTION('',(0.,-0.927183854566787,0.374606593415912));
#63882=DIRECTION('center_axis',(0.,0.529919264233205,0.848048096156426));
#63883=DIRECTION('ref_axis',(0.,-0.848048096156426,0.529919264233205));
#63884=DIRECTION('',(0.,-0.848048096156426,0.529919264233205));
#63885=DIRECTION('',(1.,0.,0.));
#63886=DIRECTION('',(1.,0.,0.));
#63887=DIRECTION('',(1.,0.,0.));
#63888=DIRECTION('',(0.,-0.848048096156426,0.529919264233205));
#63889=DIRECTION('center_axis',(0.,0.669130606358858,0.743144825477394));
#63890=DIRECTION('ref_axis',(0.,-0.743144825477394,0.669130606358858));
#63891=DIRECTION('',(0.,-0.743144825477394,0.669130606358858));
#63892=DIRECTION('',(1.,0.,0.));
#63893=DIRECTION('',(1.,0.,0.));
#63894=DIRECTION('',(0.,-0.743144825477394,0.669130606358858));
#63895=DIRECTION('center_axis',(0.,0.882947592858927,0.469471562785891));
#63896=DIRECTION('ref_axis',(0.,-0.469471562785891,0.882947592858927));
#63897=DIRECTION('',(0.,-0.469471562785891,0.882947592858927));
#63898=DIRECTION('',(1.,0.,0.));
#63899=DIRECTION('',(1.,0.,0.));
#63900=DIRECTION('',(1.,0.,0.));
#63901=DIRECTION('',(0.,-0.469471562785891,0.882947592858927));
#63902=DIRECTION('center_axis',(0.,0.951056516295154,0.309016994374948));
#63903=DIRECTION('ref_axis',(0.,-0.309016994374948,0.951056516295154));
#63904=DIRECTION('',(0.,-0.309016994374948,0.951056516295154));
#63905=DIRECTION('',(1.,0.,0.));
#63906=DIRECTION('',(1.,0.,0.));
#63907=DIRECTION('',(1.,0.,0.));
#63908=DIRECTION('',(0.,-0.309016994374948,0.951056516295154));
#63909=DIRECTION('center_axis',(0.,0.99026806874157,0.139173100960065));
#63910=DIRECTION('ref_axis',(0.,-0.139173100960065,0.99026806874157));
#63911=DIRECTION('',(0.,-0.139173100960065,0.99026806874157));
#63912=DIRECTION('',(1.,0.,0.));
#63913=DIRECTION('',(1.,0.,0.));
#63914=DIRECTION('',(1.,0.,0.));
#63915=DIRECTION('',(0.,-0.139173100960065,0.99026806874157));
#63916=DIRECTION('center_axis',(0.,0.999390827019096,-0.0348994967025009));
#63917=DIRECTION('ref_axis',(0.,0.0348994967025009,0.999390827019096));
#63918=DIRECTION('',(0.,0.0348994967025009,0.999390827019096));
#63919=DIRECTION('',(1.,0.,0.));
#63920=DIRECTION('',(1.,0.,0.));
#63921=DIRECTION('',(1.,0.,0.));
#63922=DIRECTION('',(0.,0.0348994967025009,0.999390827019096));
#63923=DIRECTION('center_axis',(0.,0.978147600733806,-0.207911690817759));
#63924=DIRECTION('ref_axis',(0.,0.207911690817759,0.978147600733806));
#63925=DIRECTION('',(0.,0.207911690817759,0.978147600733806));
#63926=DIRECTION('',(1.,0.,0.));
#63927=DIRECTION('',(1.,0.,0.));
#63928=DIRECTION('',(1.,0.,0.));
#63929=DIRECTION('',(0.,0.207911690817759,0.978147600733806));
#63930=DIRECTION('center_axis',(0.,0.927183854566787,-0.374606593415912));
#63931=DIRECTION('ref_axis',(0.,0.374606593415912,0.927183854566787));
#63932=DIRECTION('',(0.,0.374606593415912,0.927183854566787));
#63933=DIRECTION('',(1.,0.,0.));
#63934=DIRECTION('',(1.,0.,0.));
#63935=DIRECTION('',(1.,0.,0.));
#63936=DIRECTION('',(0.,0.374606593415912,0.927183854566787));
#63937=DIRECTION('center_axis',(0.,0.848048096156426,-0.529919264233205));
#63938=DIRECTION('ref_axis',(0.,0.529919264233205,0.848048096156426));
#63939=DIRECTION('',(0.,0.529919264233205,0.848048096156426));
#63940=DIRECTION('',(1.,0.,0.));
#63941=DIRECTION('',(1.,0.,0.));
#63942=DIRECTION('',(1.,0.,0.));
#63943=DIRECTION('',(0.,0.529919264233205,0.848048096156426));
#63944=DIRECTION('center_axis',(0.,0.743144825477394,-0.669130606358858));
#63945=DIRECTION('ref_axis',(0.,0.669130606358858,0.743144825477394));
#63946=DIRECTION('',(0.,0.669130606358858,0.743144825477394));
#63947=DIRECTION('',(1.,0.,0.));
#63948=DIRECTION('',(1.,0.,0.));
#63949=DIRECTION('',(1.,0.,0.));
#63950=DIRECTION('',(0.,0.669130606358858,0.743144825477394));
#63951=DIRECTION('center_axis',(0.,0.615661475325658,-0.788010753606722));
#63952=DIRECTION('ref_axis',(0.,0.788010753606722,0.615661475325658));
#63953=DIRECTION('',(0.,0.788010753606722,0.615661475325658));
#63954=DIRECTION('',(1.,0.,0.));
#63955=DIRECTION('',(1.,0.,0.));
#63956=DIRECTION('',(1.,0.,0.));
#63957=DIRECTION('',(0.,0.788010753606722,0.615661475325658));
#63958=DIRECTION('center_axis',(0.,0.469471562785891,-0.882947592858927));
#63959=DIRECTION('ref_axis',(0.,0.882947592858927,0.469471562785891));
#63960=DIRECTION('',(0.,0.882947592858927,0.469471562785891));
#63961=DIRECTION('',(1.,0.,0.));
#63962=DIRECTION('',(1.,0.,0.));
#63963=DIRECTION('',(1.,0.,0.));
#63964=DIRECTION('',(0.,0.882947592858927,0.469471562785891));
#63965=DIRECTION('center_axis',(0.,0.309016994374948,-0.951056516295154));
#63966=DIRECTION('ref_axis',(0.,0.951056516295154,0.309016994374948));
#63967=DIRECTION('',(0.,0.951056516295154,0.309016994374948));
#63968=DIRECTION('',(1.,0.,0.));
#63969=DIRECTION('',(1.,0.,0.));
#63970=DIRECTION('',(0.,0.951056516295154,0.309016994374948));
#63971=DIRECTION('center_axis',(0.,-0.996194698091746,0.0871557427476582));
#63972=DIRECTION('ref_axis',(0.,-0.0871557427476581,-0.996194698091746));
#63973=DIRECTION('',(0.,-0.0871557427476581,-0.996194698091746));
#63974=DIRECTION('center_axis',(0.,-0.996194698091746,0.0871557427476582));
#63975=DIRECTION('ref_axis',(0.,-0.0871557427476581,-0.996194698091746));
#63976=DIRECTION('',(0.,-0.0871557427476581,-0.996194698091746));
#63977=DIRECTION('center_axis',(1.,0.,0.));
#63978=DIRECTION('ref_axis',(0.,-0.17364817766693,-0.984807753012208));
#63979=DIRECTION('center_axis',(1.,0.,0.));
#63980=DIRECTION('ref_axis',(0.,-0.17364817766693,-0.984807753012208));
#63981=DIRECTION('center_axis',(1.,0.,0.));
#63982=DIRECTION('ref_axis',(0.,1.,0.));
#63983=DIRECTION('center_axis',(1.,0.,0.));
#63984=DIRECTION('ref_axis',(0.,1.,0.));
#63985=DIRECTION('center_axis',(0.,-0.965925826289068,0.258819045102521));
#63986=DIRECTION('ref_axis',(0.,-0.258819045102521,-0.965925826289068));
#63987=DIRECTION('',(0.,-0.258819045102521,-0.965925826289068));
#63988=DIRECTION('center_axis',(0.,-0.965925826289068,0.258819045102521));
#63989=DIRECTION('ref_axis',(0.,-0.258819045102521,-0.965925826289068));
#63990=DIRECTION('',(0.,-0.258819045102521,-0.965925826289068));
#63991=DIRECTION('center_axis',(1.,0.,0.));
#63992=DIRECTION('ref_axis',(0.,-0.342020143325669,-0.939692620785908));
#63993=DIRECTION('center_axis',(1.,0.,0.));
#63994=DIRECTION('ref_axis',(0.,-0.342020143325669,-0.939692620785908));
#63995=DIRECTION('center_axis',(1.,0.,0.));
#63996=DIRECTION('ref_axis',(0.,1.,0.));
#63997=DIRECTION('center_axis',(0.,-0.90630778703665,0.4226182617407));
#63998=DIRECTION('ref_axis',(0.,-0.4226182617407,-0.90630778703665));
#63999=DIRECTION('',(0.,-0.4226182617407,-0.90630778703665));
#64000=DIRECTION('center_axis',(0.,-0.90630778703665,0.4226182617407));
#64001=DIRECTION('ref_axis',(0.,-0.4226182617407,-0.90630778703665));
#64002=DIRECTION('',(0.,-0.4226182617407,-0.90630778703665));
#64003=DIRECTION('center_axis',(1.,0.,0.));
#64004=DIRECTION('ref_axis',(0.,-0.5,-0.866025403784438));
#64005=DIRECTION('center_axis',(1.,0.,0.));
#64006=DIRECTION('ref_axis',(0.,-0.5,-0.866025403784438));
#64007=DIRECTION('center_axis',(1.,0.,0.));
#64008=DIRECTION('ref_axis',(0.,1.,0.));
#64009=DIRECTION('center_axis',(0.,-0.819152044288992,0.573576436351046));
#64010=DIRECTION('ref_axis',(0.,-0.573576436351046,-0.819152044288992));
#64011=DIRECTION('',(0.,-0.573576436351046,-0.819152044288992));
#64012=DIRECTION('center_axis',(0.,-0.819152044288992,0.573576436351046));
#64013=DIRECTION('ref_axis',(0.,-0.573576436351046,-0.819152044288992));
#64014=DIRECTION('',(0.,-0.573576436351046,-0.819152044288992));
#64015=DIRECTION('center_axis',(1.,0.,0.));
#64016=DIRECTION('ref_axis',(0.,-0.64278760968654,-0.766044443118978));
#64017=DIRECTION('center_axis',(1.,0.,0.));
#64018=DIRECTION('ref_axis',(0.,-0.64278760968654,-0.766044443118978));
#64019=DIRECTION('center_axis',(1.,0.,0.));
#64020=DIRECTION('ref_axis',(0.,1.,0.));
#64021=DIRECTION('center_axis',(0.,-0.707106781186547,0.707106781186548));
#64022=DIRECTION('ref_axis',(0.,-0.707106781186548,-0.707106781186547));
#64023=DIRECTION('',(0.,-0.707106781186548,-0.707106781186547));
#64024=DIRECTION('center_axis',(0.,-0.707106781186547,0.707106781186548));
#64025=DIRECTION('ref_axis',(0.,-0.707106781186548,-0.707106781186547));
#64026=DIRECTION('',(0.,-0.707106781186548,-0.707106781186547));
#64027=DIRECTION('center_axis',(1.,0.,0.));
#64028=DIRECTION('ref_axis',(0.,-0.766044443118978,-0.642787609686539));
#64029=DIRECTION('center_axis',(1.,0.,0.));
#64030=DIRECTION('ref_axis',(0.,-0.766044443118978,-0.642787609686539));
#64031=DIRECTION('center_axis',(1.,0.,0.));
#64032=DIRECTION('ref_axis',(0.,1.,0.));
#64033=DIRECTION('center_axis',(0.,-0.573576436351046,0.819152044288992));
#64034=DIRECTION('ref_axis',(0.,-0.819152044288992,-0.573576436351046));
#64035=DIRECTION('',(0.,-0.819152044288992,-0.573576436351046));
#64036=DIRECTION('center_axis',(0.,-0.573576436351046,0.819152044288992));
#64037=DIRECTION('ref_axis',(0.,-0.819152044288992,-0.573576436351046));
#64038=DIRECTION('',(0.,-0.819152044288992,-0.573576436351046));
#64039=DIRECTION('center_axis',(1.,0.,0.));
#64040=DIRECTION('ref_axis',(0.,-0.866025403784439,-0.5));
#64041=DIRECTION('center_axis',(1.,0.,0.));
#64042=DIRECTION('ref_axis',(0.,-0.866025403784439,-0.5));
#64043=DIRECTION('center_axis',(1.,0.,0.));
#64044=DIRECTION('ref_axis',(0.,1.,0.));
#64045=DIRECTION('center_axis',(0.,-0.422618261740699,0.90630778703665));
#64046=DIRECTION('ref_axis',(0.,-0.90630778703665,-0.422618261740699));
#64047=DIRECTION('',(0.,-0.90630778703665,-0.422618261740699));
#64048=DIRECTION('center_axis',(0.,-0.422618261740699,0.90630778703665));
#64049=DIRECTION('ref_axis',(0.,-0.90630778703665,-0.422618261740699));
#64050=DIRECTION('',(0.,-0.90630778703665,-0.422618261740699));
#64051=DIRECTION('center_axis',(1.,0.,0.));
#64052=DIRECTION('ref_axis',(0.,-0.939692620785909,-0.342020143325668));
#64053=DIRECTION('center_axis',(1.,0.,0.));
#64054=DIRECTION('ref_axis',(0.,-0.939692620785909,-0.342020143325668));
#64055=DIRECTION('center_axis',(1.,0.,0.));
#64056=DIRECTION('ref_axis',(0.,1.,0.));
#64057=DIRECTION('center_axis',(0.,-0.25881904510252,0.965925826289068));
#64058=DIRECTION('ref_axis',(0.,-0.965925826289068,-0.25881904510252));
#64059=DIRECTION('',(0.,-0.965925826289068,-0.25881904510252));
#64060=DIRECTION('center_axis',(0.,-0.25881904510252,0.965925826289068));
#64061=DIRECTION('ref_axis',(0.,-0.965925826289068,-0.25881904510252));
#64062=DIRECTION('',(0.,-0.965925826289068,-0.25881904510252));
#64063=DIRECTION('center_axis',(1.,0.,0.));
#64064=DIRECTION('ref_axis',(0.,-0.984807753012208,-0.17364817766693));
#64065=DIRECTION('center_axis',(1.,0.,0.));
#64066=DIRECTION('ref_axis',(0.,-0.984807753012208,-0.17364817766693));
#64067=DIRECTION('center_axis',(1.,0.,0.));
#64068=DIRECTION('ref_axis',(0.,1.,0.));
#64069=DIRECTION('center_axis',(0.,-0.0871557427476581,0.996194698091746));
#64070=DIRECTION('ref_axis',(0.,-0.996194698091746,-0.0871557427476581));
#64071=DIRECTION('',(0.,-0.996194698091746,-0.0871557427476581));
#64072=DIRECTION('center_axis',(0.,-0.0871557427476581,0.996194698091746));
#64073=DIRECTION('ref_axis',(0.,-0.996194698091746,-0.0871557427476581));
#64074=DIRECTION('',(0.,-0.996194698091746,-0.0871557427476581));
#64075=DIRECTION('center_axis',(1.,0.,0.));
#64076=DIRECTION('ref_axis',(0.,-1.,1.83697019872103E-16));
#64077=DIRECTION('center_axis',(1.,0.,0.));
#64078=DIRECTION('ref_axis',(0.,-1.,1.83697019872103E-16));
#64079=DIRECTION('center_axis',(1.,0.,0.));
#64080=DIRECTION('ref_axis',(0.,1.,0.));
#64081=DIRECTION('center_axis',(0.,0.0871557427476581,0.996194698091746));
#64082=DIRECTION('ref_axis',(0.,-0.996194698091746,0.0871557427476581));
#64083=DIRECTION('',(0.,-0.996194698091746,0.0871557427476581));
#64084=DIRECTION('center_axis',(0.,0.0871557427476581,0.996194698091746));
#64085=DIRECTION('ref_axis',(0.,-0.996194698091746,0.0871557427476581));
#64086=DIRECTION('',(0.,-0.996194698091746,0.0871557427476581));
#64087=DIRECTION('center_axis',(1.,0.,0.));
#64088=DIRECTION('ref_axis',(0.,-0.984807753012208,0.17364817766693));
#64089=DIRECTION('center_axis',(1.,0.,0.));
#64090=DIRECTION('ref_axis',(0.,-0.984807753012208,0.17364817766693));
#64091=DIRECTION('center_axis',(1.,0.,0.));
#64092=DIRECTION('ref_axis',(0.,1.,0.));
#64093=DIRECTION('center_axis',(0.,0.258819045102521,0.965925826289068));
#64094=DIRECTION('ref_axis',(0.,-0.965925826289068,0.258819045102521));
#64095=DIRECTION('',(0.,-0.965925826289068,0.258819045102521));
#64096=DIRECTION('center_axis',(0.,0.258819045102521,0.965925826289068));
#64097=DIRECTION('ref_axis',(0.,-0.965925826289068,0.258819045102521));
#64098=DIRECTION('',(0.,-0.965925826289068,0.258819045102521));
#64099=DIRECTION('center_axis',(1.,0.,0.));
#64100=DIRECTION('ref_axis',(0.,-0.939692620785908,0.342020143325669));
#64101=DIRECTION('center_axis',(1.,0.,0.));
#64102=DIRECTION('ref_axis',(0.,-0.939692620785908,0.342020143325669));
#64103=DIRECTION('center_axis',(1.,0.,0.));
#64104=DIRECTION('ref_axis',(0.,1.,0.));
#64105=DIRECTION('center_axis',(0.,0.573576436351046,0.819152044288992));
#64106=DIRECTION('ref_axis',(0.,-0.819152044288992,0.573576436351046));
#64107=DIRECTION('',(0.,-0.819152044288992,0.573576436351046));
#64108=DIRECTION('center_axis',(0.,0.573576436351046,0.819152044288992));
#64109=DIRECTION('ref_axis',(0.,-0.819152044288992,0.573576436351046));
#64110=DIRECTION('',(0.,-0.819152044288992,0.573576436351046));
#64111=DIRECTION('center_axis',(1.,0.,0.));
#64112=DIRECTION('ref_axis',(0.,-0.766044443118978,0.642787609686539));
#64113=DIRECTION('center_axis',(1.,0.,0.));
#64114=DIRECTION('ref_axis',(0.,-0.766044443118978,0.642787609686539));
#64115=DIRECTION('center_axis',(1.,0.,0.));
#64116=DIRECTION('ref_axis',(0.,1.,0.));
#64117=DIRECTION('center_axis',(0.,0.707106781186547,0.707106781186548));
#64118=DIRECTION('ref_axis',(0.,-0.707106781186548,0.707106781186547));
#64119=DIRECTION('',(0.,-0.707106781186548,0.707106781186547));
#64120=DIRECTION('center_axis',(0.,0.707106781186547,0.707106781186548));
#64121=DIRECTION('ref_axis',(0.,-0.707106781186548,0.707106781186547));
#64122=DIRECTION('',(0.,-0.707106781186548,0.707106781186547));
#64123=DIRECTION('center_axis',(1.,0.,0.));
#64124=DIRECTION('ref_axis',(0.,-0.642787609686539,0.766044443118978));
#64125=DIRECTION('center_axis',(1.,0.,0.));
#64126=DIRECTION('ref_axis',(0.,-0.642787609686539,0.766044443118978));
#64127=DIRECTION('center_axis',(1.,0.,0.));
#64128=DIRECTION('ref_axis',(0.,1.,0.));
#64129=DIRECTION('center_axis',(0.,0.819152044288992,0.573576436351046));
#64130=DIRECTION('ref_axis',(0.,-0.573576436351046,0.819152044288992));
#64131=DIRECTION('',(0.,-0.573576436351046,0.819152044288992));
#64132=DIRECTION('center_axis',(0.,0.819152044288992,0.573576436351046));
#64133=DIRECTION('ref_axis',(0.,-0.573576436351046,0.819152044288992));
#64134=DIRECTION('',(0.,-0.573576436351046,0.819152044288992));
#64135=DIRECTION('center_axis',(1.,0.,0.));
#64136=DIRECTION('ref_axis',(0.,-0.5,0.866025403784439));
#64137=DIRECTION('center_axis',(1.,0.,0.));
#64138=DIRECTION('ref_axis',(0.,-0.5,0.866025403784439));
#64139=DIRECTION('center_axis',(1.,0.,0.));
#64140=DIRECTION('ref_axis',(0.,1.,0.));
#64141=DIRECTION('center_axis',(0.,0.90630778703665,0.422618261740699));
#64142=DIRECTION('ref_axis',(0.,-0.422618261740699,0.90630778703665));
#64143=DIRECTION('',(0.,-0.422618261740699,0.90630778703665));
#64144=DIRECTION('center_axis',(0.,0.90630778703665,0.422618261740699));
#64145=DIRECTION('ref_axis',(0.,-0.422618261740699,0.90630778703665));
#64146=DIRECTION('',(0.,-0.422618261740699,0.90630778703665));
#64147=DIRECTION('center_axis',(1.,0.,0.));
#64148=DIRECTION('ref_axis',(0.,-0.342020143325669,0.939692620785909));
#64149=DIRECTION('center_axis',(1.,0.,0.));
#64150=DIRECTION('ref_axis',(0.,-0.342020143325669,0.939692620785909));
#64151=DIRECTION('center_axis',(1.,0.,0.));
#64152=DIRECTION('ref_axis',(0.,1.,0.));
#64153=DIRECTION('center_axis',(0.,0.965925826289068,0.258819045102521));
#64154=DIRECTION('ref_axis',(0.,-0.25881904510252,0.965925826289068));
#64155=DIRECTION('',(0.,-0.25881904510252,0.965925826289068));
#64156=DIRECTION('center_axis',(0.,0.965925826289068,0.258819045102521));
#64157=DIRECTION('ref_axis',(0.,-0.25881904510252,0.965925826289068));
#64158=DIRECTION('',(0.,-0.25881904510252,0.965925826289068));
#64159=DIRECTION('center_axis',(1.,0.,0.));
#64160=DIRECTION('ref_axis',(0.,-0.17364817766693,0.984807753012208));
#64161=DIRECTION('center_axis',(1.,0.,0.));
#64162=DIRECTION('ref_axis',(0.,-0.17364817766693,0.984807753012208));
#64163=DIRECTION('center_axis',(1.,0.,0.));
#64164=DIRECTION('ref_axis',(0.,1.,0.));
#64165=DIRECTION('center_axis',(0.,0.996194698091746,0.0871557427476581));
#64166=DIRECTION('ref_axis',(0.,-0.0871557427476581,0.996194698091746));
#64167=DIRECTION('',(0.,-0.0871557427476581,0.996194698091746));
#64168=DIRECTION('center_axis',(0.,0.996194698091746,0.0871557427476581));
#64169=DIRECTION('ref_axis',(0.,-0.0871557427476581,0.996194698091746));
#64170=DIRECTION('',(0.,-0.0871557427476581,0.996194698091746));
#64171=DIRECTION('center_axis',(1.,0.,0.));
#64172=DIRECTION('ref_axis',(0.,1.22464679914735E-16,1.));
#64173=DIRECTION('center_axis',(1.,0.,0.));
#64174=DIRECTION('ref_axis',(0.,1.22464679914735E-16,1.));
#64175=DIRECTION('center_axis',(1.,0.,0.));
#64176=DIRECTION('ref_axis',(0.,-1.,-1.22464679914735E-16));
#64177=DIRECTION('center_axis',(0.,0.996194698091746,-0.0871557427476584));
#64178=DIRECTION('ref_axis',(0.,0.0871557427476584,0.996194698091746));
#64179=DIRECTION('',(0.,0.0871557427476584,0.996194698091746));
#64180=DIRECTION('center_axis',(0.,0.996194698091746,-0.0871557427476584));
#64181=DIRECTION('ref_axis',(0.,0.0871557427476584,0.996194698091746));
#64182=DIRECTION('',(0.,0.0871557427476584,0.996194698091746));
#64183=DIRECTION('center_axis',(1.,0.,0.));
#64184=DIRECTION('ref_axis',(0.,0.173648177666931,0.984807753012208));
#64185=DIRECTION('center_axis',(1.,0.,0.));
#64186=DIRECTION('ref_axis',(0.,0.173648177666931,0.984807753012208));
#64187=DIRECTION('center_axis',(1.,0.,0.));
#64188=DIRECTION('ref_axis',(0.,1.,0.));
#64189=DIRECTION('center_axis',(0.,0.965925826289068,-0.258819045102521));
#64190=DIRECTION('ref_axis',(0.,0.258819045102521,0.965925826289068));
#64191=DIRECTION('',(0.,0.258819045102521,0.965925826289068));
#64192=DIRECTION('center_axis',(0.,0.965925826289068,-0.258819045102521));
#64193=DIRECTION('ref_axis',(0.,0.258819045102521,0.965925826289068));
#64194=DIRECTION('',(0.,0.258819045102521,0.965925826289068));
#64195=DIRECTION('center_axis',(1.,0.,0.));
#64196=DIRECTION('ref_axis',(0.,0.342020143325669,0.939692620785908));
#64197=DIRECTION('center_axis',(1.,0.,0.));
#64198=DIRECTION('ref_axis',(0.,0.342020143325669,0.939692620785908));
#64199=DIRECTION('center_axis',(1.,0.,0.));
#64200=DIRECTION('ref_axis',(0.,1.,0.));
#64201=DIRECTION('center_axis',(0.,0.90630778703665,-0.422618261740699));
#64202=DIRECTION('ref_axis',(0.,0.422618261740699,0.90630778703665));
#64203=DIRECTION('',(0.,0.422618261740699,0.90630778703665));
#64204=DIRECTION('center_axis',(0.,0.90630778703665,-0.422618261740699));
#64205=DIRECTION('ref_axis',(0.,0.422618261740699,0.90630778703665));
#64206=DIRECTION('',(0.,0.422618261740699,0.90630778703665));
#64207=DIRECTION('center_axis',(1.,0.,0.));
#64208=DIRECTION('ref_axis',(0.,0.5,0.866025403784439));
#64209=DIRECTION('center_axis',(1.,0.,0.));
#64210=DIRECTION('ref_axis',(0.,0.5,0.866025403784439));
#64211=DIRECTION('center_axis',(1.,0.,0.));
#64212=DIRECTION('ref_axis',(0.,1.,0.));
#64213=DIRECTION('center_axis',(0.,0.819152044288992,-0.573576436351046));
#64214=DIRECTION('ref_axis',(0.,0.573576436351046,0.819152044288992));
#64215=DIRECTION('',(0.,0.573576436351046,0.819152044288992));
#64216=DIRECTION('center_axis',(0.,0.819152044288992,-0.573576436351046));
#64217=DIRECTION('ref_axis',(0.,0.573576436351046,0.819152044288992));
#64218=DIRECTION('',(0.,0.573576436351046,0.819152044288992));
#64219=DIRECTION('center_axis',(1.,0.,0.));
#64220=DIRECTION('ref_axis',(0.,0.642787609686539,0.766044443118978));
#64221=DIRECTION('center_axis',(1.,0.,0.));
#64222=DIRECTION('ref_axis',(0.,0.642787609686539,0.766044443118978));
#64223=DIRECTION('center_axis',(1.,0.,0.));
#64224=DIRECTION('ref_axis',(0.,1.,0.));
#64225=DIRECTION('center_axis',(0.,0.707106781186548,-0.707106781186547));
#64226=DIRECTION('ref_axis',(0.,0.707106781186547,0.707106781186548));
#64227=DIRECTION('',(0.,0.707106781186547,0.707106781186548));
#64228=DIRECTION('center_axis',(0.,0.707106781186548,-0.707106781186547));
#64229=DIRECTION('ref_axis',(0.,0.707106781186547,0.707106781186548));
#64230=DIRECTION('',(0.,0.707106781186547,0.707106781186548));
#64231=DIRECTION('center_axis',(1.,0.,0.));
#64232=DIRECTION('ref_axis',(0.,0.766044443118978,0.642787609686539));
#64233=DIRECTION('center_axis',(1.,0.,0.));
#64234=DIRECTION('ref_axis',(0.,0.766044443118978,0.642787609686539));
#64235=DIRECTION('center_axis',(1.,0.,0.));
#64236=DIRECTION('ref_axis',(0.,1.,0.));
#64237=DIRECTION('center_axis',(0.,0.422618261740699,-0.90630778703665));
#64238=DIRECTION('ref_axis',(0.,0.90630778703665,0.422618261740699));
#64239=DIRECTION('',(0.,0.90630778703665,0.422618261740699));
#64240=DIRECTION('center_axis',(0.,0.422618261740699,-0.90630778703665));
#64241=DIRECTION('ref_axis',(0.,0.90630778703665,0.422618261740699));
#64242=DIRECTION('',(0.,0.90630778703665,0.422618261740699));
#64243=DIRECTION('center_axis',(1.,0.,0.));
#64244=DIRECTION('ref_axis',(0.,0.939692620785908,0.342020143325669));
#64245=DIRECTION('center_axis',(1.,0.,0.));
#64246=DIRECTION('ref_axis',(0.,0.939692620785908,0.342020143325669));
#64247=DIRECTION('center_axis',(1.,0.,0.));
#64248=DIRECTION('ref_axis',(0.,1.,0.));
#64249=DIRECTION('center_axis',(0.,0.258819045102521,-0.965925826289068));
#64250=DIRECTION('ref_axis',(0.,0.965925826289068,0.258819045102521));
#64251=DIRECTION('',(0.,0.965925826289068,0.258819045102521));
#64252=DIRECTION('center_axis',(0.,0.258819045102521,-0.965925826289068));
#64253=DIRECTION('ref_axis',(0.,0.965925826289068,0.258819045102521));
#64254=DIRECTION('',(0.,0.965925826289068,0.258819045102521));
#64255=DIRECTION('center_axis',(1.,0.,0.));
#64256=DIRECTION('ref_axis',(0.,0.984807753012208,0.17364817766693));
#64257=DIRECTION('center_axis',(1.,0.,0.));
#64258=DIRECTION('ref_axis',(0.,0.984807753012208,0.17364817766693));
#64259=DIRECTION('center_axis',(1.,0.,0.));
#64260=DIRECTION('ref_axis',(0.,1.,0.));
#64261=DIRECTION('center_axis',(0.,0.0871557427476582,-0.996194698091746));
#64262=DIRECTION('ref_axis',(0.,0.996194698091746,0.0871557427476582));
#64263=DIRECTION('',(0.,0.996194698091746,0.0871557427476582));
#64264=DIRECTION('center_axis',(0.,0.0871557427476582,-0.996194698091746));
#64265=DIRECTION('ref_axis',(0.,0.996194698091746,0.0871557427476582));
#64266=DIRECTION('',(0.,0.996194698091746,0.0871557427476582));
#64267=DIRECTION('center_axis',(1.,0.,0.));
#64268=DIRECTION('ref_axis',(0.,1.,-6.12323399573677E-17));
#64269=DIRECTION('center_axis',(1.,0.,0.));
#64270=DIRECTION('ref_axis',(0.,1.,-6.12323399573677E-17));
#64271=DIRECTION('center_axis',(1.,0.,0.));
#64272=DIRECTION('ref_axis',(0.,1.,0.));
#64273=DIRECTION('center_axis',(0.,-0.0871557427476582,-0.996194698091746));
#64274=DIRECTION('ref_axis',(0.,0.996194698091746,-0.0871557427476582));
#64275=DIRECTION('',(0.,0.996194698091746,-0.0871557427476582));
#64276=DIRECTION('center_axis',(0.,-0.0871557427476582,-0.996194698091746));
#64277=DIRECTION('ref_axis',(0.,0.996194698091746,-0.0871557427476582));
#64278=DIRECTION('',(0.,0.996194698091746,-0.0871557427476582));
#64279=DIRECTION('center_axis',(1.,0.,0.));
#64280=DIRECTION('ref_axis',(0.,0.984807753012208,-0.17364817766693));
#64281=DIRECTION('center_axis',(1.,0.,0.));
#64282=DIRECTION('ref_axis',(0.,0.984807753012208,-0.17364817766693));
#64283=DIRECTION('center_axis',(1.,0.,0.));
#64284=DIRECTION('ref_axis',(0.,1.,0.));
#64285=DIRECTION('center_axis',(0.,-0.258819045102521,-0.965925826289068));
#64286=DIRECTION('ref_axis',(0.,0.965925826289068,-0.258819045102521));
#64287=DIRECTION('',(0.,0.965925826289068,-0.258819045102521));
#64288=DIRECTION('center_axis',(0.,-0.258819045102521,-0.965925826289068));
#64289=DIRECTION('ref_axis',(0.,0.965925826289068,-0.258819045102521));
#64290=DIRECTION('',(0.,0.965925826289068,-0.258819045102521));
#64291=DIRECTION('center_axis',(1.,0.,0.));
#64292=DIRECTION('ref_axis',(0.,0.939692620785908,-0.342020143325669));
#64293=DIRECTION('center_axis',(1.,0.,0.));
#64294=DIRECTION('ref_axis',(0.,0.939692620785908,-0.342020143325669));
#64295=DIRECTION('center_axis',(1.,0.,0.));
#64296=DIRECTION('ref_axis',(0.,1.,0.));
#64297=DIRECTION('center_axis',(0.,-0.422618261740699,-0.90630778703665));
#64298=DIRECTION('ref_axis',(0.,0.90630778703665,-0.422618261740699));
#64299=DIRECTION('',(0.,0.90630778703665,-0.422618261740699));
#64300=DIRECTION('center_axis',(0.,-0.422618261740699,-0.90630778703665));
#64301=DIRECTION('ref_axis',(0.,0.90630778703665,-0.422618261740699));
#64302=DIRECTION('',(0.,0.90630778703665,-0.422618261740699));
#64303=DIRECTION('center_axis',(1.,0.,0.));
#64304=DIRECTION('ref_axis',(0.,0.866025403784439,-0.5));
#64305=DIRECTION('center_axis',(1.,0.,0.));
#64306=DIRECTION('ref_axis',(0.,0.866025403784439,-0.5));
#64307=DIRECTION('center_axis',(1.,0.,0.));
#64308=DIRECTION('ref_axis',(0.,1.,0.));
#64309=DIRECTION('center_axis',(0.,-0.573576436351046,-0.819152044288992));
#64310=DIRECTION('ref_axis',(0.,0.819152044288992,-0.573576436351046));
#64311=DIRECTION('',(0.,0.819152044288992,-0.573576436351046));
#64312=DIRECTION('center_axis',(0.,-0.573576436351046,-0.819152044288992));
#64313=DIRECTION('ref_axis',(0.,0.819152044288992,-0.573576436351046));
#64314=DIRECTION('',(0.,0.819152044288992,-0.573576436351046));
#64315=DIRECTION('center_axis',(1.,0.,0.));
#64316=DIRECTION('ref_axis',(0.,0.766044443118978,-0.642787609686539));
#64317=DIRECTION('center_axis',(1.,0.,0.));
#64318=DIRECTION('ref_axis',(0.,0.766044443118978,-0.642787609686539));
#64319=DIRECTION('center_axis',(1.,0.,0.));
#64320=DIRECTION('ref_axis',(0.,1.,0.));
#64321=DIRECTION('center_axis',(0.,-0.707106781186547,-0.707106781186548));
#64322=DIRECTION('ref_axis',(0.,0.707106781186548,-0.707106781186547));
#64323=DIRECTION('',(0.,0.707106781186548,-0.707106781186547));
#64324=DIRECTION('center_axis',(0.,-0.707106781186547,-0.707106781186548));
#64325=DIRECTION('ref_axis',(0.,0.707106781186548,-0.707106781186547));
#64326=DIRECTION('',(0.,0.707106781186548,-0.707106781186547));
#64327=DIRECTION('center_axis',(1.,0.,0.));
#64328=DIRECTION('ref_axis',(0.,0.642787609686539,-0.766044443118978));
#64329=DIRECTION('center_axis',(1.,0.,0.));
#64330=DIRECTION('ref_axis',(0.,0.642787609686539,-0.766044443118978));
#64331=DIRECTION('center_axis',(1.,0.,0.));
#64332=DIRECTION('ref_axis',(0.,1.,0.));
#64333=DIRECTION('center_axis',(0.,-0.819152044288992,-0.573576436351046));
#64334=DIRECTION('ref_axis',(0.,0.573576436351046,-0.819152044288992));
#64335=DIRECTION('',(0.,0.573576436351046,-0.819152044288992));
#64336=DIRECTION('center_axis',(0.,-0.819152044288992,-0.573576436351046));
#64337=DIRECTION('ref_axis',(0.,0.573576436351046,-0.819152044288992));
#64338=DIRECTION('',(0.,0.573576436351046,-0.819152044288992));
#64339=DIRECTION('center_axis',(1.,0.,0.));
#64340=DIRECTION('ref_axis',(0.,0.5,-0.866025403784439));
#64341=DIRECTION('center_axis',(1.,0.,0.));
#64342=DIRECTION('ref_axis',(0.,0.5,-0.866025403784439));
#64343=DIRECTION('center_axis',(1.,0.,0.));
#64344=DIRECTION('ref_axis',(0.,1.,0.));
#64345=DIRECTION('center_axis',(0.,-0.90630778703665,-0.422618261740699));
#64346=DIRECTION('ref_axis',(0.,0.422618261740699,-0.90630778703665));
#64347=DIRECTION('',(0.,0.422618261740699,-0.90630778703665));
#64348=DIRECTION('center_axis',(0.,-0.90630778703665,-0.422618261740699));
#64349=DIRECTION('ref_axis',(0.,0.422618261740699,-0.90630778703665));
#64350=DIRECTION('',(0.,0.422618261740699,-0.90630778703665));
#64351=DIRECTION('center_axis',(1.,0.,0.));
#64352=DIRECTION('ref_axis',(0.,0.342020143325669,-0.939692620785908));
#64353=DIRECTION('center_axis',(1.,0.,0.));
#64354=DIRECTION('ref_axis',(0.,0.342020143325669,-0.939692620785908));
#64355=DIRECTION('center_axis',(1.,0.,0.));
#64356=DIRECTION('ref_axis',(0.,1.,0.));
#64357=DIRECTION('center_axis',(0.,-0.965925826289068,-0.258819045102521));
#64358=DIRECTION('ref_axis',(0.,0.258819045102521,-0.965925826289068));
#64359=DIRECTION('',(0.,0.258819045102521,-0.965925826289068));
#64360=DIRECTION('center_axis',(0.,-0.965925826289068,-0.258819045102521));
#64361=DIRECTION('ref_axis',(0.,0.258819045102521,-0.965925826289068));
#64362=DIRECTION('',(0.,0.258819045102521,-0.965925826289068));
#64363=DIRECTION('center_axis',(1.,0.,0.));
#64364=DIRECTION('ref_axis',(0.,0.17364817766693,-0.984807753012208));
#64365=DIRECTION('center_axis',(1.,0.,0.));
#64366=DIRECTION('ref_axis',(0.,0.17364817766693,-0.984807753012208));
#64367=DIRECTION('center_axis',(1.,0.,0.));
#64368=DIRECTION('ref_axis',(0.,0.,-1.));
#64369=DIRECTION('center_axis',(1.,0.,0.));
#64370=DIRECTION('ref_axis',(0.,-1.,1.83697019872103E-16));
#64371=DIRECTION('center_axis',(0.,-1.,-1.22464679914735E-16));
#64372=DIRECTION('ref_axis',(0.,-1.22464679914735E-16,1.));
#64373=DIRECTION('center_axis',(-1.,0.,0.));
#64374=DIRECTION('ref_axis',(0.,-1.,1.83697019872103E-16));
#64375=DIRECTION('center_axis',(1.,0.,0.));
#64376=DIRECTION('ref_axis',(0.,-1.,1.83697019872103E-16));
#64377=DIRECTION('center_axis',(1.,0.,0.));
#64378=DIRECTION('ref_axis',(0.,0.,-1.));
#64379=DIRECTION('center_axis',(1.,0.,0.));
#64380=DIRECTION('ref_axis',(0.,-1.,1.83697019872103E-16));
#64381=DIRECTION('center_axis',(1.,0.,0.));
#64382=DIRECTION('ref_axis',(0.,1.,0.));
#64383=DIRECTION('center_axis',(1.,0.,0.));
#64384=DIRECTION('ref_axis',(0.,0.,-1.));
#64385=DIRECTION('',(-1.,0.,0.));
#64386=DIRECTION('center_axis',(1.,0.,0.));
#64387=DIRECTION('ref_axis',(0.,0.,-1.));
#64388=DIRECTION('center_axis',(1.,0.,0.));
#64389=DIRECTION('ref_axis',(0.,-1.,1.83697019872103E-16));
#64390=DIRECTION('center_axis',(0.,-1.,-1.22464679914735E-16));
#64391=DIRECTION('ref_axis',(0.,-1.22464679914735E-16,1.));
#64392=DIRECTION('center_axis',(-1.,0.,0.));
#64393=DIRECTION('ref_axis',(0.,-1.,1.83697019872103E-16));
#64394=DIRECTION('center_axis',(-1.,0.,0.));
#64395=DIRECTION('ref_axis',(0.,-1.,1.83697019872103E-16));
#64396=DIRECTION('center_axis',(-1.,0.,0.));
#64397=DIRECTION('ref_axis',(0.,0.,1.));
#64398=DIRECTION('center_axis',(-1.,0.,0.));
#64399=DIRECTION('ref_axis',(0.,-1.,1.83697019872103E-16));
#64400=DIRECTION('center_axis',(1.,0.,0.));
#64401=DIRECTION('ref_axis',(0.,1.,0.));
#64402=DIRECTION('',(-1.,0.,0.));
#64403=DIRECTION('center_axis',(1.,0.,0.));
#64404=DIRECTION('ref_axis',(0.,0.,-1.));
#64405=DIRECTION('center_axis',(0.,-1.,-1.22464679914735E-16));
#64406=DIRECTION('ref_axis',(0.,-1.22464679914735E-16,1.));
#64407=DIRECTION('center_axis',(-1.,0.,0.));
#64408=DIRECTION('ref_axis',(0.,-1.,1.83697019872103E-16));
#64409=DIRECTION('center_axis',(-1.,0.,0.));
#64410=DIRECTION('ref_axis',(0.,-1.,1.83697019872103E-16));
#64411=DIRECTION('center_axis',(1.,0.,0.));
#64412=DIRECTION('ref_axis',(0.,1.,0.));
#64413=DIRECTION('center_axis',(1.,0.,0.));
#64414=DIRECTION('ref_axis',(0.,0.,-1.));
#64415=DIRECTION('',(-1.,0.,0.));
#64416=DIRECTION('center_axis',(1.,0.,0.));
#64417=DIRECTION('ref_axis',(0.,0.,-1.));
#64418=DIRECTION('center_axis',(1.,0.,0.));
#64419=DIRECTION('ref_axis',(0.,-1.,1.83697019872103E-16));
#64420=DIRECTION('center_axis',(0.,-1.,-1.22464679914735E-16));
#64421=DIRECTION('ref_axis',(0.,-1.22464679914735E-16,1.));
#64422=DIRECTION('center_axis',(1.,0.,0.));
#64423=DIRECTION('ref_axis',(0.,-1.,1.83697019872103E-16));
#64424=DIRECTION('center_axis',(1.,0.,0.));
#64425=DIRECTION('ref_axis',(0.,1.,0.));
#64426=DIRECTION('',(-1.,0.,0.));
#64427=DIRECTION('center_axis',(1.,0.,0.));
#64428=DIRECTION('ref_axis',(0.,0.,-1.));
#64429=DIRECTION('center_axis',(1.,0.,0.));
#64430=DIRECTION('ref_axis',(0.,1.,0.));
#64431=DIRECTION('center_axis',(1.,0.,0.));
#64432=DIRECTION('ref_axis',(0.,0.,-1.));
#64433=DIRECTION('',(-1.,0.,0.));
#64434=DIRECTION('center_axis',(1.,0.,0.));
#64435=DIRECTION('ref_axis',(0.,0.,-1.));
#64436=DIRECTION('center_axis',(-1.,0.,0.));
#64437=DIRECTION('ref_axis',(0.,1.,0.));
#64438=DIRECTION('',(-0.707106781186547,-0.707106781186548,-8.65956056235494E-17));
#64439=DIRECTION('center_axis',(1.,0.,0.));
#64440=DIRECTION('ref_axis',(0.,0.,-1.));
#64441=DIRECTION('center_axis',(-1.,0.,0.));
#64442=DIRECTION('ref_axis',(0.,0.,1.));
#64443=DIRECTION('center_axis',(1.,0.,0.));
#64444=DIRECTION('ref_axis',(0.,0.,-1.));
#64445=DIRECTION('center_axis',(1.,0.,0.));
#64446=DIRECTION('ref_axis',(0.,0.,-1.));
#64447=DIRECTION('center_axis',(1.,0.,0.));
#64448=DIRECTION('ref_axis',(0.,0.,-1.));
#64449=DIRECTION('center_axis',(1.,0.,0.));
#64450=DIRECTION('ref_axis',(0.,1.,0.));
#64451=DIRECTION('',(-0.707106781186548,0.707106781186548,8.65956056235493E-17));
#77416=CARTESIAN_POINT('',(0.,0.,0.));
#77417=CARTESIAN_POINT('Origin',(0.,-14.743395421685,-41.6736702420106));
#77418=CARTESIAN_POINT('',(22.,-11.8091924752874,-35.3812517172812));
#77419=CARTESIAN_POINT('',(21.5,-12.0218682747234,-35.8373364409968));
#77420=CARTESIAN_POINT('Ctrl Pts',(22.,-11.8091924752874,-35.3812517172812));
#77421=CARTESIAN_POINT('Ctrl Pts',(21.7516860396895,-11.9148224027831,-35.6077758278089));
#77422=CARTESIAN_POINT('Ctrl Pts',(21.5,-12.0218682747234,-35.8373364409968));
#77423=CARTESIAN_POINT('',(22.,-10.7707837613225,-33.154377043866));
#77424=CARTESIAN_POINT('',(22.,-2.40948834572521,-15.223521160693));
#77425=CARTESIAN_POINT('',(0.,-10.7707837613225,-33.154377043866));
#77426=CARTESIAN_POINT('',(0.,-10.7707837613225,-33.154377043866));
#77427=CARTESIAN_POINT('',(3.46944695195361E-17,-11.8091924752874,-35.3812517172812));
#77428=CARTESIAN_POINT('',(0.,-2.11478812371661,-14.5915344951198));
#77429=CARTESIAN_POINT('',(0.499999999999998,-12.0218682747234,-35.8373364409968));
#77430=CARTESIAN_POINT('Ctrl Pts',(0.500000000000005,-12.0218682747234,
-35.8373364409968));
#77431=CARTESIAN_POINT('Ctrl Pts',(0.248313955079475,-11.9148224005581,
-35.6077758230372));
#77432=CARTESIAN_POINT('Ctrl Pts',(2.08166817117217E-16,-11.8091924752874,
-35.3812517172812));
#77433=CARTESIAN_POINT('',(11.,-12.0218682747234,-35.8373364409968));
#77434=CARTESIAN_POINT('Origin',(0.,-18.474399951134,-29.5621218190701));
#77435=CARTESIAN_POINT('',(21.5,-19.725484464535,-32.2450812162009));
#77436=CARTESIAN_POINT('',(22.,-19.5128086650989,-31.7889964924853));
#77437=CARTESIAN_POINT('Ctrl Pts',(21.5,-19.725484464535,-32.2450812162009));
#77438=CARTESIAN_POINT('Ctrl Pts',(21.7516860442549,-19.6184385906528,-32.0155205988484));
#77439=CARTESIAN_POINT('Ctrl Pts',(22.,-19.5128086650989,-31.7889964924853));
#77440=CARTESIAN_POINT('',(0.499999999999998,-19.725484464535,-32.2450812162009));
#77441=CARTESIAN_POINT('',(11.,-19.725484464535,-32.2450812162009));
#77442=CARTESIAN_POINT('',(6.93889390390723E-17,-19.5128086650989,-31.7889964924853));
#77443=CARTESIAN_POINT('Ctrl Pts',(-2.08166817117217E-16,-19.5128086650989,
-31.7889964924853));
#77444=CARTESIAN_POINT('Ctrl Pts',(0.248313955054683,-19.6184385903591,
-32.0155205982187));
#77445=CARTESIAN_POINT('Ctrl Pts',(0.500000000000004,-19.725484464535,-32.2450812162009));
#77446=CARTESIAN_POINT('',(0.,-18.474399951134,-29.5621218190701));
#77447=CARTESIAN_POINT('',(0.,-7.83209848334684,-6.73963267125159));
#77448=CARTESIAN_POINT('',(22.,-18.474399951134,-29.5621218190701));
#77449=CARTESIAN_POINT('',(0.,-18.474399951134,-29.5621218190701));
#77450=CARTESIAN_POINT('',(22.,-8.12679870535545,-7.37161933682474));
#77451=CARTESIAN_POINT('Origin',(0.,-10.7707837613225,-33.154377043866));
#77452=CARTESIAN_POINT('',(0.,2.62230665155162,-39.3996776697515));
#77453=CARTESIAN_POINT('',(22.,1.26700687356023,-38.7676910041784));
#77454=CARTESIAN_POINT('Origin',(11.,0.,0.));
#77455=CARTESIAN_POINT('',(0.499999999999998,-11.3395294590896,-36.0590497884572));
#77456=CARTESIAN_POINT('Origin',(0.499999999999998,0.,0.));
#77457=CARTESIAN_POINT('',(21.5,-11.3395294590896,-36.0590497884572));
#77458=CARTESIAN_POINT('',(11.,-11.3395294590896,-36.0590497884572));
#77459=CARTESIAN_POINT('Origin',(21.5,0.,0.));
#77460=CARTESIAN_POINT('Origin',(21.75,0.,0.));
#77461=CARTESIAN_POINT('',(22.,-24.7364665672137,27.9176865404195));
#77462=CARTESIAN_POINT('Origin',(22.,0.,0.));
#77463=CARTESIAN_POINT('',(21.5,-25.0251096245113,28.3299115473591));
#77464=CARTESIAN_POINT('Ctrl Pts',(22.,-24.7364665672137,27.9176865404195));
#77465=CARTESIAN_POINT('Ctrl Pts',(21.7516860460885,-24.8798272340583,28.1224267910188));
#77466=CARTESIAN_POINT('Ctrl Pts',(21.5,-25.0251096245113,28.3299115473591));
#77467=CARTESIAN_POINT('',(21.5,-25.5582884235871,27.8498454727622));
#77468=CARTESIAN_POINT('Origin',(21.5,0.,0.));
#77469=CARTESIAN_POINT('',(21.8,-25.3343218406523,27.6481850557002));
#77470=CARTESIAN_POINT('Ctrl Pts',(21.5,-25.5582884235871,27.8498454727622));
#77471=CARTESIAN_POINT('Ctrl Pts',(21.650603110123,-25.4458589814141,27.7486135483316));
#77472=CARTESIAN_POINT('Ctrl Pts',(21.8,-25.3343218406523,27.6481850557002));
#77473=CARTESIAN_POINT('',(21.8,-27.6481850557002,25.3343218406523));
#77474=CARTESIAN_POINT('Ctrl Pts',(21.8,-25.3343218406523,27.6481850557002));
#77475=CARTESIAN_POINT('Ctrl Pts',(21.8713861730393,-26.4912534481763,26.4912534481763));
#77476=CARTESIAN_POINT('Ctrl Pts',(21.8,-27.6481850557002,25.3343218406523));
#77477=CARTESIAN_POINT('',(21.5,-27.8498454727622,25.5582884235871));
#77478=CARTESIAN_POINT('Ctrl Pts',(21.8,-27.6481850557002,25.3343218406523));
#77479=CARTESIAN_POINT('Ctrl Pts',(21.6506031060906,-27.7486135510424,25.4458589844248));
#77480=CARTESIAN_POINT('Ctrl Pts',(21.5,-27.8498454727622,25.5582884235871));
#77481=CARTESIAN_POINT('',(21.5,-30.0060755079215,22.9885935327265));
#77482=CARTESIAN_POINT('Origin',(21.5,0.,0.));
#77483=CARTESIAN_POINT('',(21.8,-29.7504935167013,22.8288881795131));
#77484=CARTESIAN_POINT('Ctrl Pts',(21.5,-30.0060755079215,22.9885935327265));
#77485=CARTESIAN_POINT('Ctrl Pts',(21.6506031103503,-29.87777538221,22.9084227163233));
#77486=CARTESIAN_POINT('Ctrl Pts',(21.8,-29.7504935167013,22.8288881795131));
#77487=CARTESIAN_POINT('',(21.8,-31.6274058196267,20.1483796152605));
#77488=CARTESIAN_POINT('Ctrl Pts',(21.8,-29.7504935167013,22.8288881795131));
#77489=CARTESIAN_POINT('Ctrl Pts',(21.8713861730394,-30.688949668164,21.4886338973868));
#77490=CARTESIAN_POINT('Ctrl Pts',(21.8,-31.6274058196267,20.1483796152605));
#77491=CARTESIAN_POINT('',(21.5,-31.8648939508099,20.3339256786199));
#77492=CARTESIAN_POINT('Ctrl Pts',(21.8,-31.6274058196267,20.1483796152605));
#77493=CARTESIAN_POINT('Ctrl Pts',(21.6506031078004,-31.7456768008676,20.2407830329369));
#77494=CARTESIAN_POINT('Ctrl Pts',(21.5,-31.8648939508099,20.3339256786199));
#77495=CARTESIAN_POINT('',(21.5,-33.5421431717545,17.4288448109885));
#77496=CARTESIAN_POINT('Origin',(21.5,0.,0.));
#77497=CARTESIAN_POINT('',(21.8,-33.2627115017215,17.3159470879662));
#77498=CARTESIAN_POINT('Ctrl Pts',(21.5,-33.5421431717545,17.4288448109885));
#77499=CARTESIAN_POINT('Ctrl Pts',(21.6506031076066,-33.4018706996267,17.3721710534861));
#77500=CARTESIAN_POINT('Ctrl Pts',(21.8,-33.2627115017215,17.3159470879662));
#77501=CARTESIAN_POINT('',(21.8,-34.6456438619633,14.3502390708311));
#77502=CARTESIAN_POINT('Ctrl Pts',(21.8,-33.2627115017215,17.3159470879662));
#77503=CARTESIAN_POINT('Ctrl Pts',(21.8713861730393,-33.9541776818424,15.8330930793986));
#77504=CARTESIAN_POINT('Ctrl Pts',(21.8,-34.6456438619633,14.3502390708311));
#77505=CARTESIAN_POINT('',(21.5,-34.9117437505765,14.4917268913708));
#77506=CARTESIAN_POINT('Ctrl Pts',(21.8,-34.6456438619633,14.3502390708311));
#77507=CARTESIAN_POINT('Ctrl Pts',(21.6506031051379,-34.7781637286973,14.420701133856));
#77508=CARTESIAN_POINT('Ctrl Pts',(21.5,-34.9117437505765,14.4917268913708));
#77509=CARTESIAN_POINT('',(21.5,-36.0590497884572,11.3395294590896));
#77510=CARTESIAN_POINT('Origin',(21.5,0.,0.));
#77511=CARTESIAN_POINT('',(21.8,-35.764258829506,11.2768697064435));
#77512=CARTESIAN_POINT('Ctrl Pts',(21.5,-36.0590497884572,11.3395294590896));
#77513=CARTESIAN_POINT('Ctrl Pts',(21.6506031114238,-35.9110670719085,11.3080747616734));
#77514=CARTESIAN_POINT('Ctrl Pts',(21.8,-35.764258829506,11.2768697064435));
#77515=CARTESIAN_POINT('',(21.8,-36.6111915470959,8.11607377380575));
#77516=CARTESIAN_POINT('Ctrl Pts',(21.8,-35.764258829506,11.2768697064435));
#77517=CARTESIAN_POINT('Ctrl Pts',(21.8713861730393,-36.1877251883009,9.69647174012463));
#77518=CARTESIAN_POINT('Ctrl Pts',(21.8,-36.6111915470959,8.11607377380575));
#77519=CARTESIAN_POINT('',(21.5,-36.8978178826767,8.20920431569502));
#77520=CARTESIAN_POINT('Ctrl Pts',(21.8,-36.6111915470959,8.11607377380575));
#77521=CARTESIAN_POINT('Ctrl Pts',(21.6506031086383,-36.7539337447779,8.16245352531621));
#77522=CARTESIAN_POINT('Ctrl Pts',(21.5,-36.8978178826767,8.20920431569502));
#77523=CARTESIAN_POINT('',(21.5,-37.4803204240973,4.90566824265508));
#77524=CARTESIAN_POINT('Origin',(21.5,0.,0.));
#77525=CARTESIAN_POINT('',(21.8,-37.1791272503441,4.89515034526196));
#77526=CARTESIAN_POINT('Ctrl Pts',(21.5,-37.4803204240973,4.90566824265508));
#77527=CARTESIAN_POINT('Ctrl Pts',(21.6506031095962,-37.3291238484779,4.90038834188993));
#77528=CARTESIAN_POINT('Ctrl Pts',(21.8,-37.1791272503441,4.89515034526196));
#77529=CARTESIAN_POINT('',(21.8,-37.4643267032267,1.63530568209484));
#77530=CARTESIAN_POINT('Ctrl Pts',(21.8,-37.1791272503441,4.89515034526196));
#77531=CARTESIAN_POINT('Ctrl Pts',(21.8713861730394,-37.3217269767854,3.26522801367839));
#77532=CARTESIAN_POINT('Ctrl Pts',(21.8,-37.4643267032267,1.63530568209484));
#77533=CARTESIAN_POINT('',(21.5,-37.7627704896084,1.67724922094466));
#77534=CARTESIAN_POINT('Ctrl Pts',(21.8,-37.4643267032268,1.63530568209484));
#77535=CARTESIAN_POINT('Ctrl Pts',(21.6506031090722,-37.6129540850848,1.65619389840079));
#77536=CARTESIAN_POINT('Ctrl Pts',(21.5,-37.7627704896084,1.67724922094466));
#77537=CARTESIAN_POINT('',(21.5,-37.7627704896084,-1.67724922094464));
#77538=CARTESIAN_POINT('Origin',(21.5,0.,0.));
#77539=CARTESIAN_POINT('',(21.8,-37.4643267032267,-1.63530568209482));
#77540=CARTESIAN_POINT('Ctrl Pts',(21.5,-37.7627704896084,-1.67724922094464));
#77541=CARTESIAN_POINT('Ctrl Pts',(21.6506031054658,-37.6129540886727,-1.65619389890503));
#77542=CARTESIAN_POINT('Ctrl Pts',(21.8,-37.4643267032267,-1.63530568209482));
#77543=CARTESIAN_POINT('',(21.8,-37.1791272503441,-4.89515034526194));
#77544=CARTESIAN_POINT('Ctrl Pts',(21.8,-37.4643267032267,-1.63530568209482));
#77545=CARTESIAN_POINT('Ctrl Pts',(21.8713861730393,-37.3217269767854,-3.26522801367838));
#77546=CARTESIAN_POINT('Ctrl Pts',(21.8,-37.1791272503441,-4.89515034526194));
#77547=CARTESIAN_POINT('',(21.5,-37.4803204240973,-4.90566824265506));
#77548=CARTESIAN_POINT('Ctrl Pts',(21.8,-37.1791272503441,-4.89515034526194));
#77549=CARTESIAN_POINT('Ctrl Pts',(21.6506031056359,-37.3291238524543,-4.90038834202877));
#77550=CARTESIAN_POINT('Ctrl Pts',(21.5,-37.4803204240973,-4.90566824265506));
#77551=CARTESIAN_POINT('',(21.5,-36.8978178826767,-8.209204315695));
#77552=CARTESIAN_POINT('Origin',(21.5,0.,0.));
#77553=CARTESIAN_POINT('',(21.8,-36.6111915470959,-8.11607377380573));
#77554=CARTESIAN_POINT('Ctrl Pts',(21.5,-36.8978178826767,-8.209204315695));
#77555=CARTESIAN_POINT('Ctrl Pts',(21.6506031086279,-36.7539337447878,-8.16245352531941));
#77556=CARTESIAN_POINT('Ctrl Pts',(21.8,-36.6111915470959,-8.11607377380573));
#77557=CARTESIAN_POINT('',(21.8,-35.764258829506,-11.2768697064435));
#77558=CARTESIAN_POINT('Ctrl Pts',(21.8,-36.6111915470959,-8.11607377380573));
#77559=CARTESIAN_POINT('Ctrl Pts',(21.8713861730394,-36.1877251883009,-9.69647174012462));
#77560=CARTESIAN_POINT('Ctrl Pts',(21.8,-35.764258829506,-11.2768697064435));
#77561=CARTESIAN_POINT('',(21.5,-36.0590497884573,-11.3395294590896));
#77562=CARTESIAN_POINT('Ctrl Pts',(21.8,-35.764258829506,-11.2768697064435));
#77563=CARTESIAN_POINT('Ctrl Pts',(21.6506031113732,-35.9110670719583,-11.308074761684));
#77564=CARTESIAN_POINT('Ctrl Pts',(21.5,-36.0590497884573,-11.3395294590896));
#77565=CARTESIAN_POINT('',(21.5,-34.9117437505765,-14.4917268913708));
#77566=CARTESIAN_POINT('Origin',(21.5,0.,0.));
#77567=CARTESIAN_POINT('',(21.8,-34.6456438619633,-14.3502390708311));
#77568=CARTESIAN_POINT('Ctrl Pts',(21.5,-34.9117437505765,-14.4917268913708));
#77569=CARTESIAN_POINT('Ctrl Pts',(21.6506031088497,-34.7781637254046,-14.4207011321053));
#77570=CARTESIAN_POINT('Ctrl Pts',(21.8,-34.6456438619633,-14.3502390708311));
#77571=CARTESIAN_POINT('',(21.8,-33.2627115017215,-17.3159470879662));
#77572=CARTESIAN_POINT('Ctrl Pts',(21.8,-34.6456438619633,-14.3502390708311));
#77573=CARTESIAN_POINT('Ctrl Pts',(21.8713861730394,-33.9541776818424,-15.8330930793986));
#77574=CARTESIAN_POINT('Ctrl Pts',(21.8,-33.2627115017215,-17.3159470879662));
#77575=CARTESIAN_POINT('',(21.5,-33.5421431717545,-17.4288448109885));
#77576=CARTESIAN_POINT('Ctrl Pts',(21.8,-33.2627115017215,-17.3159470879662));
#77577=CARTESIAN_POINT('Ctrl Pts',(21.6506031080477,-33.4018706992158,-17.3721710533201));
#77578=CARTESIAN_POINT('Ctrl Pts',(21.5,-33.5421431717545,-17.4288448109885));
#77579=CARTESIAN_POINT('',(21.5,-31.8648939508099,-20.3339256786199));
#77580=CARTESIAN_POINT('Origin',(21.5,0.,0.));
#77581=CARTESIAN_POINT('',(21.8,-31.6274058196267,-20.1483796152605));
#77582=CARTESIAN_POINT('Ctrl Pts',(21.5,-31.8648939508099,-20.3339256786199));
#77583=CARTESIAN_POINT('Ctrl Pts',(21.6506031077088,-31.7456768009401,-20.2407830329936));
#77584=CARTESIAN_POINT('Ctrl Pts',(21.8,-31.6274058196267,-20.1483796152605));
#77585=CARTESIAN_POINT('',(21.8,-29.7504935167013,-22.8288881795131));
#77586=CARTESIAN_POINT('Ctrl Pts',(21.8,-31.6274058196267,-20.1483796152605));
#77587=CARTESIAN_POINT('Ctrl Pts',(21.8713861730394,-30.688949668164,-21.4886338973868));
#77588=CARTESIAN_POINT('Ctrl Pts',(21.8,-29.7504935167013,-22.8288881795131));
#77589=CARTESIAN_POINT('',(21.5,-30.0060755079215,-22.9885935327265));
#77590=CARTESIAN_POINT('Ctrl Pts',(21.8,-29.7504935167013,-22.8288881795131));
#77591=CARTESIAN_POINT('Ctrl Pts',(21.6506031102095,-29.87777538233,-22.9084227163982));
#77592=CARTESIAN_POINT('Ctrl Pts',(21.5,-30.0060755079215,-22.9885935327265));
#77593=CARTESIAN_POINT('',(21.5,-27.8498454727622,-25.5582884235871));
#77594=CARTESIAN_POINT('Origin',(21.5,0.,0.));
#77595=CARTESIAN_POINT('',(21.8,-27.6481850557002,-25.3343218406523));
#77596=CARTESIAN_POINT('Ctrl Pts',(21.5,-27.8498454727622,-25.5582884235871));
#77597=CARTESIAN_POINT('Ctrl Pts',(21.6506031063136,-27.7486135508925,-25.4458589842583));
#77598=CARTESIAN_POINT('Ctrl Pts',(21.8,-27.6481850557002,-25.3343218406523));
#77599=CARTESIAN_POINT('',(21.8,-25.3343218406523,-27.6481850557002));
#77600=CARTESIAN_POINT('Ctrl Pts',(21.8,-27.6481850557002,-25.3343218406523));
#77601=CARTESIAN_POINT('Ctrl Pts',(21.8713861730393,-26.4912534481763,-26.4912534481763));
#77602=CARTESIAN_POINT('Ctrl Pts',(21.8,-25.3343218406523,-27.6481850557002));
#77603=CARTESIAN_POINT('',(21.5,-25.5582884235871,-27.8498454727622));
#77604=CARTESIAN_POINT('Ctrl Pts',(21.8,-25.3343218406523,-27.6481850557002));
#77605=CARTESIAN_POINT('Ctrl Pts',(21.6506031088795,-25.4458589823425,-27.7486135491675));
#77606=CARTESIAN_POINT('Ctrl Pts',(21.5,-25.5582884235871,-27.8498454727622));
#77607=CARTESIAN_POINT('',(21.5,-22.9885935327265,-30.0060755079215));
#77608=CARTESIAN_POINT('Origin',(21.5,0.,0.));
#77609=CARTESIAN_POINT('',(21.8,-22.8288881795131,-29.7504935167013));
#77610=CARTESIAN_POINT('Ctrl Pts',(21.5,-22.9885935327265,-30.0060755079215));
#77611=CARTESIAN_POINT('Ctrl Pts',(21.6506031103464,-22.9084227163254,-29.8777753822133));
#77612=CARTESIAN_POINT('Ctrl Pts',(21.8,-22.8288881795131,-29.7504935167013));
#77613=CARTESIAN_POINT('',(21.8,-20.1483796152605,-31.6274058196267));
#77614=CARTESIAN_POINT('Ctrl Pts',(21.8,-22.8288881795131,-29.7504935167013));
#77615=CARTESIAN_POINT('Ctrl Pts',(21.8713861730393,-21.4886338973868,-30.688949668164));
#77616=CARTESIAN_POINT('Ctrl Pts',(21.8,-20.1483796152605,-31.6274058196267));
#77617=CARTESIAN_POINT('',(21.5,-20.3339256786199,-31.8648939508099));
#77618=CARTESIAN_POINT('Ctrl Pts',(21.8,-20.1483796152605,-31.6274058196267));
#77619=CARTESIAN_POINT('Ctrl Pts',(21.6506031036307,-20.240783035516,-31.7456768041687));
#77620=CARTESIAN_POINT('Ctrl Pts',(21.5,-20.3339256786199,-31.8648939508099));
#77621=CARTESIAN_POINT('Origin',(21.5,0.,0.));
#77622=CARTESIAN_POINT('Origin',(0.,37.3,0.));
#77623=CARTESIAN_POINT('',(0.,-24.7364665672137,27.9176865404195));
#77624=CARTESIAN_POINT('Origin',(0.,0.,0.));
#77625=CARTESIAN_POINT('',(0.,-23.3271408859744,25.9049608779072));
#77626=CARTESIAN_POINT('',(0.,-9.96441562446309,6.82101143103729));
#77627=CARTESIAN_POINT('',(0.,-16.364348509518,30.7803605868911));
#77628=CARTESIAN_POINT('',(0.,-9.07210495534843,35.8864444939818));
#77629=CARTESIAN_POINT('',(0.,-17.7736741907572,32.7930862494034));
#77630=CARTESIAN_POINT('',(0.,-0.305813997156748,7.84639653186291));
#77631=CARTESIAN_POINT('',(6.93889390390723E-17,36.545659042501,7.46356517686174));
#77632=CARTESIAN_POINT('Origin',(0.,0.,0.));
#77633=CARTESIAN_POINT('',(0.,34.0979246472968,7.24941616595889));
#77634=CARTESIAN_POINT('',(0.,40.0542037481797,7.77052306408252));
#77635=CARTESIAN_POINT('',(0.,34.8387484606519,-1.21823876782095));
#77636=CARTESIAN_POINT('',(0.,34.4247983037968,3.51323317576981));
#77637=CARTESIAN_POINT('',(3.46944695195361E-17,37.2864828558561,-1.0040897569181));
#77638=CARTESIAN_POINT('',(0.,36.1129124805036,-1.10676386061131));
#77639=CARTESIAN_POINT('Origin',(0.,0.,0.));
#77640=CARTESIAN_POINT('',(0.,-34.,-4.163799117101E-15));
#77641=CARTESIAN_POINT('Origin',(0.,0.,0.));
#77642=CARTESIAN_POINT('Origin',(0.249999999999999,0.,0.));
#77643=CARTESIAN_POINT('',(0.499999999999998,-20.3339256786199,-31.8648939508099));
#77644=CARTESIAN_POINT('Origin',(0.499999999999998,0.,0.));
#77645=CARTESIAN_POINT('',(0.200000000000003,-20.1483796152605,-31.6274058196267));
#77646=CARTESIAN_POINT('Ctrl Pts',(0.500000000000002,-20.3339256786199,
-31.8648939508099));
#77647=CARTESIAN_POINT('Ctrl Pts',(0.349396891053132,-20.2407830322278,
-31.74567679996));
#77648=CARTESIAN_POINT('Ctrl Pts',(0.200000000000003,-20.1483796152605,
-31.6274058196267));
#77649=CARTESIAN_POINT('',(0.200000000000009,-22.8288881795131,-29.7504935167013));
#77650=CARTESIAN_POINT('Ctrl Pts',(0.200000000000003,-20.1483796152605,
-31.6274058196267));
#77651=CARTESIAN_POINT('Ctrl Pts',(0.12861382696065,-21.4886338973868,-30.688949668164));
#77652=CARTESIAN_POINT('Ctrl Pts',(0.200000000000009,-22.8288881795131,
-29.7504935167013));
#77653=CARTESIAN_POINT('',(0.499999999999998,-22.9885935327265,-30.0060755079215));
#77654=CARTESIAN_POINT('Ctrl Pts',(0.200000000000009,-22.8288881795131,
-29.7504935167013));
#77655=CARTESIAN_POINT('Ctrl Pts',(0.349396889603209,-22.9084227162985,
-29.8777753821704));
#77656=CARTESIAN_POINT('Ctrl Pts',(0.500000000000002,-22.9885935327265,
-30.0060755079215));
#77657=CARTESIAN_POINT('',(0.499999999999998,-25.5582884235871,-27.8498454727622));
#77658=CARTESIAN_POINT('Origin',(0.499999999999998,0.,0.));
#77659=CARTESIAN_POINT('',(0.200000000000009,-25.3343218406523,-27.6481850557002));
#77660=CARTESIAN_POINT('Ctrl Pts',(0.500000000000002,-25.5582884235871,
-27.8498454727622));
#77661=CARTESIAN_POINT('Ctrl Pts',(0.349396891196147,-25.445858982399,-27.7486135492184));
#77662=CARTESIAN_POINT('Ctrl Pts',(0.200000000000009,-25.3343218406523,
-27.6481850557002));
#77663=CARTESIAN_POINT('',(0.200000000000006,-27.6481850557002,-25.3343218406523));
#77664=CARTESIAN_POINT('Ctrl Pts',(0.200000000000009,-25.3343218406523,
-27.6481850557002));
#77665=CARTESIAN_POINT('Ctrl Pts',(0.128613826960649,-26.4912534481763,
-26.4912534481763));
#77666=CARTESIAN_POINT('Ctrl Pts',(0.200000000000006,-27.6481850557002,
-25.3343218406523));
#77667=CARTESIAN_POINT('',(0.499999999999998,-27.8498454727622,-25.5582884235871));
#77668=CARTESIAN_POINT('Ctrl Pts',(0.200000000000006,-27.6481850557002,
-25.3343218406523));
#77669=CARTESIAN_POINT('Ctrl Pts',(0.349396897552966,-27.7486135534918,
-25.4458589871452));
#77670=CARTESIAN_POINT('Ctrl Pts',(0.500000000000002,-27.8498454727622,
-25.5582884235871));
#77671=CARTESIAN_POINT('',(0.499999999999998,-30.0060755079215,-22.9885935327265));
#77672=CARTESIAN_POINT('Origin',(0.499999999999998,0.,0.));
#77673=CARTESIAN_POINT('',(0.200000000000003,-29.7504935167013,-22.8288881795131));
#77674=CARTESIAN_POINT('Ctrl Pts',(0.500000000000002,-30.0060755079215,
-22.9885935327265));
#77675=CARTESIAN_POINT('Ctrl Pts',(0.349396888618098,-29.8777753813311,
-22.9084227157741));
#77676=CARTESIAN_POINT('Ctrl Pts',(0.200000000000003,-29.7504935167013,
-22.8288881795131));
#77677=CARTESIAN_POINT('',(0.200000000000007,-31.6274058196267,-20.1483796152605));
#77678=CARTESIAN_POINT('Ctrl Pts',(0.200000000000003,-29.7504935167013,
-22.8288881795131));
#77679=CARTESIAN_POINT('Ctrl Pts',(0.128613826960649,-30.688949668164,-21.4886338973868));
#77680=CARTESIAN_POINT('Ctrl Pts',(0.200000000000007,-31.6274058196267,
-20.1483796152605));
#77681=CARTESIAN_POINT('',(0.499999999999998,-31.8648939508099,-20.3339256786199));
#77682=CARTESIAN_POINT('Ctrl Pts',(0.200000000000007,-31.6274058196267,
-20.1483796152605));
#77683=CARTESIAN_POINT('Ctrl Pts',(0.349396887455971,-31.7456767971121,
-20.2407830300028));
#77684=CARTESIAN_POINT('Ctrl Pts',(0.500000000000002,-31.8648939508099,
-20.3339256786199));
#77685=CARTESIAN_POINT('',(0.499999999999998,-33.5421431717545,-17.4288448109885));
#77686=CARTESIAN_POINT('Origin',(0.499999999999998,0.,0.));
#77687=CARTESIAN_POINT('',(0.200000000000004,-33.2627115017215,-17.3159470879662));
#77688=CARTESIAN_POINT('Ctrl Pts',(0.500000000000002,-33.5421431717545,
-17.4288448109885));
#77689=CARTESIAN_POINT('Ctrl Pts',(0.349396892668332,-33.4018706998828,
-17.3721710535896));
#77690=CARTESIAN_POINT('Ctrl Pts',(0.200000000000004,-33.2627115017215,
-17.3159470879662));
#77691=CARTESIAN_POINT('',(0.200000000000004,-34.6456438619633,-14.3502390708311));
#77692=CARTESIAN_POINT('Ctrl Pts',(0.200000000000004,-33.2627115017215,
-17.3159470879662));
#77693=CARTESIAN_POINT('Ctrl Pts',(0.128613826960645,-33.9541776818424,
-15.8330930793986));
#77694=CARTESIAN_POINT('Ctrl Pts',(0.200000000000004,-34.6456438619633,
-14.3502390708311));
#77695=CARTESIAN_POINT('',(0.499999999999998,-34.9117437505765,-14.4917268913708));
#77696=CARTESIAN_POINT('Ctrl Pts',(0.200000000000004,-34.6456438619633,
-14.3502390708311));
#77697=CARTESIAN_POINT('Ctrl Pts',(0.34939689516993,-34.7781637289703,-14.4207011340012));
#77698=CARTESIAN_POINT('Ctrl Pts',(0.500000000000002,-34.9117437505765,
-14.4917268913708));
#77699=CARTESIAN_POINT('',(0.499999999999998,-36.0590497884573,-11.3395294590896));
#77700=CARTESIAN_POINT('Origin',(0.499999999999998,0.,0.));
#77701=CARTESIAN_POINT('',(0.200000000000006,-35.764258829506,-11.2768697064435));
#77702=CARTESIAN_POINT('Ctrl Pts',(0.500000000000002,-36.0590497884573,
-11.3395294590896));
#77703=CARTESIAN_POINT('Ctrl Pts',(0.349396896306784,-35.9110670795055,
-11.3080747632882));
#77704=CARTESIAN_POINT('Ctrl Pts',(0.200000000000006,-35.764258829506,-11.2768697064435));
#77705=CARTESIAN_POINT('',(0.200000000000009,-36.6111915470959,-8.11607377380573));
#77706=CARTESIAN_POINT('Ctrl Pts',(0.200000000000006,-35.764258829506,-11.2768697064435));
#77707=CARTESIAN_POINT('Ctrl Pts',(0.128613826960652,-36.1877251883009,
-9.69647174012461));
#77708=CARTESIAN_POINT('Ctrl Pts',(0.200000000000009,-36.6111915470959,
-8.11607377380573));
#77709=CARTESIAN_POINT('',(0.499999999999998,-36.8978178826767,-8.209204315695));
#77710=CARTESIAN_POINT('Ctrl Pts',(0.200000000000009,-36.6111915470959,
-8.11607377380573));
#77711=CARTESIAN_POINT('Ctrl Pts',(0.349396891239299,-36.753933744661,-8.1624535252782));
#77712=CARTESIAN_POINT('Ctrl Pts',(0.500000000000002,-36.8978178826767,
-8.209204315695));
#77713=CARTESIAN_POINT('',(0.499999999999998,-37.4803204240973,-4.90566824265506));
#77714=CARTESIAN_POINT('Origin',(0.499999999999998,0.,0.));
#77715=CARTESIAN_POINT('',(0.200000000000002,-37.1791272503441,-4.89515034526194));
#77716=CARTESIAN_POINT('Ctrl Pts',(0.500000000000002,-37.4803204240973,
-4.90566824265506));
#77717=CARTESIAN_POINT('Ctrl Pts',(0.349396898001153,-37.3291238561062,
-4.9003883421563));
#77718=CARTESIAN_POINT('Ctrl Pts',(0.200000000000002,-37.1791272503441,
-4.89515034526194));
#77719=CARTESIAN_POINT('',(0.200000000000005,-37.4643267032267,-1.63530568209482));
#77720=CARTESIAN_POINT('Ctrl Pts',(0.200000000000002,-37.1791272503441,
-4.89515034526194));
#77721=CARTESIAN_POINT('Ctrl Pts',(0.128613826960647,-37.3217269767854,
-3.26522801367837));
#77722=CARTESIAN_POINT('Ctrl Pts',(0.200000000000005,-37.4643267032267,
-1.63530568209482));
#77723=CARTESIAN_POINT('',(0.499999999999998,-37.7627704896084,-1.67724922094464));
#77724=CARTESIAN_POINT('Ctrl Pts',(0.200000000000005,-37.4643267032267,
-1.63530568209482));
#77725=CARTESIAN_POINT('Ctrl Pts',(0.34939689448424,-37.6129540886231,-1.65619389889805));
#77726=CARTESIAN_POINT('Ctrl Pts',(0.500000000000002,-37.7627704896084,
-1.67724922094464));
#77727=CARTESIAN_POINT('',(0.499999999999998,-37.7627704896084,1.67724922094466));
#77728=CARTESIAN_POINT('Origin',(0.499999999999998,0.,0.));
#77729=CARTESIAN_POINT('',(0.200000000000009,-37.4643267032267,1.63530568209484));
#77730=CARTESIAN_POINT('Ctrl Pts',(0.500000000000002,-37.7627704896084,
1.67724922094466));
#77731=CARTESIAN_POINT('Ctrl Pts',(0.349396890810879,-37.6129540849685,
1.65619389838445));
#77732=CARTESIAN_POINT('Ctrl Pts',(0.200000000000009,-37.4643267032267,
1.63530568209484));
#77733=CARTESIAN_POINT('',(0.200000000000002,-37.1791272503441,4.89515034526196));
#77734=CARTESIAN_POINT('Ctrl Pts',(0.200000000000009,-37.4643267032267,
1.63530568209484));
#77735=CARTESIAN_POINT('Ctrl Pts',(0.128613826960646,-37.3217269767854,
3.2652280136784));
#77736=CARTESIAN_POINT('Ctrl Pts',(0.200000000000002,-37.1791272503441,
4.89515034526196));
#77737=CARTESIAN_POINT('',(0.499999999999998,-37.4803204240973,4.90566824265508));
#77738=CARTESIAN_POINT('Ctrl Pts',(0.200000000000002,-37.1791272503441,
4.89515034526196));
#77739=CARTESIAN_POINT('Ctrl Pts',(0.349396890635592,-37.3291238487107,
4.90038834189806));
#77740=CARTESIAN_POINT('Ctrl Pts',(0.500000000000002,-37.4803204240973,
4.90566824265508));
#77741=CARTESIAN_POINT('',(0.499999999999998,-36.8978178826767,8.20920431569502));
#77742=CARTESIAN_POINT('Origin',(0.499999999999998,0.,0.));
#77743=CARTESIAN_POINT('',(0.200000000000009,-36.6111915470959,8.11607377380575));
#77744=CARTESIAN_POINT('Ctrl Pts',(0.500000000000001,-36.8978178826767,
8.20920431569502));
#77745=CARTESIAN_POINT('Ctrl Pts',(0.349396891227683,-36.7539337446499,
8.16245352527461));
#77746=CARTESIAN_POINT('Ctrl Pts',(0.200000000000009,-36.6111915470959,
8.11607377380575));
#77747=CARTESIAN_POINT('',(0.20000000000001,-35.764258829506,11.2768697064435));
#77748=CARTESIAN_POINT('Ctrl Pts',(0.200000000000009,-36.6111915470959,
8.11607377380575));
#77749=CARTESIAN_POINT('Ctrl Pts',(0.12861382696065,-36.1877251883009,9.69647174012464));
#77750=CARTESIAN_POINT('Ctrl Pts',(0.20000000000001,-35.764258829506,11.2768697064435));
#77751=CARTESIAN_POINT('',(0.499999999999998,-36.0590497884572,11.3395294590896));
#77752=CARTESIAN_POINT('Ctrl Pts',(0.20000000000001,-35.764258829506,11.2768697064435));
#77753=CARTESIAN_POINT('Ctrl Pts',(0.349396892541906,-35.9110670758057,
11.3080747625018));
#77754=CARTESIAN_POINT('Ctrl Pts',(0.500000000000002,-36.0590497884573,
11.3395294590896));
#77755=CARTESIAN_POINT('',(0.499999999999998,-34.9117437505765,14.4917268913708));
#77756=CARTESIAN_POINT('Origin',(0.499999999999998,0.,0.));
#77757=CARTESIAN_POINT('',(0.200000000000008,-34.6456438619633,14.3502390708311));
#77758=CARTESIAN_POINT('Ctrl Pts',(0.500000000000001,-34.9117437505765,
14.4917268913708));
#77759=CARTESIAN_POINT('Ctrl Pts',(0.349396895264272,-34.778163729054,14.4207011340457));
#77760=CARTESIAN_POINT('Ctrl Pts',(0.200000000000008,-34.6456438619633,
14.3502390708311));
#77761=CARTESIAN_POINT('',(0.200000000000004,-33.2627115017215,17.3159470879662));
#77762=CARTESIAN_POINT('Ctrl Pts',(0.200000000000008,-34.6456438619633,
14.3502390708311));
#77763=CARTESIAN_POINT('Ctrl Pts',(0.128613826960644,-33.9541776818424,
15.8330930793986));
#77764=CARTESIAN_POINT('Ctrl Pts',(0.200000000000004,-33.2627115017215,
17.3159470879662));
#77765=CARTESIAN_POINT('',(0.499999999999998,-33.5421431717545,17.4288448109885));
#77766=CARTESIAN_POINT('Ctrl Pts',(0.200000000000004,-33.2627115017215,
17.3159470879662));
#77767=CARTESIAN_POINT('Ctrl Pts',(0.349396887767451,-33.4018706953176,
17.3721710517451));
#77768=CARTESIAN_POINT('Ctrl Pts',(0.500000000000001,-33.5421431717545,
17.4288448109885));
#77769=CARTESIAN_POINT('',(0.499999999999998,-31.8648939508099,20.3339256786199));
#77770=CARTESIAN_POINT('Origin',(0.499999999999998,0.,0.));
#77771=CARTESIAN_POINT('',(0.200000000000003,-31.6274058196267,20.1483796152605));
#77772=CARTESIAN_POINT('Ctrl Pts',(0.500000000000001,-31.8648939508099,
20.3339256786199));
#77773=CARTESIAN_POINT('Ctrl Pts',(0.349396891074454,-31.7456767999768,
20.240783032241));
#77774=CARTESIAN_POINT('Ctrl Pts',(0.200000000000003,-31.6274058196267,
20.1483796152605));
#77775=CARTESIAN_POINT('',(0.200000000000009,-29.7504935167013,22.8288881795131));
#77776=CARTESIAN_POINT('Ctrl Pts',(0.200000000000003,-31.6274058196267,
20.1483796152605));
#77777=CARTESIAN_POINT('Ctrl Pts',(0.128613826960651,-30.688949668164,21.4886338973868));
#77778=CARTESIAN_POINT('Ctrl Pts',(0.200000000000009,-29.7504935167013,
22.8288881795131));
#77779=CARTESIAN_POINT('',(0.499999999999998,-30.0060755079215,22.9885935327265));
#77780=CARTESIAN_POINT('Ctrl Pts',(0.200000000000009,-29.7504935167013,
22.8288881795131));
#77781=CARTESIAN_POINT('Ctrl Pts',(0.349396889570691,-29.8777753821427,
22.9084227162812));
#77782=CARTESIAN_POINT('Ctrl Pts',(0.500000000000001,-30.0060755079215,
22.9885935327265));
#77783=CARTESIAN_POINT('',(0.499999999999998,-27.8498454727622,25.5582884235871));
#77784=CARTESIAN_POINT('Origin',(0.499999999999998,0.,0.));
#77785=CARTESIAN_POINT('',(0.200000000000006,-27.6481850557002,25.3343218406523));
#77786=CARTESIAN_POINT('Ctrl Pts',(0.500000000000001,-27.8498454727622,
25.5582884235871));
#77787=CARTESIAN_POINT('Ctrl Pts',(0.349396893632768,-27.7486135508564,
25.4458589842183));
#77788=CARTESIAN_POINT('Ctrl Pts',(0.200000000000006,-27.6481850557002,
25.3343218406523));
#77789=CARTESIAN_POINT('',(0.200000000000006,-25.3343218406523,27.6481850557002));
#77790=CARTESIAN_POINT('Ctrl Pts',(0.200000000000006,-27.6481850557002,
25.3343218406523));
#77791=CARTESIAN_POINT('Ctrl Pts',(0.128613826960647,-26.4912534481763,
26.4912534481763));
#77792=CARTESIAN_POINT('Ctrl Pts',(0.200000000000006,-25.3343218406523,
27.6481850557002));
#77793=CARTESIAN_POINT('',(0.499999999999998,-25.5582884235871,27.8498454727622));
#77794=CARTESIAN_POINT('Ctrl Pts',(0.200000000000006,-25.3343218406523,
27.6481850557002));
#77795=CARTESIAN_POINT('Ctrl Pts',(0.349396893895724,-25.4458589844146,
27.7486135510332));
#77796=CARTESIAN_POINT('Ctrl Pts',(0.500000000000001,-25.5582884235871,
27.8498454727622));
#77797=CARTESIAN_POINT('',(0.499999999999998,-25.0251096245113,28.3299115473591));
#77798=CARTESIAN_POINT('Origin',(0.499999999999998,0.,0.));
#77799=CARTESIAN_POINT('Ctrl Pts',(0.500000000000004,-25.0251096245113,
28.3299115473591));
#77800=CARTESIAN_POINT('Ctrl Pts',(0.248313951856147,-24.8798272328718,
28.1224267893243));
#77801=CARTESIAN_POINT('Ctrl Pts',(-2.08166817117217E-16,-24.7364665672137,
27.9176865404195));
#77802=CARTESIAN_POINT('Origin',(0.249999999999999,0.,0.));
#77803=CARTESIAN_POINT('',(0.499999999999998,37.7878017125899,-0.960230040142118));
#77804=CARTESIAN_POINT('Ctrl Pts',(1.04083408558608E-16,37.2864828558561,
-1.0040897569181));
#77805=CARTESIAN_POINT('Ctrl Pts',(0.248313954120435,37.5354734476842,-0.982305902808531));
#77806=CARTESIAN_POINT('Ctrl Pts',(0.500000000000005,37.7878017125899,-0.960230040142117));
#77807=CARTESIAN_POINT('',(0.499999999999998,37.7627704896084,-1.67724922094465));
#77808=CARTESIAN_POINT('Origin',(0.499999999999998,0.,0.));
#77809=CARTESIAN_POINT('',(0.200000000000005,37.4643267032267,-1.63530568209483));
#77810=CARTESIAN_POINT('Ctrl Pts',(0.500000000000005,37.7627704896084,-1.67724922094465));
#77811=CARTESIAN_POINT('Ctrl Pts',(0.349396890677128,37.6129540848354,-1.65619389836574));
#77812=CARTESIAN_POINT('Ctrl Pts',(0.200000000000005,37.4643267032267,-1.63530568209483));
#77813=CARTESIAN_POINT('',(0.200000000000002,37.1791272503441,-4.89515034526195));
#77814=CARTESIAN_POINT('Ctrl Pts',(0.200000000000005,37.4643267032267,-1.63530568209483));
#77815=CARTESIAN_POINT('Ctrl Pts',(0.128613826960643,37.3217269767854,-3.26522801367839));
#77816=CARTESIAN_POINT('Ctrl Pts',(0.200000000000002,37.1791272503441,-4.89515034526195));
#77817=CARTESIAN_POINT('',(0.499999999999998,37.4803204240973,-4.90566824265507));
#77818=CARTESIAN_POINT('Ctrl Pts',(0.200000000000002,37.1791272503441,-4.89515034526194));
#77819=CARTESIAN_POINT('Ctrl Pts',(0.349396890484736,37.3291238485592,-4.90038834189276));
#77820=CARTESIAN_POINT('Ctrl Pts',(0.500000000000004,37.4803204240973,-4.90566824265507));
#77821=CARTESIAN_POINT('',(0.499999999999998,36.8978178826767,-8.20920431569504));
#77822=CARTESIAN_POINT('Origin',(0.499999999999998,0.,0.));
#77823=CARTESIAN_POINT('',(0.200000000000008,36.6111915470958,-8.11607377380577));
#77824=CARTESIAN_POINT('Ctrl Pts',(0.500000000000004,36.8978178826767,-8.20920431569504));
#77825=CARTESIAN_POINT('Ctrl Pts',(0.349396891393874,36.7539337448086,-8.16245352532623));
#77826=CARTESIAN_POINT('Ctrl Pts',(0.200000000000008,36.6111915470958,-8.11607377380577));
#77827=CARTESIAN_POINT('',(0.200000000000001,35.764258829506,-11.2768697064435));
#77828=CARTESIAN_POINT('Ctrl Pts',(0.200000000000008,36.6111915470958,-8.11607377380577));
#77829=CARTESIAN_POINT('Ctrl Pts',(0.128613826960642,36.1877251883009,-9.69647174012466));
#77830=CARTESIAN_POINT('Ctrl Pts',(0.200000000000001,35.764258829506,-11.2768697064435));
#77831=CARTESIAN_POINT('',(0.499999999999998,36.0590497884572,-11.3395294590896));
#77832=CARTESIAN_POINT('Ctrl Pts',(0.200000000000001,35.764258829506,-11.2768697064435));
#77833=CARTESIAN_POINT('Ctrl Pts',(0.349396888726257,35.911067072056,-11.3080747617048));
#77834=CARTESIAN_POINT('Ctrl Pts',(0.500000000000004,36.0590497884572,-11.3395294590896));
#77835=CARTESIAN_POINT('',(0.499999999999998,34.9117437505765,-14.4917268913708));
#77836=CARTESIAN_POINT('Origin',(0.499999999999998,0.,0.));
#77837=CARTESIAN_POINT('',(0.200000000000003,34.6456438619633,-14.3502390708311));
#77838=CARTESIAN_POINT('Ctrl Pts',(0.500000000000004,34.9117437505765,-14.4917268913708));
#77839=CARTESIAN_POINT('Ctrl Pts',(0.349396890191469,34.7781637245541,-14.4207011316531));
#77840=CARTESIAN_POINT('Ctrl Pts',(0.200000000000003,34.6456438619633,-14.3502390708311));
#77841=CARTESIAN_POINT('',(0.200000000000004,33.2627115017215,-17.3159470879662));
#77842=CARTESIAN_POINT('Ctrl Pts',(0.200000000000003,34.6456438619633,-14.3502390708311));
#77843=CARTESIAN_POINT('Ctrl Pts',(0.128613826960647,33.9541776818424,-15.8330930793987));
#77844=CARTESIAN_POINT('Ctrl Pts',(0.200000000000004,33.2627115017215,-17.3159470879662));
#77845=CARTESIAN_POINT('',(0.499999999999998,33.5421431717545,-17.4288448109885));
#77846=CARTESIAN_POINT('Ctrl Pts',(0.200000000000004,33.2627115017215,-17.3159470879662));
#77847=CARTESIAN_POINT('Ctrl Pts',(0.349396888098001,33.4018706956255,-17.3721710518695));
#77848=CARTESIAN_POINT('Ctrl Pts',(0.500000000000004,33.5421431717545,-17.4288448109885));
#77849=CARTESIAN_POINT('',(0.499999999999998,31.8648939508099,-20.3339256786199));
#77850=CARTESIAN_POINT('Origin',(0.499999999999998,0.,0.));
#77851=CARTESIAN_POINT('',(0.199999999999999,31.6274058196267,-20.1483796152605));
#77852=CARTESIAN_POINT('Ctrl Pts',(0.500000000000004,31.8648939508099,-20.3339256786199));
#77853=CARTESIAN_POINT('Ctrl Pts',(0.349396893153553,31.7456768016228,-20.240783033527));
#77854=CARTESIAN_POINT('Ctrl Pts',(0.199999999999999,31.6274058196267,-20.1483796152605));
#77855=CARTESIAN_POINT('',(0.200000000000003,29.7504935167013,-22.8288881795131));
#77856=CARTESIAN_POINT('Ctrl Pts',(0.199999999999999,31.6274058196267,-20.1483796152605));
#77857=CARTESIAN_POINT('Ctrl Pts',(0.128613826960646,30.688949668164,-21.4886338973868));
#77858=CARTESIAN_POINT('Ctrl Pts',(0.200000000000003,29.7504935167013,-22.8288881795131));
#77859=CARTESIAN_POINT('',(0.499999999999998,30.0060755079215,-22.9885935327265));
#77860=CARTESIAN_POINT('Ctrl Pts',(0.200000000000003,29.7504935167013,-22.8288881795131));
#77861=CARTESIAN_POINT('Ctrl Pts',(0.34939689381316,29.8777753857573,-22.9084227185399));
#77862=CARTESIAN_POINT('Ctrl Pts',(0.500000000000003,30.0060755079215,-22.9885935327265));
#77863=CARTESIAN_POINT('',(0.499999999999998,27.8498454727622,-25.5582884235871));
#77864=CARTESIAN_POINT('Origin',(0.499999999999998,0.,0.));
#77865=CARTESIAN_POINT('',(0.2,27.6481850557002,-25.3343218406523));
#77866=CARTESIAN_POINT('Ctrl Pts',(0.500000000000003,27.8498454727622,-25.5582884235871));
#77867=CARTESIAN_POINT('Ctrl Pts',(0.34939689386556,27.7486135510129,-25.4458589843921));
#77868=CARTESIAN_POINT('Ctrl Pts',(0.2,27.6481850557002,-25.3343218406523));
#77869=CARTESIAN_POINT('',(0.200000000000006,25.3343218406523,-27.6481850557003));
#77870=CARTESIAN_POINT('Ctrl Pts',(0.2,27.6481850557002,-25.3343218406523));
#77871=CARTESIAN_POINT('Ctrl Pts',(0.128613826960646,26.4912534481763,-26.4912534481763));
#77872=CARTESIAN_POINT('Ctrl Pts',(0.200000000000006,25.3343218406523,-27.6481850557003));
#77873=CARTESIAN_POINT('',(0.499999999999998,25.5582884235871,-27.8498454727622));
#77874=CARTESIAN_POINT('Ctrl Pts',(0.200000000000006,25.3343218406523,-27.6481850557003));
#77875=CARTESIAN_POINT('Ctrl Pts',(0.34939689385293,25.4458589843826,-27.7486135510044));
#77876=CARTESIAN_POINT('Ctrl Pts',(0.500000000000003,25.5582884235871,-27.8498454727622));
#77877=CARTESIAN_POINT('',(0.499999999999998,22.9885935327265,-30.0060755079215));
#77878=CARTESIAN_POINT('Origin',(0.499999999999998,0.,0.));
#77879=CARTESIAN_POINT('',(0.200000000000003,22.8288881795131,-29.7504935167013));
#77880=CARTESIAN_POINT('Ctrl Pts',(0.500000000000003,22.9885935327265,-30.0060755079215));
#77881=CARTESIAN_POINT('Ctrl Pts',(0.349396892499578,22.9084227178406,-29.8777753846381));
#77882=CARTESIAN_POINT('Ctrl Pts',(0.200000000000003,22.8288881795131,-29.7504935167013));
#77883=CARTESIAN_POINT('',(0.200000000000009,20.1483796152605,-31.6274058196267));
#77884=CARTESIAN_POINT('Ctrl Pts',(0.200000000000003,22.8288881795131,-29.7504935167013));
#77885=CARTESIAN_POINT('Ctrl Pts',(0.128613826960651,21.4886338973868,-30.688949668164));
#77886=CARTESIAN_POINT('Ctrl Pts',(0.200000000000009,20.1483796152605,-31.6274058196267));
#77887=CARTESIAN_POINT('',(0.499999999999998,20.3339256786199,-31.8648939508099));
#77888=CARTESIAN_POINT('Ctrl Pts',(0.200000000000009,20.1483796152605,-31.6274058196267));
#77889=CARTESIAN_POINT('Ctrl Pts',(0.349396892229315,20.2407830329553,-31.7456768008911));
#77890=CARTESIAN_POINT('Ctrl Pts',(0.500000000000003,20.3339256786199,-31.8648939508099));
#77891=CARTESIAN_POINT('',(0.499999999999998,17.4288448109885,-33.5421431717545));
#77892=CARTESIAN_POINT('Origin',(0.499999999999998,0.,0.));
#77893=CARTESIAN_POINT('',(0.200000000000008,17.3159470879662,-33.2627115017215));
#77894=CARTESIAN_POINT('Ctrl Pts',(0.500000000000003,17.4288448109885,-33.5421431717546));
#77895=CARTESIAN_POINT('Ctrl Pts',(0.349396892187316,17.3721710534085,-33.4018706994348));
#77896=CARTESIAN_POINT('Ctrl Pts',(0.200000000000008,17.3159470879662,-33.2627115017215));
#77897=CARTESIAN_POINT('',(0.200000000000009,14.350239070831,-34.6456438619633));
#77898=CARTESIAN_POINT('Ctrl Pts',(0.200000000000008,17.3159470879662,-33.2627115017215));
#77899=CARTESIAN_POINT('Ctrl Pts',(0.128613826960651,15.8330930793986,-33.9541776818424));
#77900=CARTESIAN_POINT('Ctrl Pts',(0.200000000000009,14.350239070831,-34.6456438619633));
#77901=CARTESIAN_POINT('',(0.499999999999998,14.4917268913708,-34.9117437505765));
#77902=CARTESIAN_POINT('Ctrl Pts',(0.200000000000009,14.350239070831,-34.6456438619633));
#77903=CARTESIAN_POINT('Ctrl Pts',(0.349396890607192,14.4207011318491,-34.7781637249228));
#77904=CARTESIAN_POINT('Ctrl Pts',(0.500000000000003,14.4917268913708,-34.9117437505765));
#77905=CARTESIAN_POINT('',(0.499999999999998,11.3395294590896,-36.0590497884573));
#77906=CARTESIAN_POINT('Origin',(0.499999999999998,0.,0.));
#77907=CARTESIAN_POINT('',(0.200000000000006,11.2768697064435,-35.764258829506));
#77908=CARTESIAN_POINT('Ctrl Pts',(0.500000000000003,11.3395294590896,-36.0590497884573));
#77909=CARTESIAN_POINT('Ctrl Pts',(0.349396892569828,11.3080747625076,-35.9110670758332));
#77910=CARTESIAN_POINT('Ctrl Pts',(0.200000000000006,11.2768697064435,-35.764258829506));
#77911=CARTESIAN_POINT('',(0.200000000000008,8.11607377380573,-36.6111915470959));
#77912=CARTESIAN_POINT('Ctrl Pts',(0.200000000000006,11.2768697064435,-35.764258829506));
#77913=CARTESIAN_POINT('Ctrl Pts',(0.128613826960652,9.69647174012461,-36.1877251883009));
#77914=CARTESIAN_POINT('Ctrl Pts',(0.200000000000009,8.11607377380573,-36.6111915470959));
#77915=CARTESIAN_POINT('',(0.499999999999998,8.209204315695,-36.8978178826767));
#77916=CARTESIAN_POINT('Ctrl Pts',(0.200000000000008,8.11607377380573,-36.6111915470959));
#77917=CARTESIAN_POINT('Ctrl Pts',(0.349396891147052,8.16245352524956,-36.7539337445728));
#77918=CARTESIAN_POINT('Ctrl Pts',(0.500000000000003,8.209204315695,-36.8978178826767));
#77919=CARTESIAN_POINT('',(0.499999999999998,4.90566824265506,-37.4803204240973));
#77920=CARTESIAN_POINT('Origin',(0.499999999999998,0.,0.));
#77921=CARTESIAN_POINT('',(0.200000000000002,4.89515034526193,-37.1791272503441));
#77922=CARTESIAN_POINT('Ctrl Pts',(0.500000000000003,4.90566824265506,-37.4803204240973));
#77923=CARTESIAN_POINT('Ctrl Pts',(0.349396890683097,4.90038834189971,-37.3291238487584));
#77924=CARTESIAN_POINT('Ctrl Pts',(0.200000000000002,4.89515034526193,-37.1791272503441));
#77925=CARTESIAN_POINT('',(0.200000000000005,1.63530568209482,-37.4643267032267));
#77926=CARTESIAN_POINT('Ctrl Pts',(0.200000000000002,4.89515034526193,-37.1791272503441));
#77927=CARTESIAN_POINT('Ctrl Pts',(0.128613826960647,3.26522801367837,-37.3217269767854));
#77928=CARTESIAN_POINT('Ctrl Pts',(0.200000000000005,1.63530568209482,-37.4643267032267));
#77929=CARTESIAN_POINT('',(0.499999999999998,1.67724922094464,-37.7627704896084));
#77930=CARTESIAN_POINT('Ctrl Pts',(0.200000000000005,1.63530568209482,-37.4643267032267));
#77931=CARTESIAN_POINT('Ctrl Pts',(0.34939689445096,1.6561938988934,-37.61295408859));
#77932=CARTESIAN_POINT('Ctrl Pts',(0.500000000000003,1.67724922094464,-37.7627704896084));
#77933=CARTESIAN_POINT('',(0.499999999999998,-1.67724922094465,-37.7627704896084));
#77934=CARTESIAN_POINT('Origin',(0.499999999999998,0.,0.));
#77935=CARTESIAN_POINT('',(0.200000000000005,-1.63530568209482,-37.4643267032267));
#77936=CARTESIAN_POINT('Ctrl Pts',(0.500000000000003,-1.67724922094465,
-37.7627704896084));
#77937=CARTESIAN_POINT('Ctrl Pts',(0.349396890783986,-1.65619389838068,
-37.6129540849417));
#77938=CARTESIAN_POINT('Ctrl Pts',(0.200000000000005,-1.63530568209482,
-37.4643267032267));
#77939=CARTESIAN_POINT('',(0.200000000000002,-4.89515034526194,-37.1791272503441));
#77940=CARTESIAN_POINT('Ctrl Pts',(0.200000000000005,-1.63530568209482,
-37.4643267032267));
#77941=CARTESIAN_POINT('Ctrl Pts',(0.128613826960644,-3.26522801367839,
-37.3217269767854));
#77942=CARTESIAN_POINT('Ctrl Pts',(0.200000000000002,-4.89515034526194,
-37.1791272503441));
#77943=CARTESIAN_POINT('',(0.499999999999998,-4.90566824265507,-37.4803204240973));
#77944=CARTESIAN_POINT('Ctrl Pts',(0.200000000000002,-4.89515034526194,
-37.1791272503441));
#77945=CARTESIAN_POINT('Ctrl Pts',(0.349396894243145,-4.90038834202454,
-37.3291238523329));
#77946=CARTESIAN_POINT('Ctrl Pts',(0.500000000000003,-4.90566824265507,
-37.4803204240973));
#77947=CARTESIAN_POINT('',(0.499999999999998,-8.20920431569503,-36.8978178826767));
#77948=CARTESIAN_POINT('Origin',(0.499999999999998,0.,0.));
#77949=CARTESIAN_POINT('',(0.200000000000013,-8.11607377380577,-36.6111915470959));
#77950=CARTESIAN_POINT('Ctrl Pts',(0.500000000000003,-8.20920431569504,
-36.8978178826767));
#77951=CARTESIAN_POINT('Ctrl Pts',(0.349396891427038,-8.16245352533653,
-36.7539337448403));
#77952=CARTESIAN_POINT('Ctrl Pts',(0.200000000000013,-8.11607377380577,
-36.6111915470959));
#77953=CARTESIAN_POINT('',(0.200000000000006,-11.2768697064435,-35.764258829506));
#77954=CARTESIAN_POINT('Ctrl Pts',(0.200000000000013,-8.11607377380577,
-36.6111915470959));
#77955=CARTESIAN_POINT('Ctrl Pts',(0.12861382696065,-9.69647174012466,-36.1877251883009));
#77956=CARTESIAN_POINT('Ctrl Pts',(0.200000000000006,-11.2768697064435,
-35.764258829506));
#77957=CARTESIAN_POINT('Ctrl Pts',(0.200000000000006,-11.2768697064435,
-35.764258829506));
#77958=CARTESIAN_POINT('Ctrl Pts',(0.349396892466969,-11.3080747624862,
-35.9110670757321));
#77959=CARTESIAN_POINT('Ctrl Pts',(0.500000000000002,-11.3395294590896,
-36.0590497884572));
#77960=CARTESIAN_POINT('Origin',(0.,-28.7187593876742,33.6049900942237));
#77961=CARTESIAN_POINT('',(22.,-23.3271408859744,25.9049608779072));
#77962=CARTESIAN_POINT('',(22.,-10.5072490062194,7.59625784318566));
#77963=CARTESIAN_POINT('',(0.,-23.3271408859744,25.9049608779072));
#77964=CARTESIAN_POINT('',(11.,-25.0251096245113,28.3299115473591));
#77965=CARTESIAN_POINT('Origin',(0.,-16.364348509518,30.7803605868911));
#77966=CARTESIAN_POINT('',(21.5,-18.0623172480549,33.205311256343));
#77967=CARTESIAN_POINT('',(22.,-17.7736741907572,32.7930862494034));
#77968=CARTESIAN_POINT('Ctrl Pts',(21.5,-18.0623172480549,33.205311256343));
#77969=CARTESIAN_POINT('Ctrl Pts',(21.7516860460885,-17.9170348576018,32.9978265000027));
#77970=CARTESIAN_POINT('Ctrl Pts',(22.,-17.7736741907572,32.7930862494034));
#77971=CARTESIAN_POINT('',(0.499999999999998,-18.0623172480549,33.205311256343));
#77972=CARTESIAN_POINT('',(11.,-18.0623172480549,33.205311256343));
#77973=CARTESIAN_POINT('Ctrl Pts',(3.12250225675825E-16,-17.7736741907572,
32.7930862494034));
#77974=CARTESIAN_POINT('Ctrl Pts',(0.248313958347431,-17.9170348601627,
32.99782650366));
#77975=CARTESIAN_POINT('Ctrl Pts',(0.500000000000005,-18.0623172480549,
33.205311256343));
#77976=CARTESIAN_POINT('',(22.,-16.364348509518,30.7803605868911));
#77977=CARTESIAN_POINT('',(0.,-16.364348509518,30.7803605868911));
#77978=CARTESIAN_POINT('',(22.,-0.848647378913067,8.62164294401129));
#77979=CARTESIAN_POINT('Origin',(0.,-23.3271408859744,25.9049608779072));
#77980=CARTESIAN_POINT('',(22.,-10.1792715735921,35.1111980818334));
#77981=CARTESIAN_POINT('Origin',(21.75,0.,0.));
#77982=CARTESIAN_POINT('',(22.,36.545659042501,7.46356517686174));
#77983=CARTESIAN_POINT('Origin',(22.,0.,0.));
#77984=CARTESIAN_POINT('',(21.5,37.0469778992348,7.50742489363772));
#77985=CARTESIAN_POINT('Ctrl Pts',(22.,36.545659042501,7.46356517686174));
#77986=CARTESIAN_POINT('Ctrl Pts',(21.7516860406108,36.7946496396117,7.48534903143347));
#77987=CARTESIAN_POINT('Ctrl Pts',(21.5,37.0469778992348,7.50742489363772));
#77988=CARTESIAN_POINT('',(21.5,36.8978178826767,8.20920431569501));
#77989=CARTESIAN_POINT('Origin',(21.5,0.,0.));
#77990=CARTESIAN_POINT('',(21.8,36.6111915470959,8.11607377380574));
#77991=CARTESIAN_POINT('Ctrl Pts',(21.5,36.8978178826767,8.20920431569501));
#77992=CARTESIAN_POINT('Ctrl Pts',(21.6506031085866,36.7539337448273,8.16245352533225));
#77993=CARTESIAN_POINT('Ctrl Pts',(21.8,36.6111915470959,8.11607377380574));
#77994=CARTESIAN_POINT('',(21.8,35.764258829506,11.2768697064435));
#77995=CARTESIAN_POINT('Ctrl Pts',(21.8,36.6111915470959,8.11607377380574));
#77996=CARTESIAN_POINT('Ctrl Pts',(21.8713861730393,36.1877251883009,9.69647174012463));
#77997=CARTESIAN_POINT('Ctrl Pts',(21.8,35.764258829506,11.2768697064435));
#77998=CARTESIAN_POINT('',(21.5,36.0590497884573,11.3395294590896));
#77999=CARTESIAN_POINT('Ctrl Pts',(21.8,35.764258829506,11.2768697064435));
#78000=CARTESIAN_POINT('Ctrl Pts',(21.6506031072715,35.9110670759891,11.3080747625408));
#78001=CARTESIAN_POINT('Ctrl Pts',(21.5,36.0590497884573,11.3395294590896));
#78002=CARTESIAN_POINT('',(21.5,34.9117437505765,14.4917268913708));
#78003=CARTESIAN_POINT('Origin',(21.5,0.,0.));
#78004=CARTESIAN_POINT('',(21.8,34.6456438619633,14.3502390708311));
#78005=CARTESIAN_POINT('Ctrl Pts',(21.5,34.9117437505765,14.4917268913708));
#78006=CARTESIAN_POINT('Ctrl Pts',(21.6506031059505,34.7781637279764,14.4207011334727));
#78007=CARTESIAN_POINT('Ctrl Pts',(21.8,34.6456438619633,14.3502390708311));
#78008=CARTESIAN_POINT('',(21.8,33.2627115017215,17.3159470879662));
#78009=CARTESIAN_POINT('Ctrl Pts',(21.8,34.6456438619633,14.3502390708311));
#78010=CARTESIAN_POINT('Ctrl Pts',(21.8713861730394,33.9541776818424,15.8330930793986));
#78011=CARTESIAN_POINT('Ctrl Pts',(21.8,33.2627115017215,17.3159470879662));
#78012=CARTESIAN_POINT('',(21.5,33.5421431717545,17.4288448109885));
#78013=CARTESIAN_POINT('Ctrl Pts',(21.8,33.2627115017215,17.3159470879662));
#78014=CARTESIAN_POINT('Ctrl Pts',(21.650603107741,33.4018706995015,17.3721710534355));
#78015=CARTESIAN_POINT('Ctrl Pts',(21.5,33.5421431717545,17.4288448109885));
#78016=CARTESIAN_POINT('',(21.5,31.8648939508099,20.3339256786199));
#78017=CARTESIAN_POINT('Origin',(21.5,0.,0.));
#78018=CARTESIAN_POINT('',(21.8,31.6274058196267,20.1483796152605));
#78019=CARTESIAN_POINT('Ctrl Pts',(21.5,31.8648939508099,20.3339256786199));
#78020=CARTESIAN_POINT('Ctrl Pts',(21.6506031088134,31.7456768000656,20.2407830323103));
#78021=CARTESIAN_POINT('Ctrl Pts',(21.8,31.6274058196267,20.1483796152605));
#78022=CARTESIAN_POINT('',(21.8,29.7504935167013,22.8288881795131));
#78023=CARTESIAN_POINT('Ctrl Pts',(21.8,31.6274058196267,20.1483796152605));
#78024=CARTESIAN_POINT('Ctrl Pts',(21.8713861730394,30.688949668164,21.4886338973868));
#78025=CARTESIAN_POINT('Ctrl Pts',(21.8,29.7504935167013,22.8288881795131));
#78026=CARTESIAN_POINT('',(21.5,30.0060755079215,22.9885935327265));
#78027=CARTESIAN_POINT('Ctrl Pts',(21.8,29.7504935167013,22.8288881795131));
#78028=CARTESIAN_POINT('Ctrl Pts',(21.6506031101081,29.8777753824163,22.9084227164522));
#78029=CARTESIAN_POINT('Ctrl Pts',(21.5,30.0060755079215,22.9885935327265));
#78030=CARTESIAN_POINT('',(21.5,27.8498454727622,25.5582884235871));
#78031=CARTESIAN_POINT('Origin',(21.5,0.,0.));
#78032=CARTESIAN_POINT('',(21.8,27.6481850557002,25.3343218406523));
#78033=CARTESIAN_POINT('Ctrl Pts',(21.5,27.8498454727622,25.5582884235871));
#78034=CARTESIAN_POINT('Ctrl Pts',(21.6506031063136,27.7486135508925,25.4458589842583));
#78035=CARTESIAN_POINT('Ctrl Pts',(21.8,27.6481850557002,25.3343218406523));
#78036=CARTESIAN_POINT('',(21.8,25.3343218406523,27.6481850557002));
#78037=CARTESIAN_POINT('Ctrl Pts',(21.8,27.6481850557002,25.3343218406523));
#78038=CARTESIAN_POINT('Ctrl Pts',(21.8713861730393,26.4912534481763,26.4912534481763));
#78039=CARTESIAN_POINT('Ctrl Pts',(21.8,25.3343218406523,27.6481850557002));
#78040=CARTESIAN_POINT('',(21.5,25.5582884235871,27.8498454727622));
#78041=CARTESIAN_POINT('Ctrl Pts',(21.8,25.3343218406523,27.6481850557002));
#78042=CARTESIAN_POINT('Ctrl Pts',(21.6506031088795,25.4458589823425,27.7486135491675));
#78043=CARTESIAN_POINT('Ctrl Pts',(21.5,25.5582884235871,27.8498454727622));
#78044=CARTESIAN_POINT('',(21.5,22.9885935327265,30.0060755079215));
#78045=CARTESIAN_POINT('Origin',(21.5,0.,0.));
#78046=CARTESIAN_POINT('',(21.8,22.8288881795131,29.7504935167013));
#78047=CARTESIAN_POINT('Ctrl Pts',(21.5,22.9885935327265,30.0060755079215));
#78048=CARTESIAN_POINT('Ctrl Pts',(21.6506031143833,22.9084227141762,29.8777753787739));
#78049=CARTESIAN_POINT('Ctrl Pts',(21.8,22.8288881795131,29.7504935167013));
#78050=CARTESIAN_POINT('',(21.8,20.1483796152605,31.6274058196267));
#78051=CARTESIAN_POINT('Ctrl Pts',(21.8,22.8288881795131,29.7504935167013));
#78052=CARTESIAN_POINT('Ctrl Pts',(21.8713861730394,21.4886338973868,30.688949668164));
#78053=CARTESIAN_POINT('Ctrl Pts',(21.8,20.1483796152605,31.6274058196267));
#78054=CARTESIAN_POINT('',(21.5,20.3339256786199,31.8648939508099));
#78055=CARTESIAN_POINT('Ctrl Pts',(21.8,20.1483796152605,31.6274058196267));
#78056=CARTESIAN_POINT('Ctrl Pts',(21.6506031061559,20.2407830339541,31.7456768021696));
#78057=CARTESIAN_POINT('Ctrl Pts',(21.5,20.3339256786199,31.8648939508099));
#78058=CARTESIAN_POINT('',(21.5,17.4288448109885,33.5421431717545));
#78059=CARTESIAN_POINT('Origin',(21.5,0.,0.));
#78060=CARTESIAN_POINT('',(21.8,17.3159470879662,33.2627115017215));
#78061=CARTESIAN_POINT('Ctrl Pts',(21.5,17.4288448109885,33.5421431717545));
#78062=CARTESIAN_POINT('Ctrl Pts',(21.6506031121263,17.3721710517851,33.4018706954166));
#78063=CARTESIAN_POINT('Ctrl Pts',(21.8,17.3159470879662,33.2627115017215));
#78064=CARTESIAN_POINT('',(21.8,14.3502390708311,34.6456438619633));
#78065=CARTESIAN_POINT('Ctrl Pts',(21.8,17.3159470879662,33.2627115017215));
#78066=CARTESIAN_POINT('Ctrl Pts',(21.8713861730394,15.8330930793986,33.9541776818424));
#78067=CARTESIAN_POINT('Ctrl Pts',(21.8,14.3502390708311,34.6456438619633));
#78068=CARTESIAN_POINT('',(21.5,14.4917268913708,34.9117437505765));
#78069=CARTESIAN_POINT('Ctrl Pts',(21.8,14.3502390708311,34.6456438619633));
#78070=CARTESIAN_POINT('Ctrl Pts',(21.6506031093095,14.4207011318884,34.7781637249967));
#78071=CARTESIAN_POINT('Ctrl Pts',(21.5,14.4917268913708,34.9117437505765));
#78072=CARTESIAN_POINT('',(21.5,11.3395294590896,36.0590497884572));
#78073=CARTESIAN_POINT('Origin',(21.5,0.,0.));
#78074=CARTESIAN_POINT('',(21.8,11.2768697064435,35.764258829506));
#78075=CARTESIAN_POINT('Ctrl Pts',(21.5,11.3395294590896,36.0590497884573));
#78076=CARTESIAN_POINT('Ctrl Pts',(21.6506031035411,11.30807476332,35.911067079655));
#78077=CARTESIAN_POINT('Ctrl Pts',(21.8,11.2768697064435,35.764258829506));
#78078=CARTESIAN_POINT('',(21.8,8.11607377380575,36.6111915470959));
#78079=CARTESIAN_POINT('Ctrl Pts',(21.8,11.2768697064435,35.764258829506));
#78080=CARTESIAN_POINT('Ctrl Pts',(21.8713861730393,9.69647174012463,36.1877251883009));
#78081=CARTESIAN_POINT('Ctrl Pts',(21.8,8.11607377380575,36.6111915470959));
#78082=CARTESIAN_POINT('',(21.5,8.20920431569501,36.8978178826767));
#78083=CARTESIAN_POINT('Ctrl Pts',(21.8,8.11607377380575,36.6111915470959));
#78084=CARTESIAN_POINT('Ctrl Pts',(21.6506031086535,8.1624535253115,36.7539337447634));
#78085=CARTESIAN_POINT('Ctrl Pts',(21.5,8.20920431569501,36.8978178826767));
#78086=CARTESIAN_POINT('',(21.5,4.90566824265507,37.4803204240973));
#78087=CARTESIAN_POINT('Origin',(21.5,0.,0.));
#78088=CARTESIAN_POINT('',(21.8,4.89515034526195,37.1791272503441));
#78089=CARTESIAN_POINT('Ctrl Pts',(21.5,4.90566824265507,37.4803204240973));
#78090=CARTESIAN_POINT('Ctrl Pts',(21.6506031094157,4.90038834189625,37.3291238486592));
#78091=CARTESIAN_POINT('Ctrl Pts',(21.8,4.89515034526195,37.1791272503441));
#78092=CARTESIAN_POINT('',(21.8,1.63530568209483,37.4643267032268));
#78093=CARTESIAN_POINT('Ctrl Pts',(21.8,4.89515034526195,37.1791272503441));
#78094=CARTESIAN_POINT('Ctrl Pts',(21.8713861730393,3.26522801367839,37.3217269767854));
#78095=CARTESIAN_POINT('Ctrl Pts',(21.8,1.63530568209483,37.4643267032268));
#78096=CARTESIAN_POINT('',(21.5,1.67724922094465,37.7627704896084));
#78097=CARTESIAN_POINT('Ctrl Pts',(21.8,1.63530568209483,37.4643267032268));
#78098=CARTESIAN_POINT('Ctrl Pts',(21.6506031053325,1.65619389892368,37.6129540888054));
#78099=CARTESIAN_POINT('Ctrl Pts',(21.5,1.67724922094465,37.7627704896084));
#78100=CARTESIAN_POINT('',(21.5,-1.67724922094464,37.7627704896084));
#78101=CARTESIAN_POINT('Origin',(21.5,0.,0.));
#78102=CARTESIAN_POINT('',(21.8,-1.63530568209482,37.4643267032267));
#78103=CARTESIAN_POINT('Ctrl Pts',(21.5,-1.67724922094464,37.7627704896084));
#78104=CARTESIAN_POINT('Ctrl Pts',(21.6506031054257,-1.65619389891064,37.6129540887127));
#78105=CARTESIAN_POINT('Ctrl Pts',(21.8,-1.63530568209482,37.4643267032267));
#78106=CARTESIAN_POINT('',(21.8,-4.89515034526194,37.1791272503441));
#78107=CARTESIAN_POINT('Ctrl Pts',(21.8,-1.63530568209482,37.4643267032267));
#78108=CARTESIAN_POINT('Ctrl Pts',(21.8713861730394,-3.26522801367839,37.3217269767854));
#78109=CARTESIAN_POINT('Ctrl Pts',(21.8,-4.89515034526194,37.1791272503441));
#78110=CARTESIAN_POINT('',(21.5,-4.90566824265506,37.4803204240973));
#78111=CARTESIAN_POINT('Ctrl Pts',(21.8,-4.89515034526194,37.1791272503441));
#78112=CARTESIAN_POINT('Ctrl Pts',(21.6506031056954,-4.90038834202669,37.3291238523946));
#78113=CARTESIAN_POINT('Ctrl Pts',(21.5,-4.90566824265506,37.4803204240973));
#78114=CARTESIAN_POINT('',(21.5,-8.20920431569501,36.8978178826767));
#78115=CARTESIAN_POINT('Origin',(21.5,0.,0.));
#78116=CARTESIAN_POINT('',(21.8,-8.11607377380574,36.6111915470959));
#78117=CARTESIAN_POINT('Ctrl Pts',(21.5,-8.20920431569501,36.8978178826767));
#78118=CARTESIAN_POINT('Ctrl Pts',(21.6506031085607,-8.16245352534031,36.7539337448521));
#78119=CARTESIAN_POINT('Ctrl Pts',(21.8,-8.11607377380574,36.6111915470959));
#78120=CARTESIAN_POINT('',(21.8,-11.2768697064435,35.764258829506));
#78121=CARTESIAN_POINT('Ctrl Pts',(21.8,-8.11607377380574,36.6111915470959));
#78122=CARTESIAN_POINT('Ctrl Pts',(21.8713861730394,-9.69647174012463,36.1877251883009));
#78123=CARTESIAN_POINT('Ctrl Pts',(21.8,-11.2768697064435,35.764258829506));
#78124=CARTESIAN_POINT('',(21.5,-11.3395294590896,36.0590497884573));
#78125=CARTESIAN_POINT('Ctrl Pts',(21.8,-11.2768697064435,35.764258829506));
#78126=CARTESIAN_POINT('Ctrl Pts',(21.6506031074235,-11.308074762509,35.9110670758397));
#78127=CARTESIAN_POINT('Ctrl Pts',(21.5,-11.3395294590896,36.0590497884573));
#78128=CARTESIAN_POINT('',(21.5,-14.4917268913708,34.9117437505765));
#78129=CARTESIAN_POINT('Origin',(21.5,0.,0.));
#78130=CARTESIAN_POINT('',(21.8,-14.3502390708311,34.6456438619633));
#78131=CARTESIAN_POINT('Ctrl Pts',(21.5,-14.4917268913708,34.9117437505765));
#78132=CARTESIAN_POINT('Ctrl Pts',(21.6506031093456,-14.4207011318714,34.7781637249647));
#78133=CARTESIAN_POINT('Ctrl Pts',(21.8,-14.3502390708311,34.6456438619633));
#78134=CARTESIAN_POINT('',(21.8,-17.3159470879662,33.2627115017215));
#78135=CARTESIAN_POINT('Ctrl Pts',(21.8,-14.3502390708311,34.6456438619633));
#78136=CARTESIAN_POINT('Ctrl Pts',(21.8713861730394,-15.8330930793986,33.9541776818424));
#78137=CARTESIAN_POINT('Ctrl Pts',(21.8,-17.3159470879662,33.2627115017215));
#78138=CARTESIAN_POINT('',(21.5,-17.4288448109885,33.5421431717545));
#78139=CARTESIAN_POINT('Ctrl Pts',(21.8,-17.3159470879662,33.2627115017215));
#78140=CARTESIAN_POINT('Ctrl Pts',(21.6506031114957,-17.3721710520224,33.401870696004));
#78141=CARTESIAN_POINT('Ctrl Pts',(21.5,-17.4288448109885,33.5421431717545));
#78142=CARTESIAN_POINT('Origin',(21.5,0.,0.));
#78143=CARTESIAN_POINT('Origin',(21.75,0.,0.));
#78144=CARTESIAN_POINT('',(21.8,-11.2768697064435,-35.764258829506));
#78145=CARTESIAN_POINT('Ctrl Pts',(21.5,-11.3395294590896,-36.0590497884572));
#78146=CARTESIAN_POINT('Ctrl Pts',(21.6506031111505,-11.3080747617305,-35.9110670721771));
#78147=CARTESIAN_POINT('Ctrl Pts',(21.8,-11.2768697064435,-35.764258829506));
#78148=CARTESIAN_POINT('',(21.8,-8.11607377380577,-36.6111915470959));
#78149=CARTESIAN_POINT('Ctrl Pts',(21.8,-11.2768697064435,-35.764258829506));
#78150=CARTESIAN_POINT('Ctrl Pts',(21.8713861730393,-9.69647174012465,-36.1877251883009));
#78151=CARTESIAN_POINT('Ctrl Pts',(21.8,-8.11607377380577,-36.6111915470959));
#78152=CARTESIAN_POINT('',(21.5,-8.20920431569503,-36.8978178826767));
#78153=CARTESIAN_POINT('Ctrl Pts',(21.8,-8.11607377380577,-36.6111915470959));
#78154=CARTESIAN_POINT('Ctrl Pts',(21.6506031047876,-8.16245352651173,-36.7539337484572));
#78155=CARTESIAN_POINT('Ctrl Pts',(21.5,-8.20920431569504,-36.8978178826767));
#78156=CARTESIAN_POINT('',(21.5,-4.90566824265507,-37.4803204240973));
#78157=CARTESIAN_POINT('Origin',(21.5,0.,0.));
#78158=CARTESIAN_POINT('',(21.8,-4.89515034526194,-37.1791272503441));
#78159=CARTESIAN_POINT('Ctrl Pts',(21.5,-4.90566824265507,-37.4803204240973));
#78160=CARTESIAN_POINT('Ctrl Pts',(21.6506031094336,-4.90038834189562,-37.3291238486412));
#78161=CARTESIAN_POINT('Ctrl Pts',(21.8,-4.89515034526194,-37.1791272503441));
#78162=CARTESIAN_POINT('',(21.8,-1.63530568209482,-37.4643267032267));
#78163=CARTESIAN_POINT('Ctrl Pts',(21.8,-4.89515034526194,-37.1791272503441));
#78164=CARTESIAN_POINT('Ctrl Pts',(21.8713861730394,-3.26522801367838,-37.3217269767854));
#78165=CARTESIAN_POINT('Ctrl Pts',(21.8,-1.63530568209482,-37.4643267032267));
#78166=CARTESIAN_POINT('',(21.5,-1.67724922094465,-37.7627704896084));
#78167=CARTESIAN_POINT('Ctrl Pts',(21.8,-1.63530568209482,-37.4643267032267));
#78168=CARTESIAN_POINT('Ctrl Pts',(21.6506031054194,-1.65619389891153,-37.612954088719));
#78169=CARTESIAN_POINT('Ctrl Pts',(21.5,-1.67724922094465,-37.7627704896084));
#78170=CARTESIAN_POINT('',(21.5,1.67724922094464,-37.7627704896084));
#78171=CARTESIAN_POINT('Origin',(21.5,0.,0.));
#78172=CARTESIAN_POINT('',(21.8,1.63530568209482,-37.4643267032267));
#78173=CARTESIAN_POINT('Ctrl Pts',(21.5,1.67724922094464,-37.7627704896084));
#78174=CARTESIAN_POINT('Ctrl Pts',(21.6506031054903,1.6561938989016,-37.6129540886484));
#78175=CARTESIAN_POINT('Ctrl Pts',(21.8,1.63530568209482,-37.4643267032267));
#78176=CARTESIAN_POINT('',(21.8,4.89515034526193,-37.1791272503441));
#78177=CARTESIAN_POINT('Ctrl Pts',(21.8,1.63530568209482,-37.4643267032267));
#78178=CARTESIAN_POINT('Ctrl Pts',(21.8713861730394,3.26522801367838,-37.3217269767854));
#78179=CARTESIAN_POINT('Ctrl Pts',(21.8,4.89515034526193,-37.1791272503441));
#78180=CARTESIAN_POINT('',(21.5,4.90566824265506,-37.4803204240973));
#78181=CARTESIAN_POINT('Ctrl Pts',(21.8,4.89515034526193,-37.1791272503441));
#78182=CARTESIAN_POINT('Ctrl Pts',(21.6506031093552,4.90038834189836,-37.3291238487199));
#78183=CARTESIAN_POINT('Ctrl Pts',(21.5,4.90566824265506,-37.4803204240973));
#78184=CARTESIAN_POINT('',(21.5,8.209204315695,-36.8978178826767));
#78185=CARTESIAN_POINT('Origin',(21.5,0.,0.));
#78186=CARTESIAN_POINT('',(21.8,8.11607377380573,-36.6111915470959));
#78187=CARTESIAN_POINT('Ctrl Pts',(21.5,8.209204315695,-36.8978178826767));
#78188=CARTESIAN_POINT('Ctrl Pts',(21.6506031085797,8.1624535253344,-36.7539337448339));
#78189=CARTESIAN_POINT('Ctrl Pts',(21.8,8.11607377380573,-36.6111915470958));
#78190=CARTESIAN_POINT('',(21.8,11.2768697064435,-35.764258829506));
#78191=CARTESIAN_POINT('Ctrl Pts',(21.8,8.11607377380573,-36.6111915470959));
#78192=CARTESIAN_POINT('Ctrl Pts',(21.8713861730394,9.69647174012462,-36.1877251883009));
#78193=CARTESIAN_POINT('Ctrl Pts',(21.8,11.2768697064435,-35.764258829506));
#78194=CARTESIAN_POINT('',(21.5,11.3395294590896,-36.0590497884573));
#78195=CARTESIAN_POINT('Ctrl Pts',(21.8,11.2768697064435,-35.764258829506));
#78196=CARTESIAN_POINT('Ctrl Pts',(21.6506031037827,11.3080747632695,-35.9110670794176));
#78197=CARTESIAN_POINT('Ctrl Pts',(21.5,11.3395294590896,-36.0590497884573));
#78198=CARTESIAN_POINT('',(21.5,14.4917268913708,-34.9117437505765));
#78199=CARTESIAN_POINT('Origin',(21.5,0.,0.));
#78200=CARTESIAN_POINT('',(21.8,14.350239070831,-34.6456438619633));
#78201=CARTESIAN_POINT('Ctrl Pts',(21.5,14.4917268913708,-34.9117437505766));
#78202=CARTESIAN_POINT('Ctrl Pts',(21.6506031096943,14.4207011317069,-34.7781637246554));
#78203=CARTESIAN_POINT('Ctrl Pts',(21.8,14.350239070831,-34.6456438619633));
#78204=CARTESIAN_POINT('',(21.8,17.3159470879662,-33.2627115017215));
#78205=CARTESIAN_POINT('Ctrl Pts',(21.8,14.350239070831,-34.6456438619633));
#78206=CARTESIAN_POINT('Ctrl Pts',(21.8713861730393,15.8330930793986,-33.9541776818424));
#78207=CARTESIAN_POINT('Ctrl Pts',(21.8,17.3159470879662,-33.2627115017215));
#78208=CARTESIAN_POINT('',(21.5,17.4288448109885,-33.5421431717545));
#78209=CARTESIAN_POINT('Ctrl Pts',(21.8,17.3159470879662,-33.2627115017215));
#78210=CARTESIAN_POINT('Ctrl Pts',(21.6506031077603,17.3721710534283,-33.4018706994836));
#78211=CARTESIAN_POINT('Ctrl Pts',(21.5,17.4288448109885,-33.5421431717546));
#78212=CARTESIAN_POINT('',(21.5,20.3339256786199,-31.8648939508099));
#78213=CARTESIAN_POINT('Origin',(21.5,0.,0.));
#78214=CARTESIAN_POINT('',(21.8,20.1483796152605,-31.6274058196267));
#78215=CARTESIAN_POINT('Ctrl Pts',(21.5,20.3339256786199,-31.8648939508099));
#78216=CARTESIAN_POINT('Ctrl Pts',(21.6506031087829,20.2407830323292,-31.7456768000897));
#78217=CARTESIAN_POINT('Ctrl Pts',(21.8,20.1483796152605,-31.6274058196267));
#78218=CARTESIAN_POINT('',(21.8,22.8288881795131,-29.7504935167013));
#78219=CARTESIAN_POINT('Ctrl Pts',(21.8,20.1483796152605,-31.6274058196267));
#78220=CARTESIAN_POINT('Ctrl Pts',(21.8713861730394,21.4886338973868,-30.688949668164));
#78221=CARTESIAN_POINT('Ctrl Pts',(21.8,22.8288881795131,-29.7504935167013));
#78222=CARTESIAN_POINT('',(21.5,22.9885935327265,-30.0060755079215));
#78223=CARTESIAN_POINT('Ctrl Pts',(21.8,22.8288881795131,-29.7504935167013));
#78224=CARTESIAN_POINT('Ctrl Pts',(21.6506031065164,22.9084227183644,-29.8777753854765));
#78225=CARTESIAN_POINT('Ctrl Pts',(21.5,22.9885935327265,-30.0060755079215));
#78226=CARTESIAN_POINT('',(21.5,25.5582884235871,-27.8498454727622));
#78227=CARTESIAN_POINT('Origin',(21.5,0.,0.));
#78228=CARTESIAN_POINT('',(21.8,25.3343218406523,-27.6481850557002));
#78229=CARTESIAN_POINT('Ctrl Pts',(21.5,25.5582884235871,-27.8498454727622));
#78230=CARTESIAN_POINT('Ctrl Pts',(21.6506031049548,25.4458589852728,-27.748613551806));
#78231=CARTESIAN_POINT('Ctrl Pts',(21.8,25.3343218406523,-27.6481850557002));
#78232=CARTESIAN_POINT('',(21.8,27.6481850557002,-25.3343218406523));
#78233=CARTESIAN_POINT('Ctrl Pts',(21.8,25.3343218406523,-27.6481850557002));
#78234=CARTESIAN_POINT('Ctrl Pts',(21.8713861730394,26.4912534481763,-26.4912534481763));
#78235=CARTESIAN_POINT('Ctrl Pts',(21.8,27.6481850557002,-25.3343218406523));
#78236=CARTESIAN_POINT('',(21.5,27.8498454727622,-25.5582884235871));
#78237=CARTESIAN_POINT('Ctrl Pts',(21.8,27.6481850557002,-25.3343218406523));
#78238=CARTESIAN_POINT('Ctrl Pts',(21.650603106132,27.7486135510146,-25.4458589843939));
#78239=CARTESIAN_POINT('Ctrl Pts',(21.5,27.8498454727622,-25.5582884235871));
#78240=CARTESIAN_POINT('',(21.5,30.0060755079215,-22.9885935327265));
#78241=CARTESIAN_POINT('Origin',(21.5,0.,0.));
#78242=CARTESIAN_POINT('',(21.8,29.7504935167013,-22.8288881795131));
#78243=CARTESIAN_POINT('Ctrl Pts',(21.5,30.0060755079215,-22.9885935327265));
#78244=CARTESIAN_POINT('Ctrl Pts',(21.6506031103219,29.8777753822342,-22.9084227163384));
#78245=CARTESIAN_POINT('Ctrl Pts',(21.8,29.7504935167013,-22.8288881795131));
#78246=CARTESIAN_POINT('',(21.8,31.6274058196267,-20.1483796152605));
#78247=CARTESIAN_POINT('Ctrl Pts',(21.8,29.7504935167013,-22.8288881795131));
#78248=CARTESIAN_POINT('Ctrl Pts',(21.8713861730394,30.688949668164,-21.4886338973868));
#78249=CARTESIAN_POINT('Ctrl Pts',(21.8,31.6274058196267,-20.1483796152605));
#78250=CARTESIAN_POINT('',(21.5,31.8648939508099,-20.3339256786199));
#78251=CARTESIAN_POINT('Ctrl Pts',(21.8,31.6274058196267,-20.1483796152605));
#78252=CARTESIAN_POINT('Ctrl Pts',(21.6506031038392,31.7456768040036,-20.2407830353871));
#78253=CARTESIAN_POINT('Ctrl Pts',(21.5,31.8648939508099,-20.3339256786199));
#78254=CARTESIAN_POINT('',(21.5,33.5421431717545,-17.4288448109885));
#78255=CARTESIAN_POINT('Origin',(21.5,0.,0.));
#78256=CARTESIAN_POINT('',(21.8,33.2627115017215,-17.3159470879662));
#78257=CARTESIAN_POINT('Ctrl Pts',(21.5,33.5421431717545,-17.4288448109885));
#78258=CARTESIAN_POINT('Ctrl Pts',(21.6506031041173,33.4018707028771,-17.3721710547994));
#78259=CARTESIAN_POINT('Ctrl Pts',(21.8,33.2627115017215,-17.3159470879662));
#78260=CARTESIAN_POINT('',(21.8,34.6456438619633,-14.3502390708311));
#78261=CARTESIAN_POINT('Ctrl Pts',(21.8,33.2627115017215,-17.3159470879662));
#78262=CARTESIAN_POINT('Ctrl Pts',(21.8713861730393,33.9541776818424,-15.8330930793987));
#78263=CARTESIAN_POINT('Ctrl Pts',(21.8,34.6456438619633,-14.3502390708311));
#78264=CARTESIAN_POINT('',(21.5,34.9117437505765,-14.4917268913708));
#78265=CARTESIAN_POINT('Ctrl Pts',(21.8,34.6456438619633,-14.3502390708311));
#78266=CARTESIAN_POINT('Ctrl Pts',(21.6506031056005,34.7781637282868,-14.4207011336378));
#78267=CARTESIAN_POINT('Ctrl Pts',(21.5,34.9117437505765,-14.4917268913708));
#78268=CARTESIAN_POINT('',(21.5,36.0590497884572,-11.3395294590896));
#78269=CARTESIAN_POINT('Origin',(21.5,0.,0.));
#78270=CARTESIAN_POINT('',(21.8,35.764258829506,-11.2768697064435));
#78271=CARTESIAN_POINT('Ctrl Pts',(21.5,36.0590497884572,-11.3395294590896));
#78272=CARTESIAN_POINT('Ctrl Pts',(21.6506031073768,35.9110670758856,-11.3080747625188));
#78273=CARTESIAN_POINT('Ctrl Pts',(21.8,35.764258829506,-11.2768697064435));
#78274=CARTESIAN_POINT('',(21.8,36.6111915470958,-8.11607377380577));
#78275=CARTESIAN_POINT('Ctrl Pts',(21.8,35.764258829506,-11.2768697064435));
#78276=CARTESIAN_POINT('Ctrl Pts',(21.8713861730393,36.1877251883009,-9.69647174012465));
#78277=CARTESIAN_POINT('Ctrl Pts',(21.8,36.6111915470958,-8.11607377380577));
#78278=CARTESIAN_POINT('',(21.5,36.8978178826767,-8.20920431569504));
#78279=CARTESIAN_POINT('Ctrl Pts',(21.8,36.6111915470958,-8.11607377380577));
#78280=CARTESIAN_POINT('Ctrl Pts',(21.6506031087027,36.7539337447164,-8.16245352529625));
#78281=CARTESIAN_POINT('Ctrl Pts',(21.5,36.8978178826767,-8.20920431569504));
#78282=CARTESIAN_POINT('',(21.5,37.4803204240973,-4.90566824265507));
#78283=CARTESIAN_POINT('Origin',(21.5,0.,0.));
#78284=CARTESIAN_POINT('',(21.8,37.1791272503441,-4.89515034526195));
#78285=CARTESIAN_POINT('Ctrl Pts',(21.5,37.4803204240973,-4.90566824265507));
#78286=CARTESIAN_POINT('Ctrl Pts',(21.6506031020327,37.3291238560722,-4.90038834215512));
#78287=CARTESIAN_POINT('Ctrl Pts',(21.8,37.1791272503441,-4.89515034526195));
#78288=CARTESIAN_POINT('',(21.8,37.4643267032267,-1.63530568209483));
#78289=CARTESIAN_POINT('Ctrl Pts',(21.8,37.1791272503441,-4.89515034526195));
#78290=CARTESIAN_POINT('Ctrl Pts',(21.8713861730394,37.3217269767854,-3.26522801367838));
#78291=CARTESIAN_POINT('Ctrl Pts',(21.8,37.4643267032267,-1.63530568209483));
#78292=CARTESIAN_POINT('',(21.5,37.7627704896084,-1.67724922094465));
#78293=CARTESIAN_POINT('Ctrl Pts',(21.8,37.4643267032267,-1.63530568209483));
#78294=CARTESIAN_POINT('Ctrl Pts',(21.6506031055069,37.6129540886319,-1.6561938988993));
#78295=CARTESIAN_POINT('Ctrl Pts',(21.5,37.7627704896084,-1.67724922094465));
#78296=CARTESIAN_POINT('',(21.5,37.7878017125899,-0.960230040142118));
#78297=CARTESIAN_POINT('Origin',(21.5,0.,0.));
#78298=CARTESIAN_POINT('',(22.,37.2864828558561,-1.0040897569181));
#78299=CARTESIAN_POINT('Ctrl Pts',(21.5,37.7878017125899,-0.960230040142117));
#78300=CARTESIAN_POINT('Ctrl Pts',(21.7516860406602,37.5354734529172,-0.982305902350696));
#78301=CARTESIAN_POINT('Ctrl Pts',(22.,37.2864828558561,-1.0040897569181));
#78302=CARTESIAN_POINT('Origin',(22.,0.,0.));
#78303=CARTESIAN_POINT('Origin',(11.,0.,0.));
#78304=CARTESIAN_POINT('',(11.,-25.5582884235871,27.8498454727622));
#78305=CARTESIAN_POINT('Origin',(0.249999999999999,0.,0.));
#78306=CARTESIAN_POINT('',(0.499999999999998,-17.4288448109885,33.5421431717545));
#78307=CARTESIAN_POINT('Origin',(0.499999999999998,0.,0.));
#78308=CARTESIAN_POINT('',(0.200000000000004,-17.3159470879662,33.2627115017215));
#78309=CARTESIAN_POINT('Ctrl Pts',(0.500000000000001,-17.4288448109885,
33.5421431717545));
#78310=CARTESIAN_POINT('Ctrl Pts',(0.349396891634736,-17.3721710532006,
33.40187069892));
#78311=CARTESIAN_POINT('Ctrl Pts',(0.200000000000004,-17.3159470879662,
33.2627115017215));
#78312=CARTESIAN_POINT('',(0.200000000000008,-14.3502390708311,34.6456438619633));
#78313=CARTESIAN_POINT('Ctrl Pts',(0.200000000000004,-17.3159470879662,
33.2627115017215));
#78314=CARTESIAN_POINT('Ctrl Pts',(0.128613826960649,-15.8330930793986,
33.9541776818424));
#78315=CARTESIAN_POINT('Ctrl Pts',(0.200000000000008,-14.3502390708311,
34.6456438619633));
#78316=CARTESIAN_POINT('',(0.499999999999998,-14.4917268913708,34.9117437505765));
#78317=CARTESIAN_POINT('Ctrl Pts',(0.200000000000008,-14.3502390708311,
34.6456438619633));
#78318=CARTESIAN_POINT('Ctrl Pts',(0.349396894490965,-14.420701133681,34.778163728368));
#78319=CARTESIAN_POINT('Ctrl Pts',(0.500000000000001,-14.4917268913708,
34.9117437505765));
#78320=CARTESIAN_POINT('',(0.499999999999998,-11.3395294590896,36.0590497884573));
#78321=CARTESIAN_POINT('Origin',(0.499999999999998,0.,0.));
#78322=CARTESIAN_POINT('',(0.200000000000006,-11.2768697064435,35.764258829506));
#78323=CARTESIAN_POINT('Ctrl Pts',(0.500000000000001,-11.3395294590896,
36.0590497884573));
#78324=CARTESIAN_POINT('Ctrl Pts',(0.349396892532884,-11.3080747624999,
35.9110670757969));
#78325=CARTESIAN_POINT('Ctrl Pts',(0.200000000000006,-11.2768697064435,
35.764258829506));
#78326=CARTESIAN_POINT('',(0.200000000000009,-8.11607377380574,36.6111915470959));
#78327=CARTESIAN_POINT('Ctrl Pts',(0.200000000000006,-11.2768697064435,
35.764258829506));
#78328=CARTESIAN_POINT('Ctrl Pts',(0.128613826960651,-9.69647174012462,
36.1877251883009));
#78329=CARTESIAN_POINT('Ctrl Pts',(0.200000000000009,-8.11607377380574,
36.6111915470959));
#78330=CARTESIAN_POINT('',(0.499999999999998,-8.20920431569501,36.8978178826767));
#78331=CARTESIAN_POINT('Ctrl Pts',(0.200000000000009,-8.11607377380574,
36.6111915470959));
#78332=CARTESIAN_POINT('Ctrl Pts',(0.349396891056085,-8.16245352522133,
36.7539337444859));
#78333=CARTESIAN_POINT('Ctrl Pts',(0.500000000000001,-8.20920431569501,
36.8978178826767));
#78334=CARTESIAN_POINT('',(0.499999999999998,-4.90566824265506,37.4803204240973));
#78335=CARTESIAN_POINT('Origin',(0.499999999999998,0.,0.));
#78336=CARTESIAN_POINT('',(0.200000000000002,-4.89515034526194,37.1791272503441));
#78337=CARTESIAN_POINT('Ctrl Pts',(0.500000000000001,-4.90566824265506,
37.4803204240973));
#78338=CARTESIAN_POINT('Ctrl Pts',(0.349396894143512,-4.90038834202104,
37.3291238522329));
#78339=CARTESIAN_POINT('Ctrl Pts',(0.200000000000002,-4.89515034526194,
37.1791272503441));
#78340=CARTESIAN_POINT('',(0.200000000000005,-1.63530568209482,37.4643267032267));
#78341=CARTESIAN_POINT('Ctrl Pts',(0.200000000000002,-4.89515034526194,
37.1791272503441));
#78342=CARTESIAN_POINT('Ctrl Pts',(0.128613826960647,-3.26522801367838,
37.3217269767854));
#78343=CARTESIAN_POINT('Ctrl Pts',(0.200000000000005,-1.63530568209482,
37.4643267032267));
#78344=CARTESIAN_POINT('',(0.499999999999998,-1.67724922094464,37.7627704896084));
#78345=CARTESIAN_POINT('Ctrl Pts',(0.200000000000005,-1.63530568209482,
37.4643267032267));
#78346=CARTESIAN_POINT('Ctrl Pts',(0.349396890838704,-1.65619389838832,
37.6129540849961));
#78347=CARTESIAN_POINT('Ctrl Pts',(0.500000000000001,-1.67724922094464,
37.7627704896084));
#78348=CARTESIAN_POINT('',(0.499999999999998,1.67724922094465,37.7627704896084));
#78349=CARTESIAN_POINT('Origin',(0.499999999999998,0.,0.));
#78350=CARTESIAN_POINT('',(0.200000000000009,1.63530568209483,37.4643267032268));
#78351=CARTESIAN_POINT('Ctrl Pts',(0.500000000000001,1.67724922094465,37.7627704896084));
#78352=CARTESIAN_POINT('Ctrl Pts',(0.349396890774378,1.65619389837934,37.6129540849322));
#78353=CARTESIAN_POINT('Ctrl Pts',(0.200000000000009,1.63530568209483,37.4643267032268));
#78354=CARTESIAN_POINT('',(0.200000000000002,4.89515034526195,37.1791272503441));
#78355=CARTESIAN_POINT('Ctrl Pts',(0.200000000000009,1.63530568209483,37.4643267032268));
#78356=CARTESIAN_POINT('Ctrl Pts',(0.128613826960647,3.26522801367839,37.3217269767854));
#78357=CARTESIAN_POINT('Ctrl Pts',(0.200000000000002,4.89515034526195,37.1791272503441));
#78358=CARTESIAN_POINT('',(0.499999999999998,4.90566824265507,37.4803204240973));
#78359=CARTESIAN_POINT('Ctrl Pts',(0.200000000000002,4.89515034526195,37.1791272503441));
#78360=CARTESIAN_POINT('Ctrl Pts',(0.34939689050702,4.90038834189354,37.3291238485816));
#78361=CARTESIAN_POINT('Ctrl Pts',(0.500000000000001,4.90566824265507,37.4803204240973));
#78362=CARTESIAN_POINT('',(0.499999999999998,8.20920431569501,36.8978178826767));
#78363=CARTESIAN_POINT('Origin',(0.499999999999998,0.,0.));
#78364=CARTESIAN_POINT('',(0.200000000000009,8.11607377380574,36.6111915470959));
#78365=CARTESIAN_POINT('Ctrl Pts',(0.500000000000001,8.20920431569502,36.8978178826767));
#78366=CARTESIAN_POINT('Ctrl Pts',(0.349396891227305,8.16245352527449,36.7539337446495));
#78367=CARTESIAN_POINT('Ctrl Pts',(0.200000000000009,8.11607377380575,36.6111915470959));
#78368=CARTESIAN_POINT('',(0.20000000000001,11.2768697064435,35.764258829506));
#78369=CARTESIAN_POINT('Ctrl Pts',(0.200000000000009,8.11607377380574,36.6111915470959));
#78370=CARTESIAN_POINT('Ctrl Pts',(0.128613826960651,9.69647174012464,36.1877251883009));
#78371=CARTESIAN_POINT('Ctrl Pts',(0.20000000000001,11.2768697064435,35.764258829506));
#78372=CARTESIAN_POINT('',(0.499999999999998,11.3395294590896,36.0590497884572));
#78373=CARTESIAN_POINT('Ctrl Pts',(0.20000000000001,11.2768697064435,35.764258829506));
#78374=CARTESIAN_POINT('Ctrl Pts',(0.349396892476858,11.3080747624882,35.9110670757418));
#78375=CARTESIAN_POINT('Ctrl Pts',(0.500000000000001,11.3395294590896,36.0590497884572));
#78376=CARTESIAN_POINT('',(0.499999999999998,14.4917268913708,34.9117437505765));
#78377=CARTESIAN_POINT('Origin',(0.499999999999998,0.,0.));
#78378=CARTESIAN_POINT('',(0.200000000000003,14.3502390708311,34.6456438619633));
#78379=CARTESIAN_POINT('Ctrl Pts',(0.500000000000001,14.4917268913708,34.9117437505765));
#78380=CARTESIAN_POINT('Ctrl Pts',(0.349396894532555,14.4207011337006,34.7781637284049));
#78381=CARTESIAN_POINT('Ctrl Pts',(0.200000000000003,14.3502390708311,34.6456438619633));
#78382=CARTESIAN_POINT('',(0.200000000000003,17.3159470879662,33.2627115017215));
#78383=CARTESIAN_POINT('Ctrl Pts',(0.200000000000003,14.3502390708311,34.6456438619633));
#78384=CARTESIAN_POINT('Ctrl Pts',(0.128613826960644,15.8330930793986,33.9541776818424));
#78385=CARTESIAN_POINT('Ctrl Pts',(0.200000000000003,17.3159470879662,33.2627115017215));
#78386=CARTESIAN_POINT('',(0.499999999999998,17.4288448109885,33.5421431717545));
#78387=CARTESIAN_POINT('Ctrl Pts',(0.200000000000003,17.3159470879662,33.2627115017215));
#78388=CARTESIAN_POINT('Ctrl Pts',(0.349396895954869,17.3721710548265,33.4018707029443));
#78389=CARTESIAN_POINT('Ctrl Pts',(0.500000000000001,17.4288448109885,33.5421431717545));
#78390=CARTESIAN_POINT('',(0.499999999999998,20.3339256786199,31.8648939508099));
#78391=CARTESIAN_POINT('Origin',(0.499999999999998,0.,0.));
#78392=CARTESIAN_POINT('',(0.200000000000003,20.1483796152605,31.6274058196267));
#78393=CARTESIAN_POINT('Ctrl Pts',(0.500000000000001,20.3339256786199,31.8648939508099));
#78394=CARTESIAN_POINT('Ctrl Pts',(0.349396892392812,20.2407830330564,31.7456768010206));
#78395=CARTESIAN_POINT('Ctrl Pts',(0.200000000000003,20.1483796152605,31.6274058196267));
#78396=CARTESIAN_POINT('',(0.200000000000003,22.8288881795131,29.7504935167013));
#78397=CARTESIAN_POINT('Ctrl Pts',(0.200000000000003,20.1483796152605,31.6274058196267));
#78398=CARTESIAN_POINT('Ctrl Pts',(0.128613826960645,21.4886338973868,30.688949668164));
#78399=CARTESIAN_POINT('Ctrl Pts',(0.200000000000003,22.8288881795131,29.7504935167013));
#78400=CARTESIAN_POINT('',(0.499999999999998,22.9885935327265,30.0060755079215));
#78401=CARTESIAN_POINT('Ctrl Pts',(0.200000000000003,22.8288881795131,29.7504935167013));
#78402=CARTESIAN_POINT('Ctrl Pts',(0.349396892464199,22.9084227178217,29.877775384608));
#78403=CARTESIAN_POINT('Ctrl Pts',(0.500000000000001,22.9885935327265,30.0060755079215));
#78404=CARTESIAN_POINT('',(0.499999999999998,25.5582884235871,27.8498454727622));
#78405=CARTESIAN_POINT('Origin',(0.499999999999998,0.,0.));
#78406=CARTESIAN_POINT('',(0.200000000000009,25.3343218406523,27.6481850557002));
#78407=CARTESIAN_POINT('Ctrl Pts',(0.500000000000001,25.5582884235871,27.8498454727622));
#78408=CARTESIAN_POINT('Ctrl Pts',(0.3493968910558,25.4458589822943,27.7486135491241));
#78409=CARTESIAN_POINT('Ctrl Pts',(0.200000000000009,25.3343218406523,27.6481850557002));
#78410=CARTESIAN_POINT('',(0.200000000000006,27.6481850557002,25.3343218406523));
#78411=CARTESIAN_POINT('Ctrl Pts',(0.200000000000009,25.3343218406523,27.6481850557002));
#78412=CARTESIAN_POINT('Ctrl Pts',(0.128613826960648,26.4912534481763,26.4912534481763));
#78413=CARTESIAN_POINT('Ctrl Pts',(0.200000000000006,27.6481850557002,25.3343218406523));
#78414=CARTESIAN_POINT('',(0.499999999999998,27.8498454727622,25.5582884235871));
#78415=CARTESIAN_POINT('Ctrl Pts',(0.200000000000006,27.6481850557002,25.3343218406523));
#78416=CARTESIAN_POINT('Ctrl Pts',(0.349396897556482,27.7486135534942,25.4458589871478));
#78417=CARTESIAN_POINT('Ctrl Pts',(0.5,27.8498454727622,25.5582884235871));
#78418=CARTESIAN_POINT('',(0.499999999999998,30.0060755079215,22.9885935327265));
#78419=CARTESIAN_POINT('Origin',(0.499999999999998,0.,0.));
#78420=CARTESIAN_POINT('',(0.199999999999999,29.7504935167013,22.8288881795131));
#78421=CARTESIAN_POINT('Ctrl Pts',(0.5,30.0060755079215,22.9885935327265));
#78422=CARTESIAN_POINT('Ctrl Pts',(0.349396889752811,29.8777753822979,22.9084227163782));
#78423=CARTESIAN_POINT('Ctrl Pts',(0.199999999999999,29.7504935167013,22.8288881795131));
#78424=CARTESIAN_POINT('',(0.200000000000006,31.6274058196267,20.1483796152605));
#78425=CARTESIAN_POINT('Ctrl Pts',(0.199999999999999,29.7504935167013,22.8288881795131));
#78426=CARTESIAN_POINT('Ctrl Pts',(0.128613826960648,30.688949668164,21.4886338973868));
#78427=CARTESIAN_POINT('Ctrl Pts',(0.200000000000006,31.6274058196267,20.1483796152605));
#78428=CARTESIAN_POINT('',(0.499999999999998,31.8648939508099,20.3339256786199));
#78429=CARTESIAN_POINT('Ctrl Pts',(0.200000000000006,31.6274058196267,20.1483796152605));
#78430=CARTESIAN_POINT('Ctrl Pts',(0.349396891131353,31.7456768000219,20.2407830322762));
#78431=CARTESIAN_POINT('Ctrl Pts',(0.5,31.8648939508099,20.3339256786199));
#78432=CARTESIAN_POINT('',(0.499999999999998,33.5421431717545,17.4288448109885));
#78433=CARTESIAN_POINT('Origin',(0.499999999999998,0.,0.));
#78434=CARTESIAN_POINT('',(0.200000000000004,33.2627115017215,17.3159470879662));
#78435=CARTESIAN_POINT('Ctrl Pts',(0.5,33.5421431717545,17.4288448109885));
#78436=CARTESIAN_POINT('Ctrl Pts',(0.349396892387157,33.4018706996209,17.3721710534838));
#78437=CARTESIAN_POINT('Ctrl Pts',(0.200000000000004,33.2627115017215,17.3159470879662));
#78438=CARTESIAN_POINT('',(0.200000000000008,34.6456438619633,14.3502390708311));
#78439=CARTESIAN_POINT('Ctrl Pts',(0.200000000000004,33.2627115017215,17.3159470879662));
#78440=CARTESIAN_POINT('Ctrl Pts',(0.128613826960652,33.9541776818424,15.8330930793986));
#78441=CARTESIAN_POINT('Ctrl Pts',(0.200000000000008,34.6456438619633,14.3502390708311));
#78442=CARTESIAN_POINT('',(0.499999999999998,34.9117437505765,14.4917268913708));
#78443=CARTESIAN_POINT('Ctrl Pts',(0.200000000000008,34.6456438619633,14.3502390708311));
#78444=CARTESIAN_POINT('Ctrl Pts',(0.349396894409378,34.7781637282956,14.4207011336425));
#78445=CARTESIAN_POINT('Ctrl Pts',(0.5,34.9117437505765,14.4917268913708));
#78446=CARTESIAN_POINT('',(0.499999999999998,36.0590497884573,11.3395294590896));
#78447=CARTESIAN_POINT('Origin',(0.499999999999998,0.,0.));
#78448=CARTESIAN_POINT('',(0.20000000000001,35.764258829506,11.2768697064435));
#78449=CARTESIAN_POINT('Ctrl Pts',(0.5,36.0590497884572,11.3395294590896));
#78450=CARTESIAN_POINT('Ctrl Pts',(0.349396896292396,35.9110670794914,11.3080747632852));
#78451=CARTESIAN_POINT('Ctrl Pts',(0.20000000000001,35.764258829506,11.2768697064435));
#78452=CARTESIAN_POINT('',(0.200000000000009,36.6111915470959,8.11607377380574));
#78453=CARTESIAN_POINT('Ctrl Pts',(0.20000000000001,35.764258829506,11.2768697064435));
#78454=CARTESIAN_POINT('Ctrl Pts',(0.12861382696065,36.1877251883009,9.69647174012463));
#78455=CARTESIAN_POINT('Ctrl Pts',(0.200000000000009,36.6111915470958,8.11607377380574));
#78456=CARTESIAN_POINT('',(0.499999999999998,36.8978178826767,8.20920431569501));
#78457=CARTESIAN_POINT('Ctrl Pts',(0.200000000000009,36.6111915470959,8.11607377380574));
#78458=CARTESIAN_POINT('Ctrl Pts',(0.349396891698014,36.7539337450992,8.16245352542062));
#78459=CARTESIAN_POINT('Ctrl Pts',(0.5,36.8978178826767,8.20920431569501));
#78460=CARTESIAN_POINT('',(0.499999999999998,37.0469778992348,7.50742489363772));
#78461=CARTESIAN_POINT('Origin',(0.499999999999998,0.,0.));
#78462=CARTESIAN_POINT('Ctrl Pts',(0.500000000000004,37.0469778992348,7.50742489363772));
#78463=CARTESIAN_POINT('Ctrl Pts',(0.248313959403557,36.7946496396261,7.48534903143474));
#78464=CARTESIAN_POINT('Ctrl Pts',(-1.04083408558608E-16,36.545659042501,
7.46356517686174));
#78465=CARTESIAN_POINT('Origin',(0.,43.4621548093593,8.06868014778688));
#78466=CARTESIAN_POINT('',(22.,34.0979246472968,7.24941616595889));
#78467=CARTESIAN_POINT('',(22.,38.4167373519446,7.62726331750731));
#78468=CARTESIAN_POINT('',(0.,34.0979246472968,7.24941616595889));
#78469=CARTESIAN_POINT('',(11.,37.0469778992348,7.50742489363772));
#78470=CARTESIAN_POINT('Origin',(0.,34.8387484606519,-1.21823876782095));
#78471=CARTESIAN_POINT('',(11.,37.7878017125899,-0.960230040142118));
#78472=CARTESIAN_POINT('',(22.,34.8387484606519,-1.21823876782095));
#78473=CARTESIAN_POINT('',(0.,34.8387484606519,-1.21823876782095));
#78474=CARTESIAN_POINT('',(22.,34.4754460842685,-1.25002360718652));
#78475=CARTESIAN_POINT('Origin',(0.,34.0979246472968,7.24941616595889));
#78476=CARTESIAN_POINT('',(22.,34.4122647000319,3.65649292234502));
#78477=CARTESIAN_POINT('Origin',(11.,0.,0.));
#78478=CARTESIAN_POINT('',(11.,36.8978178826767,8.20920431569501));
#78479=CARTESIAN_POINT('Origin',(21.55,0.,0.));
#78480=CARTESIAN_POINT('',(21.3357142857143,40.9563385449745,9.52789761644379));
#78481=CARTESIAN_POINT('',(22.,40.3644845257006,9.33559258828708));
#78482=CARTESIAN_POINT('Ctrl Pts',(21.3357142857143,40.9563385449745,9.52789761644379));
#78483=CARTESIAN_POINT('Ctrl Pts',(21.6703423800909,40.6582137039501,9.43103098365865));
#78484=CARTESIAN_POINT('Ctrl Pts',(22.,40.3644845257006,9.33559258828708));
#78485=CARTESIAN_POINT('',(21.3357142857143,40.2331784341656,12.2267678919897));
#78486=CARTESIAN_POINT('Ctrl Pts',(21.3357142857143,40.2331784341656,12.2267678919897));
#78487=CARTESIAN_POINT('Ctrl Pts',(21.385443740297,40.5947584895701,10.8773327542167));
#78488=CARTESIAN_POINT('Ctrl Pts',(21.3357142857143,40.9563385449745,9.52789761644379));
#78489=CARTESIAN_POINT('',(22.,39.6244653040641,12.0973819220119));
#78490=CARTESIAN_POINT('Ctrl Pts',(22.,39.6244653040641,12.0973819220119));
#78491=CARTESIAN_POINT('Ctrl Pts',(21.670342377286,39.9265614345165,12.1615944367947));
#78492=CARTESIAN_POINT('Ctrl Pts',(21.3357142857143,40.2331784341656,12.2267678919897));
#78493=CARTESIAN_POINT('Origin',(22.,0.,0.));
#78494=CARTESIAN_POINT('Origin',(21.55,0.,0.));
#78495=CARTESIAN_POINT('',(21.3357142857143,38.6796176759911,16.4951409948251));
#78496=CARTESIAN_POINT('',(22.,38.1301486668543,16.2029831402613));
#78497=CARTESIAN_POINT('Ctrl Pts',(21.3357142857143,38.6796176759911,16.4951409948251));
#78498=CARTESIAN_POINT('Ctrl Pts',(21.6703423781672,38.4028427370355,16.3479771493348));
#78499=CARTESIAN_POINT('Ctrl Pts',(22.,38.1301486668543,16.2029831402613));
#78500=CARTESIAN_POINT('',(21.3357142857143,37.4987900870893,19.0274339311535));
#78501=CARTESIAN_POINT('Ctrl Pts',(21.3357142857143,37.4987900870893,19.0274339311535));
#78502=CARTESIAN_POINT('Ctrl Pts',(21.385443740297,38.0892038815402,17.7612874629893));
#78503=CARTESIAN_POINT('Ctrl Pts',(21.3357142857143,38.6796176759911,16.4951409948251));
#78504=CARTESIAN_POINT('',(22.,36.9217923151073,18.7943116990243));
#78505=CARTESIAN_POINT('Ctrl Pts',(22.,36.9217923151073,18.7943116990243));
#78506=CARTESIAN_POINT('Ctrl Pts',(21.6703423774372,37.2081485402251,18.9100071239031));
#78507=CARTESIAN_POINT('Ctrl Pts',(21.3357142857143,37.4987900870893,19.0274339311535));
#78508=CARTESIAN_POINT('Origin',(22.,0.,0.));
#78509=CARTESIAN_POINT('Origin',(21.55,0.,0.));
#78510=CARTESIAN_POINT('',(21.3357142857143,35.2276361967536,22.9611878610227));
#78511=CARTESIAN_POINT('',(22.,34.7372475355518,22.5780542486238));
#78512=CARTESIAN_POINT('Ctrl Pts',(21.3357142857143,35.2276361967536,22.9611878610227));
#78513=CARTESIAN_POINT('Ctrl Pts',(21.670342378474,34.9806208243921,22.7681983010704));
#78514=CARTESIAN_POINT('Ctrl Pts',(22.,34.7372475355518,22.5780542486238));
#78515=CARTESIAN_POINT('',(21.3357142857143,33.6250199785202,25.2499610186653));
#78516=CARTESIAN_POINT('Ctrl Pts',(21.3357142857143,33.6250199785202,25.2499610186653));
#78517=CARTESIAN_POINT('Ctrl Pts',(21.385443740297,34.4263280876369,24.105574439844));
#78518=CARTESIAN_POINT('Ctrl Pts',(21.3357142857143,35.2276361967536,22.9611878610227));
#78519=CARTESIAN_POINT('',(22.,33.0972693499844,24.9201858254425));
#78520=CARTESIAN_POINT('Ctrl Pts',(22.,33.0972693499844,24.9201858254425));
#78521=CARTESIAN_POINT('Ctrl Pts',(21.6703423824005,33.3591848769665,25.0838488110428));
#78522=CARTESIAN_POINT('Ctrl Pts',(21.3357142857143,33.6250199785202,25.2499610186653));
#78523=CARTESIAN_POINT('Origin',(22.,0.,0.));
#78524=CARTESIAN_POINT('Origin',(21.55,0.,0.));
#78525=CARTESIAN_POINT('',(21.3357142857143,30.7052808177218,28.7295706529848));
#78526=CARTESIAN_POINT('',(22.,30.288872715777,28.2671026036886));
#78527=CARTESIAN_POINT('Ctrl Pts',(21.3357142857143,30.7052808177218,28.7295706529848));
#78528=CARTESIAN_POINT('Ctrl Pts',(21.6703423793899,30.4955304487274,28.4966192681895));
#78529=CARTESIAN_POINT('Ctrl Pts',(22.,30.288872715777,28.2671026036886));
#78530=CARTESIAN_POINT('',(21.3357142857143,28.7295706529848,30.7052808177218));
#78531=CARTESIAN_POINT('Ctrl Pts',(21.3357142857143,28.7295706529848,30.7052808177218));
#78532=CARTESIAN_POINT('Ctrl Pts',(21.385443740297,29.7174257353533,29.7174257353533));
#78533=CARTESIAN_POINT('Ctrl Pts',(21.3357142857143,30.7052808177218,28.7295706529848));
#78534=CARTESIAN_POINT('',(22.,28.2671026036886,30.288872715777));
#78535=CARTESIAN_POINT('Ctrl Pts',(22.,28.2671026036886,30.288872715777));
#78536=CARTESIAN_POINT('Ctrl Pts',(21.6703423804808,28.4966192674301,30.4955304480436));
#78537=CARTESIAN_POINT('Ctrl Pts',(21.3357142857143,28.7295706529848,30.7052808177218));
#78538=CARTESIAN_POINT('Origin',(22.,0.,0.));
#78539=CARTESIAN_POINT('Origin',(21.55,0.,0.));
#78540=CARTESIAN_POINT('',(21.3357142857143,25.2499610186653,33.6250199785202));
#78541=CARTESIAN_POINT('',(22.,24.9201858254425,33.0972693499844));
#78542=CARTESIAN_POINT('Ctrl Pts',(21.3357142857143,25.2499610186653,33.6250199785202));
#78543=CARTESIAN_POINT('Ctrl Pts',(21.6703423822881,25.0838488110986,33.3591848770558));
#78544=CARTESIAN_POINT('Ctrl Pts',(22.,24.9201858254425,33.0972693499844));
#78545=CARTESIAN_POINT('',(21.3357142857143,22.9611878610227,35.2276361967536));
#78546=CARTESIAN_POINT('Ctrl Pts',(21.3357142857143,22.9611878610227,35.2276361967536));
#78547=CARTESIAN_POINT('Ctrl Pts',(21.385443740297,24.105574439844,34.4263280876369));
#78548=CARTESIAN_POINT('Ctrl Pts',(21.3357142857143,25.2499610186653,33.6250199785202));
#78549=CARTESIAN_POINT('',(22.,22.5780542486238,34.7372475355518));
#78550=CARTESIAN_POINT('Ctrl Pts',(22.,22.5780542486238,34.7372475355518));
#78551=CARTESIAN_POINT('Ctrl Pts',(21.6703423746987,22.7681983032475,34.9806208271787));
#78552=CARTESIAN_POINT('Ctrl Pts',(21.3357142857143,22.9611878610227,35.2276361967536));
#78553=CARTESIAN_POINT('Origin',(22.,0.,0.));
#78554=CARTESIAN_POINT('Origin',(21.55,0.,0.));
#78555=CARTESIAN_POINT('',(21.3357142857143,19.0274339311535,37.4987900870893));
#78556=CARTESIAN_POINT('',(22.,18.7943116990243,36.9217923151073));
#78557=CARTESIAN_POINT('Ctrl Pts',(21.3357142857143,19.0274339311535,37.4987900870893));
#78558=CARTESIAN_POINT('Ctrl Pts',(21.670342376995,18.9100071240582,37.2081485406091));
#78559=CARTESIAN_POINT('Ctrl Pts',(22.,18.7943116990243,36.9217923151073));
#78560=CARTESIAN_POINT('',(21.3357142857143,16.4951409948251,38.6796176759911));
#78561=CARTESIAN_POINT('Ctrl Pts',(21.3357142857143,16.4951409948251,38.6796176759911));
#78562=CARTESIAN_POINT('Ctrl Pts',(21.385443740297,17.7612874629893,38.0892038815402));
#78563=CARTESIAN_POINT('Ctrl Pts',(21.3357142857143,19.0274339311535,37.4987900870893));
#78564=CARTESIAN_POINT('',(22.,16.2029831402613,38.1301486668542));
#78565=CARTESIAN_POINT('Ctrl Pts',(22.,16.2029831402613,38.1301486668543));
#78566=CARTESIAN_POINT('Ctrl Pts',(21.6703423781921,16.3479771493239,38.4028427370149));
#78567=CARTESIAN_POINT('Ctrl Pts',(21.3357142857143,16.4951409948251,38.6796176759911));
#78568=CARTESIAN_POINT('Origin',(22.,0.,0.));
#78569=CARTESIAN_POINT('Origin',(21.55,0.,0.));
#78570=CARTESIAN_POINT('',(21.3357142857143,12.2267678919897,40.2331784341656));
#78571=CARTESIAN_POINT('',(22.,12.097381922012,39.6244653040641));
#78572=CARTESIAN_POINT('Ctrl Pts',(21.3357142857143,12.2267678919897,40.2331784341656));
#78573=CARTESIAN_POINT('Ctrl Pts',(21.6703423713064,12.1615944379593,39.9265614399951));
#78574=CARTESIAN_POINT('Ctrl Pts',(22.,12.097381922012,39.6244653040641));
#78575=CARTESIAN_POINT('',(21.3357142857143,9.5278976164438,40.9563385449745));
#78576=CARTESIAN_POINT('Ctrl Pts',(21.3357142857143,9.5278976164438,40.9563385449745));
#78577=CARTESIAN_POINT('Ctrl Pts',(21.385443740297,10.8773327542168,40.5947584895701));
#78578=CARTESIAN_POINT('Ctrl Pts',(21.3357142857143,12.2267678919897,40.2331784341656));
#78579=CARTESIAN_POINT('',(22.,9.33559258828709,40.3644845257006));
#78580=CARTESIAN_POINT('Ctrl Pts',(22.,9.33559258828708,40.3644845257006));
#78581=CARTESIAN_POINT('Ctrl Pts',(21.6703423800867,9.43103098365986,40.6582137039538));
#78582=CARTESIAN_POINT('Ctrl Pts',(21.3357142857143,9.5278976164438,40.9563385449745));
#78583=CARTESIAN_POINT('Origin',(22.,0.,0.));
#78584=CARTESIAN_POINT('Origin',(21.55,0.,0.));
#78585=CARTESIAN_POINT('',(21.3357142857143,5.05459769747092,41.7451020134904));
#78586=CARTESIAN_POINT('',(22.,5.03287931686986,41.1231689657038));
#78587=CARTESIAN_POINT('Ctrl Pts',(21.3357142857143,5.05459769747092,41.7451020134904));
#78588=CARTESIAN_POINT('Ctrl Pts',(21.6703423747022,5.04365785681953,41.4318259657226));
#78589=CARTESIAN_POINT('Ctrl Pts',(22.,5.03287931686986,41.1231689657038));
#78590=CARTESIAN_POINT('',(21.3357142857143,2.27115389033571,41.9886217921762));
#78591=CARTESIAN_POINT('Ctrl Pts',(21.3357142857143,2.27115389033571,41.9886217921762));
#78592=CARTESIAN_POINT('Ctrl Pts',(21.385443740297,3.66287579390336,41.8668619028333));
#78593=CARTESIAN_POINT('Ctrl Pts',(21.3357142857143,5.05459769747092,41.7451020134904));
#78594=CARTESIAN_POINT('',(22.,2.18454477955552,41.3723659476482));
#78595=CARTESIAN_POINT('Ctrl Pts',(22.,2.18454477955552,41.3723659476482));
#78596=CARTESIAN_POINT('Ctrl Pts',(21.670342377366,2.22752771507708,41.6782054256375));
#78597=CARTESIAN_POINT('Ctrl Pts',(21.3357142857143,2.27115389033571,41.9886217921762));
#78598=CARTESIAN_POINT('Origin',(22.,0.,0.));
#78599=CARTESIAN_POINT('Origin',(21.55,0.,0.));
#78600=CARTESIAN_POINT('',(21.3357142857143,-2.2711538903357,41.9886217921762));
#78601=CARTESIAN_POINT('',(22.,-2.18454477955551,41.3723659476482));
#78602=CARTESIAN_POINT('Ctrl Pts',(21.3357142857143,-2.2711538903357,41.9886217921762));
#78603=CARTESIAN_POINT('Ctrl Pts',(21.6703423740032,-2.22752771551545,41.6782054287567));
#78604=CARTESIAN_POINT('Ctrl Pts',(22.,-2.18454477955551,41.3723659476482));
#78605=CARTESIAN_POINT('',(21.3357142857143,-5.05459769747091,41.7451020134904));
#78606=CARTESIAN_POINT('Ctrl Pts',(21.3357142857143,-5.05459769747091,41.7451020134904));
#78607=CARTESIAN_POINT('Ctrl Pts',(21.385443740297,-3.66287579390327,41.8668619028333));
#78608=CARTESIAN_POINT('Ctrl Pts',(21.3357142857143,-2.27115389033571,41.9886217921762));
#78609=CARTESIAN_POINT('',(22.,-5.03287931686985,41.1231689657038));
#78610=CARTESIAN_POINT('Ctrl Pts',(22.,-5.03287931686985,41.1231689657038));
#78611=CARTESIAN_POINT('Ctrl Pts',(21.6703423749418,-5.04365785681169,41.4318259654982));
#78612=CARTESIAN_POINT('Ctrl Pts',(21.3357142857143,-5.05459769747091,41.7451020134904));
#78613=CARTESIAN_POINT('Origin',(22.,0.,0.));
#78614=CARTESIAN_POINT('Origin',(21.55,0.,0.));
#78615=CARTESIAN_POINT('',(21.3357142857143,-9.52789761644379,40.9563385449745));
#78616=CARTESIAN_POINT('',(22.,-9.33559258828708,40.3644845257006));
#78617=CARTESIAN_POINT('Ctrl Pts',(21.3357142857143,-9.52789761644379,40.9563385449745));
#78618=CARTESIAN_POINT('Ctrl Pts',(21.6703423801097,-9.43103098365321,40.6582137039333));
#78619=CARTESIAN_POINT('Ctrl Pts',(22.,-9.33559258828708,40.3644845257006));
#78620=CARTESIAN_POINT('',(21.3357142857143,-12.2267678919897,40.2331784341656));
#78621=CARTESIAN_POINT('Ctrl Pts',(21.3357142857143,-12.2267678919897,40.2331784341656));
#78622=CARTESIAN_POINT('Ctrl Pts',(21.385443740297,-10.8773327542167,40.5947584895701));
#78623=CARTESIAN_POINT('Ctrl Pts',(21.3357142857143,-9.52789761644379,40.9563385449745));
#78624=CARTESIAN_POINT('',(22.,-12.0973819220119,39.6244653040641));
#78625=CARTESIAN_POINT('Ctrl Pts',(22.,-12.0973819220119,39.6244653040641));
#78626=CARTESIAN_POINT('Ctrl Pts',(21.6703423772675,-12.1615944367983,39.9265614345335));
#78627=CARTESIAN_POINT('Ctrl Pts',(21.3357142857143,-12.2267678919897,40.2331784341656));
#78628=CARTESIAN_POINT('Origin',(22.,0.,0.));
#78629=CARTESIAN_POINT('Origin',(21.55,0.,0.));
#78630=CARTESIAN_POINT('',(21.3357142857143,-16.4951409948251,38.6796176759911));
#78631=CARTESIAN_POINT('',(22.,-16.2029831402613,38.1301486668543));
#78632=CARTESIAN_POINT('Ctrl Pts',(21.3357142857143,-16.4951409948251,38.6796176759911));
#78633=CARTESIAN_POINT('Ctrl Pts',(21.6703423749317,-16.3479771507576,38.4028427397114));
#78634=CARTESIAN_POINT('Ctrl Pts',(22.,-16.2029831402613,38.1301486668543));
#78635=CARTESIAN_POINT('',(21.3357142857143,-19.0274339311535,37.4987900870893));
#78636=CARTESIAN_POINT('Ctrl Pts',(21.3357142857143,-19.0274339311535,37.4987900870893));
#78637=CARTESIAN_POINT('Ctrl Pts',(21.385443740297,-17.7612874629893,38.0892038815402));
#78638=CARTESIAN_POINT('Ctrl Pts',(21.3357142857143,-16.4951409948251,38.6796176759911));
#78639=CARTESIAN_POINT('',(22.,-18.7943116990243,36.9217923151073));
#78640=CARTESIAN_POINT('Ctrl Pts',(22.,-18.7943116990243,36.9217923151073));
#78641=CARTESIAN_POINT('Ctrl Pts',(21.6703423742972,-18.9100071250049,37.2081485429521));
#78642=CARTESIAN_POINT('Ctrl Pts',(21.3357142857143,-19.0274339311535,37.4987900870893));
#78643=CARTESIAN_POINT('Origin',(22.,0.,0.));
#78644=CARTESIAN_POINT('Origin',(21.55,0.,0.));
#78645=CARTESIAN_POINT('',(21.3357142857143,-28.7295706529848,30.7052808177218));
#78646=CARTESIAN_POINT('',(22.,-28.2671026036886,30.288872715777));
#78647=CARTESIAN_POINT('Ctrl Pts',(21.3357142857143,-28.7295706529848,30.7052808177218));
#78648=CARTESIAN_POINT('Ctrl Pts',(21.6703423825864,-28.4966192659645,30.4955304467239));
#78649=CARTESIAN_POINT('Ctrl Pts',(22.,-28.2671026036886,30.288872715777));
#78650=CARTESIAN_POINT('',(21.3357142857143,-30.7052808177218,28.7295706529848));
#78651=CARTESIAN_POINT('Ctrl Pts',(21.3357142857143,-30.7052808177218,28.7295706529848));
#78652=CARTESIAN_POINT('Ctrl Pts',(21.385443740297,-29.7174257353533,29.7174257353533));
#78653=CARTESIAN_POINT('Ctrl Pts',(21.3357142857143,-28.7295706529848,30.7052808177218));
#78654=CARTESIAN_POINT('',(22.,-30.288872715777,28.2671026036886));
#78655=CARTESIAN_POINT('Ctrl Pts',(22.,-30.288872715777,28.2671026036886));
#78656=CARTESIAN_POINT('Ctrl Pts',(21.6703423803358,-30.4955304481345,28.4966192675311));
#78657=CARTESIAN_POINT('Ctrl Pts',(21.3357142857143,-30.7052808177218,28.7295706529848));
#78658=CARTESIAN_POINT('Origin',(22.,0.,0.));
#78659=CARTESIAN_POINT('Origin',(21.55,0.,0.));
#78660=CARTESIAN_POINT('',(21.3357142857143,-33.6250199785202,25.2499610186654));
#78661=CARTESIAN_POINT('',(22.,-33.0972693499844,24.9201858254425));
#78662=CARTESIAN_POINT('Ctrl Pts',(21.3357142857143,-33.6250199785202,25.2499610186654));
#78663=CARTESIAN_POINT('Ctrl Pts',(21.6703423791589,-33.3591848795415,25.0838488126518));
#78664=CARTESIAN_POINT('Ctrl Pts',(22.,-33.0972693499844,24.9201858254425));
#78665=CARTESIAN_POINT('',(21.3357142857143,-35.2276361967536,22.9611878610227));
#78666=CARTESIAN_POINT('Ctrl Pts',(21.3357142857143,-35.2276361967536,22.9611878610227));
#78667=CARTESIAN_POINT('Ctrl Pts',(21.385443740297,-34.4263280876369,24.1055744398441));
#78668=CARTESIAN_POINT('Ctrl Pts',(21.3357142857143,-33.6250199785202,25.2499610186654));
#78669=CARTESIAN_POINT('',(22.,-34.7372475355518,22.5780542486238));
#78670=CARTESIAN_POINT('Ctrl Pts',(22.,-34.7372475355518,22.5780542486238));
#78671=CARTESIAN_POINT('Ctrl Pts',(21.6703423746934,-34.9806208271825,22.7681983032506));
#78672=CARTESIAN_POINT('Ctrl Pts',(21.3357142857143,-35.2276361967536,22.9611878610227));
#78673=CARTESIAN_POINT('Origin',(22.,0.,0.));
#78674=CARTESIAN_POINT('Origin',(21.55,0.,0.));
#78675=CARTESIAN_POINT('',(21.3357142857143,-37.4987900870893,19.0274339311535));
#78676=CARTESIAN_POINT('',(22.,-36.9217923151073,18.7943116990243));
#78677=CARTESIAN_POINT('Ctrl Pts',(21.3357142857143,-37.4987900870893,19.0274339311535));
#78678=CARTESIAN_POINT('Ctrl Pts',(21.6703423777508,-37.2081485399528,18.9100071237931));
#78679=CARTESIAN_POINT('Ctrl Pts',(22.,-36.9217923151073,18.7943116990243));
#78680=CARTESIAN_POINT('',(21.3357142857143,-38.6796176759911,16.4951409948251));
#78681=CARTESIAN_POINT('Ctrl Pts',(21.3357142857143,-38.6796176759911,16.4951409948251));
#78682=CARTESIAN_POINT('Ctrl Pts',(21.385443740297,-38.0892038815402,17.7612874629893));
#78683=CARTESIAN_POINT('Ctrl Pts',(21.3357142857143,-37.4987900870893,19.0274339311535));
#78684=CARTESIAN_POINT('',(22.,-38.1301486668543,16.2029831402613));
#78685=CARTESIAN_POINT('Ctrl Pts',(22.,-38.1301486668543,16.2029831402613));
#78686=CARTESIAN_POINT('Ctrl Pts',(21.670342380746,-38.4028427349027,16.3479771482008));
#78687=CARTESIAN_POINT('Ctrl Pts',(21.3357142857143,-38.6796176759911,16.4951409948251));
#78688=CARTESIAN_POINT('Origin',(22.,0.,0.));
#78689=CARTESIAN_POINT('Origin',(21.55,0.,0.));
#78690=CARTESIAN_POINT('',(21.3357142857143,-40.2331784341656,12.2267678919897));
#78691=CARTESIAN_POINT('',(22.,-39.6244653040641,12.097381922012));
#78692=CARTESIAN_POINT('Ctrl Pts',(21.3357142857143,-40.2331784341656,12.2267678919897));
#78693=CARTESIAN_POINT('Ctrl Pts',(21.670342374299,-39.9265614372533,12.1615944373765));
#78694=CARTESIAN_POINT('Ctrl Pts',(22.,-39.6244653040641,12.097381922012));
#78695=CARTESIAN_POINT('',(21.3357142857143,-40.9563385449745,9.5278976164438));
#78696=CARTESIAN_POINT('Ctrl Pts',(21.3357142857143,-40.9563385449745,9.5278976164438));
#78697=CARTESIAN_POINT('Ctrl Pts',(21.385443740297,-40.5947584895701,10.8773327542168));
#78698=CARTESIAN_POINT('Ctrl Pts',(21.3357142857143,-40.2331784341656,12.2267678919897));
#78699=CARTESIAN_POINT('',(22.,-40.3644845257006,9.33559258828709));
#78700=CARTESIAN_POINT('Ctrl Pts',(22.,-40.3644845257006,9.33559258828709));
#78701=CARTESIAN_POINT('Ctrl Pts',(21.6703423770111,-40.6582137066937,9.4310309845501));
#78702=CARTESIAN_POINT('Ctrl Pts',(21.3357142857143,-40.9563385449745,9.5278976164438));
#78703=CARTESIAN_POINT('Origin',(22.,0.,0.));
#78704=CARTESIAN_POINT('Origin',(21.55,0.,0.));
#78705=CARTESIAN_POINT('',(21.3357142857143,-41.7451020134904,5.05459769747093));
#78706=CARTESIAN_POINT('',(22.,-41.1231689657038,5.03287931686987));
#78707=CARTESIAN_POINT('Ctrl Pts',(21.3357142857143,-41.7451020134904,5.05459769747093));
#78708=CARTESIAN_POINT('Ctrl Pts',(21.6703423749518,-41.4318259654889,5.04365785681138));
#78709=CARTESIAN_POINT('Ctrl Pts',(22.,-41.1231689657038,5.03287931686987));
#78710=CARTESIAN_POINT('',(21.3357142857143,-41.9886217921762,2.27115389033572));
#78711=CARTESIAN_POINT('Ctrl Pts',(21.3357142857143,-41.9886217921762,2.27115389033572));
#78712=CARTESIAN_POINT('Ctrl Pts',(21.385443740297,-41.8668619028333,3.66287579390337));
#78713=CARTESIAN_POINT('Ctrl Pts',(21.3357142857143,-41.7451020134904,5.05459769747093));
#78714=CARTESIAN_POINT('',(22.,-41.3723659476482,2.18454477955553));
#78715=CARTESIAN_POINT('Ctrl Pts',(22.,-41.3723659476482,2.18454477955553));
#78716=CARTESIAN_POINT('Ctrl Pts',(21.6703423713149,-41.6782054312502,2.22752771586591));
#78717=CARTESIAN_POINT('Ctrl Pts',(21.3357142857143,-41.9886217921762,2.27115389033572));
#78718=CARTESIAN_POINT('Origin',(22.,0.,0.));
#78719=CARTESIAN_POINT('Origin',(21.55,0.,0.));
#78720=CARTESIAN_POINT('',(21.3357142857143,-41.9886217921762,-2.2711538903357));
#78721=CARTESIAN_POINT('',(22.,-41.3723659476482,-2.18454477955551));
#78722=CARTESIAN_POINT('Ctrl Pts',(21.3357142857143,-41.9886217921762,-2.2711538903357));
#78723=CARTESIAN_POINT('Ctrl Pts',(21.6703423741524,-41.6782054286182,-2.22752771549599));
#78724=CARTESIAN_POINT('Ctrl Pts',(22.,-41.3723659476482,-2.18454477955551));
#78725=CARTESIAN_POINT('',(21.3357142857143,-41.7451020134904,-5.0545976974709));
#78726=CARTESIAN_POINT('Ctrl Pts',(21.3357142857143,-41.7451020134904,-5.0545976974709));
#78727=CARTESIAN_POINT('Ctrl Pts',(21.385443740297,-41.8668619028333,-3.66287579390326));
#78728=CARTESIAN_POINT('Ctrl Pts',(21.3357142857143,-41.9886217921762,-2.2711538903357));
#78729=CARTESIAN_POINT('',(22.,-41.1231689657038,-5.03287931686985));
#78730=CARTESIAN_POINT('Ctrl Pts',(22.,-41.1231689657038,-5.03287931686985));
#78731=CARTESIAN_POINT('Ctrl Pts',(21.6703423748145,-41.4318259656174,-5.04365785681585));
#78732=CARTESIAN_POINT('Ctrl Pts',(21.3357142857143,-41.7451020134904,-5.0545976974709));
#78733=CARTESIAN_POINT('Origin',(22.,0.,0.));
#78734=CARTESIAN_POINT('Origin',(21.55,0.,0.));
#78735=CARTESIAN_POINT('',(21.3357142857143,-40.9563385449745,-9.52789761644378));
#78736=CARTESIAN_POINT('',(22.,-40.3644845257006,-9.33559258828707));
#78737=CARTESIAN_POINT('Ctrl Pts',(21.3357142857143,-40.9563385449745,-9.52789761644378));
#78738=CARTESIAN_POINT('Ctrl Pts',(21.670342374081,-40.6582137093039,-9.43103098539821));
#78739=CARTESIAN_POINT('Ctrl Pts',(22.,-40.3644845257006,-9.33559258828707));
#78740=CARTESIAN_POINT('',(21.3357142857143,-40.2331784341656,-12.2267678919897));
#78741=CARTESIAN_POINT('Ctrl Pts',(21.3357142857143,-40.2331784341656,-12.2267678919897));
#78742=CARTESIAN_POINT('Ctrl Pts',(21.385443740297,-40.5947584895701,-10.8773327542167));
#78743=CARTESIAN_POINT('Ctrl Pts',(21.3357142857143,-40.9563385449745,-9.52789761644378));
#78744=CARTESIAN_POINT('',(22.,-39.6244653040641,-12.0973819220119));
#78745=CARTESIAN_POINT('Ctrl Pts',(22.,-39.6244653040641,-12.0973819220119));
#78746=CARTESIAN_POINT('Ctrl Pts',(21.6703423801992,-39.9265614318475,-12.1615944362274));
#78747=CARTESIAN_POINT('Ctrl Pts',(21.3357142857143,-40.2331784341656,-12.2267678919897));
#78748=CARTESIAN_POINT('Origin',(22.,0.,0.));
#78749=CARTESIAN_POINT('Origin',(21.55,0.,0.));
#78750=CARTESIAN_POINT('',(21.3357142857143,-38.6796176759911,-16.4951409948251));
#78751=CARTESIAN_POINT('',(22.,-38.1301486668543,-16.2029831402613));
#78752=CARTESIAN_POINT('Ctrl Pts',(21.3357142857143,-38.6796176759911,-16.4951409948251));
#78753=CARTESIAN_POINT('Ctrl Pts',(21.670342377579,-38.402842737522,-16.3479771495935));
#78754=CARTESIAN_POINT('Ctrl Pts',(22.,-38.1301486668543,-16.2029831402613));
#78755=CARTESIAN_POINT('',(21.3357142857143,-37.4987900870893,-19.0274339311535));
#78756=CARTESIAN_POINT('Ctrl Pts',(21.3357142857143,-37.4987900870893,-19.0274339311535));
#78757=CARTESIAN_POINT('Ctrl Pts',(21.385443740297,-38.0892038815402,-17.7612874629892));
#78758=CARTESIAN_POINT('Ctrl Pts',(21.3357142857143,-38.6796176759911,-16.4951409948251));
#78759=CARTESIAN_POINT('',(22.,-36.9217923151073,-18.7943116990243));
#78760=CARTESIAN_POINT('Ctrl Pts',(22.,-36.9217923151073,-18.7943116990243));
#78761=CARTESIAN_POINT('Ctrl Pts',(21.6703423805662,-37.2081485375077,-18.9100071228052));
#78762=CARTESIAN_POINT('Ctrl Pts',(21.3357142857143,-37.4987900870893,-19.0274339311535));
#78763=CARTESIAN_POINT('Origin',(22.,0.,0.));
#78764=CARTESIAN_POINT('Origin',(21.55,0.,0.));
#78765=CARTESIAN_POINT('',(21.3357142857143,-35.2276361967536,-22.9611878610227));
#78766=CARTESIAN_POINT('',(22.,-34.7372475355518,-22.5780542486238));
#78767=CARTESIAN_POINT('Ctrl Pts',(21.3357142857143,-35.2276361967536,-22.9611878610227));
#78768=CARTESIAN_POINT('Ctrl Pts',(21.6703423786233,-34.9806208242819,-22.7681983009843));
#78769=CARTESIAN_POINT('Ctrl Pts',(22.,-34.7372475355518,-22.5780542486238));
#78770=CARTESIAN_POINT('',(21.3357142857143,-33.6250199785202,-25.2499610186653));
#78771=CARTESIAN_POINT('Ctrl Pts',(21.3357142857143,-33.6250199785202,-25.2499610186653));
#78772=CARTESIAN_POINT('Ctrl Pts',(21.385443740297,-34.4263280876369,-24.105574439844));
#78773=CARTESIAN_POINT('Ctrl Pts',(21.3357142857143,-35.2276361967536,-22.9611878610227));
#78774=CARTESIAN_POINT('',(22.,-33.0972693499844,-24.9201858254425));
#78775=CARTESIAN_POINT('Ctrl Pts',(22.,-33.0972693499844,-24.9201858254425));
#78776=CARTESIAN_POINT('Ctrl Pts',(21.670342369686,-33.3591848870663,-25.0838488173538));
#78777=CARTESIAN_POINT('Ctrl Pts',(21.3357142857143,-33.6250199785202,-25.2499610186653));
#78778=CARTESIAN_POINT('Origin',(22.,0.,0.));
#78779=CARTESIAN_POINT('Origin',(21.55,0.,0.));
#78780=CARTESIAN_POINT('',(21.3357142857143,-30.7052808177218,-28.7295706529848));
#78781=CARTESIAN_POINT('',(22.,-30.288872715777,-28.2671026036886));
#78782=CARTESIAN_POINT('Ctrl Pts',(21.3357142857143,-30.7052808177218,-28.7295706529848));
#78783=CARTESIAN_POINT('Ctrl Pts',(21.6703423793899,-30.4955304487274,-28.4966192681895));
#78784=CARTESIAN_POINT('Ctrl Pts',(22.,-30.288872715777,-28.2671026036886));
#78785=CARTESIAN_POINT('',(21.3357142857143,-28.7295706529848,-30.7052808177218));
#78786=CARTESIAN_POINT('Ctrl Pts',(21.3357142857143,-28.7295706529848,-30.7052808177218));
#78787=CARTESIAN_POINT('Ctrl Pts',(21.385443740297,-29.7174257353533,-29.7174257353533));
#78788=CARTESIAN_POINT('Ctrl Pts',(21.3357142857143,-30.7052808177218,-28.7295706529848));
#78789=CARTESIAN_POINT('',(22.,-28.2671026036886,-30.288872715777));
#78790=CARTESIAN_POINT('Ctrl Pts',(22.,-28.2671026036886,-30.288872715777));
#78791=CARTESIAN_POINT('Ctrl Pts',(21.6703423804808,-28.4966192674301,-30.4955304480436));
#78792=CARTESIAN_POINT('Ctrl Pts',(21.3357142857143,-28.7295706529848,-30.7052808177218));
#78793=CARTESIAN_POINT('Origin',(22.,0.,0.));
#78794=CARTESIAN_POINT('Origin',(21.55,0.,0.));
#78795=CARTESIAN_POINT('',(21.3357142857143,-25.2499610186654,-33.6250199785202));
#78796=CARTESIAN_POINT('',(22.,-24.9201858254425,-33.0972693499844));
#78797=CARTESIAN_POINT('Ctrl Pts',(21.3357142857143,-25.2499610186654,-33.6250199785202));
#78798=CARTESIAN_POINT('Ctrl Pts',(21.6703423798578,-25.0838488123049,-33.3591848789864));
#78799=CARTESIAN_POINT('Ctrl Pts',(22.,-24.9201858254425,-33.0972693499844));
#78800=CARTESIAN_POINT('',(21.3357142857143,-22.9611878610227,-35.2276361967536));
#78801=CARTESIAN_POINT('Ctrl Pts',(21.3357142857143,-22.9611878610227,-35.2276361967536));
#78802=CARTESIAN_POINT('Ctrl Pts',(21.385443740297,-24.1055744398441,-34.4263280876369));
#78803=CARTESIAN_POINT('Ctrl Pts',(21.3357142857143,-25.2499610186654,-33.6250199785202));
#78804=CARTESIAN_POINT('',(22.,-22.5780542486238,-34.7372475355518));
#78805=CARTESIAN_POINT('Ctrl Pts',(22.,-22.5780542486238,-34.7372475355518));
#78806=CARTESIAN_POINT('Ctrl Pts',(21.670342374658,-22.768198303271,-34.9806208272087));
#78807=CARTESIAN_POINT('Ctrl Pts',(21.3357142857143,-22.9611878610227,-35.2276361967536));
#78808=CARTESIAN_POINT('Origin',(22.,0.,0.));
#78809=CARTESIAN_POINT('Origin',(21.55,0.,0.));
#78810=CARTESIAN_POINT('',(21.3357142857143,-12.2267678919898,-40.2331784341656));
#78811=CARTESIAN_POINT('',(22.,-12.097381922012,-39.6244653040641));
#78812=CARTESIAN_POINT('Ctrl Pts',(21.3357142857143,-12.2267678919898,-40.2331784341656));
#78813=CARTESIAN_POINT('Ctrl Pts',(21.6703423804963,-12.1615944361696,-39.9265614315752));
#78814=CARTESIAN_POINT('Ctrl Pts',(22.,-12.097381922012,-39.6244653040641));
#78815=CARTESIAN_POINT('',(21.3357142857143,-9.52789761644383,-40.9563385449745));
#78816=CARTESIAN_POINT('Ctrl Pts',(21.3357142857143,-9.52789761644383,-40.9563385449745));
#78817=CARTESIAN_POINT('Ctrl Pts',(21.385443740297,-10.8773327542168,-40.5947584895701));
#78818=CARTESIAN_POINT('Ctrl Pts',(21.3357142857143,-12.2267678919898,-40.2331784341656));
#78819=CARTESIAN_POINT('',(22.,-9.33559258828711,-40.3644845257006));
#78820=CARTESIAN_POINT('Ctrl Pts',(22.,-9.3355925882871,-40.3644845257006));
#78821=CARTESIAN_POINT('Ctrl Pts',(21.6703423830878,-9.43103098279123,-40.6582137012803));
#78822=CARTESIAN_POINT('Ctrl Pts',(21.3357142857143,-9.52789761644383,-40.9563385449745));
#78823=CARTESIAN_POINT('Origin',(22.,0.,0.));
#78824=CARTESIAN_POINT('Origin',(21.55,0.,0.));
#78825=CARTESIAN_POINT('',(21.3357142857143,-5.05459769747091,-41.7451020134904));
#78826=CARTESIAN_POINT('',(22.,-5.03287931686986,-41.1231689657038));
#78827=CARTESIAN_POINT('Ctrl Pts',(21.3357142857143,-5.05459769747091,-41.7451020134904));
#78828=CARTESIAN_POINT('Ctrl Pts',(21.6703423808798,-5.04365785661758,-41.4318259599396));
#78829=CARTESIAN_POINT('Ctrl Pts',(22.,-5.03287931686986,-41.1231689657038));
#78830=CARTESIAN_POINT('',(21.3357142857143,-2.27115389033571,-41.9886217921762));
#78831=CARTESIAN_POINT('Ctrl Pts',(21.3357142857143,-2.27115389033571,-41.9886217921762));
#78832=CARTESIAN_POINT('Ctrl Pts',(21.385443740297,-3.66287579390335,-41.8668619028333));
#78833=CARTESIAN_POINT('Ctrl Pts',(21.3357142857143,-5.05459769747091,-41.7451020134904));
#78834=CARTESIAN_POINT('',(22.,-2.18454477955551,-41.3723659476482));
#78835=CARTESIAN_POINT('Ctrl Pts',(22.,-2.18454477955551,-41.3723659476482));
#78836=CARTESIAN_POINT('Ctrl Pts',(21.670342377365,-2.2275277150772,-41.6782054256383));
#78837=CARTESIAN_POINT('Ctrl Pts',(21.3357142857143,-2.27115389033571,-41.9886217921762));
#78838=CARTESIAN_POINT('Origin',(22.,0.,0.));
#78839=CARTESIAN_POINT('Origin',(21.55,0.,0.));
#78840=CARTESIAN_POINT('',(21.3357142857143,2.2711538903357,-41.9886217921762));
#78841=CARTESIAN_POINT('',(22.,2.1845447795555,-41.3723659476482));
#78842=CARTESIAN_POINT('Ctrl Pts',(21.3357142857143,2.2711538903357,-41.9886217921762));
#78843=CARTESIAN_POINT('Ctrl Pts',(21.6703423741031,2.22752771550241,-41.678205428664));
#78844=CARTESIAN_POINT('Ctrl Pts',(22.,2.1845447795555,-41.3723659476482));
#78845=CARTESIAN_POINT('',(21.3357142857143,5.0545976974709,-41.7451020134904));
#78846=CARTESIAN_POINT('Ctrl Pts',(21.3357142857143,5.0545976974709,-41.7451020134904));
#78847=CARTESIAN_POINT('Ctrl Pts',(21.385443740297,3.66287579390326,-41.8668619028333));
#78848=CARTESIAN_POINT('Ctrl Pts',(21.3357142857143,2.2711538903357,-41.9886217921762));
#78849=CARTESIAN_POINT('',(22.,5.03287931686985,-41.1231689657038));
#78850=CARTESIAN_POINT('Ctrl Pts',(22.,5.03287931686985,-41.1231689657038));
#78851=CARTESIAN_POINT('Ctrl Pts',(21.6703423747918,5.04365785681659,-41.4318259656387));
#78852=CARTESIAN_POINT('Ctrl Pts',(21.3357142857143,5.0545976974709,-41.7451020134904));
#78853=CARTESIAN_POINT('Origin',(22.,0.,0.));
#78854=CARTESIAN_POINT('Origin',(21.55,0.,0.));
#78855=CARTESIAN_POINT('',(21.3357142857143,9.52789761644378,-40.9563385449745));
#78856=CARTESIAN_POINT('',(22.,9.33559258828707,-40.3644845257006));
#78857=CARTESIAN_POINT('Ctrl Pts',(21.3357142857143,9.52789761644378,-40.9563385449745));
#78858=CARTESIAN_POINT('Ctrl Pts',(21.670342374061,9.43103098540399,-40.6582137093217));
#78859=CARTESIAN_POINT('Ctrl Pts',(22.,9.33559258828707,-40.3644845257006));
#78860=CARTESIAN_POINT('',(21.3357142857143,12.2267678919897,-40.2331784341656));
#78861=CARTESIAN_POINT('Ctrl Pts',(21.3357142857143,12.2267678919897,-40.2331784341656));
#78862=CARTESIAN_POINT('Ctrl Pts',(21.385443740297,10.8773327542167,-40.5947584895701));
#78863=CARTESIAN_POINT('Ctrl Pts',(21.3357142857143,9.52789761644378,-40.9563385449745));
#78864=CARTESIAN_POINT('',(22.,12.0973819220119,-39.6244653040641));
#78865=CARTESIAN_POINT('Ctrl Pts',(22.,12.0973819220119,-39.6244653040641));
#78866=CARTESIAN_POINT('Ctrl Pts',(21.6703423744266,12.1615944373516,-39.9265614371364));
#78867=CARTESIAN_POINT('Ctrl Pts',(21.3357142857143,12.2267678919897,-40.2331784341656));
#78868=CARTESIAN_POINT('Origin',(22.,0.,0.));
#78869=CARTESIAN_POINT('Origin',(21.55,0.,0.));
#78870=CARTESIAN_POINT('',(21.3357142857143,16.4951409948251,-38.6796176759911));
#78871=CARTESIAN_POINT('',(22.,16.2029831402613,-38.1301486668543));
#78872=CARTESIAN_POINT('Ctrl Pts',(21.3357142857143,16.495140994825,-38.6796176759911));
#78873=CARTESIAN_POINT('Ctrl Pts',(21.6703423780787,16.3479771493738,-38.4028427371088));
#78874=CARTESIAN_POINT('Ctrl Pts',(22.,16.2029831402613,-38.1301486668543));
#78875=CARTESIAN_POINT('',(21.3357142857143,19.0274339311535,-37.4987900870893));
#78876=CARTESIAN_POINT('Ctrl Pts',(21.3357142857143,19.0274339311535,-37.4987900870893));
#78877=CARTESIAN_POINT('Ctrl Pts',(21.385443740297,17.7612874629892,-38.0892038815402));
#78878=CARTESIAN_POINT('Ctrl Pts',(21.3357142857143,16.4951409948251,-38.6796176759911));
#78879=CARTESIAN_POINT('',(22.,18.7943116990243,-36.9217923151073));
#78880=CARTESIAN_POINT('Ctrl Pts',(22.,18.7943116990243,-36.9217923151073));
#78881=CARTESIAN_POINT('Ctrl Pts',(21.6703423777322,18.9100071237995,-37.2081485399689));
#78882=CARTESIAN_POINT('Ctrl Pts',(21.3357142857143,19.0274339311535,-37.4987900870893));
#78883=CARTESIAN_POINT('Origin',(22.,0.,0.));
#78884=CARTESIAN_POINT('Origin',(21.55,0.,0.));
#78885=CARTESIAN_POINT('',(21.3357142857143,22.9611878610227,-35.2276361967536));
#78886=CARTESIAN_POINT('',(22.,22.5780542486238,-34.7372475355518));
#78887=CARTESIAN_POINT('Ctrl Pts',(21.3357142857143,22.9611878610227,-35.2276361967536));
#78888=CARTESIAN_POINT('Ctrl Pts',(21.6703423755923,22.7681983027322,-34.9806208265191));
#78889=CARTESIAN_POINT('Ctrl Pts',(22.,22.5780542486238,-34.7372475355518));
#78890=CARTESIAN_POINT('',(21.3357142857143,25.2499610186654,-33.6250199785202));
#78891=CARTESIAN_POINT('Ctrl Pts',(21.3357142857143,25.2499610186654,-33.6250199785202));
#78892=CARTESIAN_POINT('Ctrl Pts',(21.385443740297,24.105574439844,-34.4263280876369));
#78893=CARTESIAN_POINT('Ctrl Pts',(21.3357142857143,22.9611878610227,-35.2276361967536));
#78894=CARTESIAN_POINT('',(22.,24.9201858254425,-33.0972693499844));
#78895=CARTESIAN_POINT('Ctrl Pts',(22.,24.9201858254425,-33.0972693499844));
#78896=CARTESIAN_POINT('Ctrl Pts',(21.6703423766858,25.0838488138794,-33.359184881506));
#78897=CARTESIAN_POINT('Ctrl Pts',(21.3357142857143,25.2499610186654,-33.6250199785202));
#78898=CARTESIAN_POINT('Origin',(22.,0.,0.));
#78899=CARTESIAN_POINT('Origin',(21.55,0.,0.));
#78900=CARTESIAN_POINT('',(21.3357142857143,28.7295706529848,-30.7052808177218));
#78901=CARTESIAN_POINT('',(22.,28.2671026036886,-30.288872715777));
#78902=CARTESIAN_POINT('Ctrl Pts',(21.3357142857143,28.7295706529848,-30.7052808177218));
#78903=CARTESIAN_POINT('Ctrl Pts',(21.6703423805549,28.4966192673785,-30.4955304479972));
#78904=CARTESIAN_POINT('Ctrl Pts',(22.,28.2671026036886,-30.288872715777));
#78905=CARTESIAN_POINT('',(21.3357142857143,30.7052808177218,-28.7295706529848));
#78906=CARTESIAN_POINT('Ctrl Pts',(21.3357142857143,30.7052808177218,-28.7295706529848));
#78907=CARTESIAN_POINT('Ctrl Pts',(21.385443740297,29.7174257353533,-29.7174257353533));
#78908=CARTESIAN_POINT('Ctrl Pts',(21.3357142857143,28.7295706529848,-30.7052808177218));
#78909=CARTESIAN_POINT('',(22.,30.288872715777,-28.2671026036886));
#78910=CARTESIAN_POINT('Ctrl Pts',(22.,30.288872715777,-28.2671026036886));
#78911=CARTESIAN_POINT('Ctrl Pts',(21.6703423826323,30.4955304466952,-28.4966192659325));
#78912=CARTESIAN_POINT('Ctrl Pts',(21.3357142857143,30.7052808177218,-28.7295706529848));
#78913=CARTESIAN_POINT('Origin',(22.,0.,0.));
#78914=CARTESIAN_POINT('Origin',(21.55,0.,0.));
#78915=CARTESIAN_POINT('',(21.3357142857143,33.6250199785202,-25.2499610186654));
#78916=CARTESIAN_POINT('',(22.,33.0972693499844,-24.9201858254425));
#78917=CARTESIAN_POINT('Ctrl Pts',(21.3357142857143,33.6250199785202,-25.2499610186654));
#78918=CARTESIAN_POINT('Ctrl Pts',(21.6703423759705,33.3591848820742,-25.0838488142344));
#78919=CARTESIAN_POINT('Ctrl Pts',(22.,33.0972693499844,-24.9201858254425));
#78920=CARTESIAN_POINT('',(21.3357142857143,35.2276361967536,-22.9611878610227));
#78921=CARTESIAN_POINT('Ctrl Pts',(21.3357142857143,35.2276361967536,-22.9611878610227));
#78922=CARTESIAN_POINT('Ctrl Pts',(21.385443740297,34.4263280876368,-24.1055744398441));
#78923=CARTESIAN_POINT('Ctrl Pts',(21.3357142857143,33.6250199785202,-25.2499610186654));
#78924=CARTESIAN_POINT('',(22.,34.7372475355518,-22.5780542486238));
#78925=CARTESIAN_POINT('Ctrl Pts',(22.,34.7372475355518,-22.5780542486238));
#78926=CARTESIAN_POINT('Ctrl Pts',(21.6703423724652,34.9806208288272,-22.7681983045355));
#78927=CARTESIAN_POINT('Ctrl Pts',(21.3357142857143,35.2276361967536,-22.9611878610227));
#78928=CARTESIAN_POINT('Origin',(22.,0.,0.));
#78929=CARTESIAN_POINT('Origin',(21.55,0.,0.));
#78930=CARTESIAN_POINT('',(21.3357142857143,37.4987900870893,-19.0274339311535));
#78931=CARTESIAN_POINT('',(22.,36.9217923151073,-18.7943116990244));
#78932=CARTESIAN_POINT('Ctrl Pts',(21.3357142857143,37.4987900870893,-19.0274339311535));
#78933=CARTESIAN_POINT('Ctrl Pts',(21.6703423745627,37.2081485427215,-18.9100071249117));
#78934=CARTESIAN_POINT('Ctrl Pts',(22.,36.9217923151073,-18.7943116990244));
#78935=CARTESIAN_POINT('',(21.3357142857143,38.6796176759911,-16.4951409948251));
#78936=CARTESIAN_POINT('Ctrl Pts',(21.3357142857143,38.6796176759911,-16.4951409948251));
#78937=CARTESIAN_POINT('Ctrl Pts',(21.385443740297,38.0892038815402,-17.7612874629894));
#78938=CARTESIAN_POINT('Ctrl Pts',(21.3357142857143,37.4987900870893,-19.0274339311535));
#78939=CARTESIAN_POINT('',(22.,38.1301486668542,-16.2029831402614));
#78940=CARTESIAN_POINT('Ctrl Pts',(22.,38.1301486668542,-16.2029831402613));
#78941=CARTESIAN_POINT('Ctrl Pts',(21.670342378402,38.4028427368413,-16.3479771492316));
#78942=CARTESIAN_POINT('Ctrl Pts',(21.3357142857143,38.6796176759911,-16.4951409948251));
#78943=CARTESIAN_POINT('Origin',(22.,0.,0.));
#78944=CARTESIAN_POINT('Origin',(21.55,0.,0.));
#78945=CARTESIAN_POINT('',(21.3357142857143,40.2331784341656,-12.2267678919898));
#78946=CARTESIAN_POINT('',(22.,39.6244653040641,-12.097381922012));
#78947=CARTESIAN_POINT('Ctrl Pts',(21.3357142857143,40.2331784341656,-12.2267678919898));
#78948=CARTESIAN_POINT('Ctrl Pts',(21.6703423772556,39.9265614345444,-12.1615944368007));
#78949=CARTESIAN_POINT('Ctrl Pts',(22.,39.6244653040641,-12.097381922012));
#78950=CARTESIAN_POINT('',(21.3357142857143,40.9563385449745,-9.52789761644383));
#78951=CARTESIAN_POINT('Ctrl Pts',(21.3357142857143,40.9563385449745,-9.52789761644383));
#78952=CARTESIAN_POINT('Ctrl Pts',(21.385443740297,40.59475848957,-10.8773327542168));
#78953=CARTESIAN_POINT('Ctrl Pts',(21.3357142857143,40.2331784341656,-12.2267678919898));
#78954=CARTESIAN_POINT('',(22.,40.3644845257005,-9.33559258828711));
#78955=CARTESIAN_POINT('Ctrl Pts',(22.,40.3644845257005,-9.33559258828712));
#78956=CARTESIAN_POINT('Ctrl Pts',(21.6703423769138,40.6582137067803,-9.43103098457829));
#78957=CARTESIAN_POINT('Ctrl Pts',(21.3357142857143,40.9563385449745,-9.52789761644383));
#78958=CARTESIAN_POINT('Origin',(22.,0.,0.));
#78959=CARTESIAN_POINT('Origin',(21.55,0.,0.));
#78960=CARTESIAN_POINT('',(21.3357142857143,41.7451020134904,-5.05459769747091));
#78961=CARTESIAN_POINT('',(22.,41.1231689657038,-5.03287931686986));
#78962=CARTESIAN_POINT('Ctrl Pts',(21.3357142857143,41.7451020134904,-5.05459769747091));
#78963=CARTESIAN_POINT('Ctrl Pts',(21.6703423779714,41.4318259626622,-5.04365785671265));
#78964=CARTESIAN_POINT('Ctrl Pts',(22.,41.1231689657038,-5.03287931686986));
#78965=CARTESIAN_POINT('',(21.3357142857143,41.9886217921762,-2.27115389033571));
#78966=CARTESIAN_POINT('Ctrl Pts',(21.3357142857143,41.9886217921762,-2.27115389033571));
#78967=CARTESIAN_POINT('Ctrl Pts',(21.385443740297,41.8668619028333,-3.66287579390335));
#78968=CARTESIAN_POINT('Ctrl Pts',(21.3357142857143,41.7451020134904,-5.05459769747091));
#78969=CARTESIAN_POINT('',(22.,41.3723659476482,-2.18454477955551));
#78970=CARTESIAN_POINT('Ctrl Pts',(22.,41.3723659476482,-2.18454477955551));
#78971=CARTESIAN_POINT('Ctrl Pts',(21.6703423741537,41.678205428617,-2.22752771549582));
#78972=CARTESIAN_POINT('Ctrl Pts',(21.3357142857143,41.9886217921762,-2.27115389033571));
#78973=CARTESIAN_POINT('Origin',(22.,0.,0.));
#78974=CARTESIAN_POINT('Origin',(0.,41.9886217921762,-2.27115389033571));
#78975=CARTESIAN_POINT('',(0.66428571428571,41.9886217921762,-2.27115389033571));
#78976=CARTESIAN_POINT('',(0.,41.9886217921762,-2.27115389033571));
#78977=CARTESIAN_POINT('',(-6.93889390390723E-17,41.3723659476482,-2.18454477955551));
#78978=CARTESIAN_POINT('Ctrl Pts',(0.66428571428571,41.9886217921762,-2.27115389033571));
#78979=CARTESIAN_POINT('Ctrl Pts',(0.329657625802016,41.678205428576,-2.22752771549006));
#78980=CARTESIAN_POINT('Ctrl Pts',(6.93889390390723E-17,41.3723659476482,
-2.18454477955552));
#78981=CARTESIAN_POINT('',(0.,37.4643267032267,-1.63530568209483));
#78982=CARTESIAN_POINT('',(0.,41.9886217921762,-2.27115389033571));
#78983=CARTESIAN_POINT('',(0.,37.4643267032267,-1.63530568209483));
#78984=CARTESIAN_POINT('',(11.,37.7627704896084,-1.67724922094465));
#78985=CARTESIAN_POINT('',(22.,37.4643267032267,-1.63530568209483));
#78986=CARTESIAN_POINT('',(0.,37.4643267032267,-1.63530568209483));
#78987=CARTESIAN_POINT('',(22.,41.9886217921762,-2.27115389033571));
#78988=CARTESIAN_POINT('Origin',(0.,41.7451020134904,-5.05459769747091));
#78989=CARTESIAN_POINT('',(0.664285714285704,41.7451020134904,-5.05459769747091));
#78990=CARTESIAN_POINT('',(0.,41.7451020134904,-5.05459769747091));
#78991=CARTESIAN_POINT('Ctrl Pts',(0.664285714285704,41.7451020134904,-5.05459769747091));
#78992=CARTESIAN_POINT('Ctrl Pts',(0.614556259703002,41.8668619028333,-3.66287579390327));
#78993=CARTESIAN_POINT('Ctrl Pts',(0.66428571428571,41.9886217921762,-2.27115389033571));
#78994=CARTESIAN_POINT('Origin',(0.,40.9563385449745,-9.52789761644383));
#78995=CARTESIAN_POINT('',(0.664285714285704,40.9563385449745,-9.52789761644383));
#78996=CARTESIAN_POINT('',(0.,40.9563385449745,-9.52789761644383));
#78997=CARTESIAN_POINT('',(2.08166817117217E-16,40.3644845257005,-9.33559258828711));
#78998=CARTESIAN_POINT('Ctrl Pts',(0.664285714285704,40.9563385449745,-9.52789761644383));
#78999=CARTESIAN_POINT('Ctrl Pts',(0.329657628901705,40.658213711961,-9.43103098626159));
#79000=CARTESIAN_POINT('Ctrl Pts',(4.16333634234434E-16,40.3644845257005,
-9.33559258828712));
#79001=CARTESIAN_POINT('',(0.,36.6111915470958,-8.11607377380577));
#79002=CARTESIAN_POINT('',(0.,40.9563385449745,-9.52789761644383));
#79003=CARTESIAN_POINT('',(0.,36.6111915470958,-8.11607377380577));
#79004=CARTESIAN_POINT('',(11.,36.8978178826767,-8.20920431569504));
#79005=CARTESIAN_POINT('',(22.,36.6111915470958,-8.11607377380577));
#79006=CARTESIAN_POINT('',(0.,36.6111915470958,-8.11607377380577));
#79007=CARTESIAN_POINT('',(22.,40.9563385449745,-9.52789761644383));
#79008=CARTESIAN_POINT('Origin',(0.,40.2331784341656,-12.2267678919898));
#79009=CARTESIAN_POINT('',(0.664285714285704,40.2331784341656,-12.2267678919898));
#79010=CARTESIAN_POINT('',(0.,40.2331784341656,-12.2267678919898));
#79011=CARTESIAN_POINT('Ctrl Pts',(0.664285714285704,40.2331784341656,-12.2267678919898));
#79012=CARTESIAN_POINT('Ctrl Pts',(0.614556259703,40.5947584895701,-10.8773327542167));
#79013=CARTESIAN_POINT('Ctrl Pts',(0.664285714285704,40.9563385449745,-9.52789761644383));
#79014=CARTESIAN_POINT('Origin',(0.,38.6796176759911,-16.4951409948251));
#79015=CARTESIAN_POINT('',(0.664285714285706,38.6796176759911,-16.4951409948251));
#79016=CARTESIAN_POINT('',(0.,38.6796176759911,-16.4951409948251));
#79017=CARTESIAN_POINT('',(6.93889390390723E-17,38.1301486668542,-16.2029831402614));
#79018=CARTESIAN_POINT('Ctrl Pts',(0.664285714285706,38.6796176759911,-16.4951409948251));
#79019=CARTESIAN_POINT('Ctrl Pts',(0.329657628291304,38.402842742377,-16.347977152175));
#79020=CARTESIAN_POINT('Ctrl Pts',(-6.93889390390723E-17,38.1301486668542,
-16.2029831402614));
#79021=CARTESIAN_POINT('',(0.,34.6456438619633,-14.3502390708311));
#79022=CARTESIAN_POINT('',(0.,38.6796176759911,-16.4951409948251));
#79023=CARTESIAN_POINT('',(0.,34.6456438619633,-14.3502390708311));
#79024=CARTESIAN_POINT('',(11.,34.9117437505765,-14.4917268913708));
#79025=CARTESIAN_POINT('',(22.,34.6456438619633,-14.3502390708311));
#79026=CARTESIAN_POINT('',(0.,34.6456438619633,-14.3502390708311));
#79027=CARTESIAN_POINT('',(22.,38.6796176759911,-16.4951409948251));
#79028=CARTESIAN_POINT('Origin',(0.,37.4987900870893,-19.0274339311535));
#79029=CARTESIAN_POINT('',(0.664285714285706,37.4987900870893,-19.0274339311535));
#79030=CARTESIAN_POINT('',(0.,37.4987900870893,-19.0274339311535));
#79031=CARTESIAN_POINT('Ctrl Pts',(0.664285714285706,37.4987900870893,-19.0274339311535));
#79032=CARTESIAN_POINT('Ctrl Pts',(0.614556259703001,38.0892038815402,-17.7612874629893));
#79033=CARTESIAN_POINT('Ctrl Pts',(0.664285714285706,38.6796176759911,-16.4951409948251));
#79034=CARTESIAN_POINT('Origin',(0.,35.2276361967536,-22.9611878610227));
#79035=CARTESIAN_POINT('',(0.664285714285706,35.2276361967536,-22.9611878610227));
#79036=CARTESIAN_POINT('',(0.,35.2276361967536,-22.9611878610227));
#79037=CARTESIAN_POINT('',(7.63278329429795E-16,34.7372475355518,-22.5780542486238));
#79038=CARTESIAN_POINT('Ctrl Pts',(0.664285714285706,35.2276361967536,-22.9611878610227));
#79039=CARTESIAN_POINT('Ctrl Pts',(0.329657624533208,34.9806208266117,-22.7681983028046));
#79040=CARTESIAN_POINT('Ctrl Pts',(6.24500451351651E-16,34.7372475355518,
-22.5780542486238));
#79041=CARTESIAN_POINT('',(0.,31.6274058196267,-20.1483796152605));
#79042=CARTESIAN_POINT('',(0.,35.2276361967536,-22.9611878610227));
#79043=CARTESIAN_POINT('',(0.,31.6274058196267,-20.1483796152605));
#79044=CARTESIAN_POINT('',(11.,31.8648939508099,-20.3339256786199));
#79045=CARTESIAN_POINT('',(22.,31.6274058196267,-20.1483796152605));
#79046=CARTESIAN_POINT('',(0.,31.6274058196267,-20.1483796152605));
#79047=CARTESIAN_POINT('',(22.,35.2276361967536,-22.9611878610227));
#79048=CARTESIAN_POINT('Origin',(0.,33.6250199785202,-25.2499610186654));
#79049=CARTESIAN_POINT('',(0.66428571428571,33.6250199785202,-25.2499610186654));
#79050=CARTESIAN_POINT('',(0.,33.6250199785202,-25.2499610186654));
#79051=CARTESIAN_POINT('Ctrl Pts',(0.66428571428571,33.6250199785202,-25.2499610186654));
#79052=CARTESIAN_POINT('Ctrl Pts',(0.614556259703001,34.4263280876369,-24.105574439844));
#79053=CARTESIAN_POINT('Ctrl Pts',(0.664285714285706,35.2276361967536,-22.9611878610227));
#79054=CARTESIAN_POINT('Origin',(0.,30.7052808177218,-28.7295706529848));
#79055=CARTESIAN_POINT('',(0.664285714285712,30.7052808177218,-28.7295706529848));
#79056=CARTESIAN_POINT('',(0.,30.7052808177218,-28.7295706529848));
#79057=CARTESIAN_POINT('',(2.08166817117217E-16,30.288872715777,-28.2671026036886));
#79058=CARTESIAN_POINT('Ctrl Pts',(0.664285714285712,30.7052808177218,-28.7295706529848));
#79059=CARTESIAN_POINT('Ctrl Pts',(0.329657623601863,30.4955304506025,-28.4966192702721));
#79060=CARTESIAN_POINT('Ctrl Pts',(2.08166817117217E-16,30.288872715777,
-28.2671026036886));
#79061=CARTESIAN_POINT('',(0.,27.6481850557002,-25.3343218406523));
#79062=CARTESIAN_POINT('',(0.,30.7052808177218,-28.7295706529848));
#79063=CARTESIAN_POINT('',(0.,27.6481850557002,-25.3343218406523));
#79064=CARTESIAN_POINT('',(11.,27.8498454727622,-25.5582884235871));
#79065=CARTESIAN_POINT('',(22.,27.6481850557002,-25.3343218406523));
#79066=CARTESIAN_POINT('',(0.,27.6481850557002,-25.3343218406523));
#79067=CARTESIAN_POINT('',(22.,30.7052808177218,-28.7295706529848));
#79068=CARTESIAN_POINT('Origin',(0.,28.7295706529848,-30.7052808177218));
#79069=CARTESIAN_POINT('',(0.664285714285712,28.7295706529848,-30.7052808177218));
#79070=CARTESIAN_POINT('',(0.,28.7295706529848,-30.7052808177218));
#79071=CARTESIAN_POINT('Ctrl Pts',(0.664285714285712,28.7295706529848,-30.7052808177218));
#79072=CARTESIAN_POINT('Ctrl Pts',(0.614556259703005,29.7174257353533,-29.7174257353533));
#79073=CARTESIAN_POINT('Ctrl Pts',(0.664285714285712,30.7052808177218,-28.7295706529848));
#79074=CARTESIAN_POINT('Origin',(0.,25.2499610186654,-33.6250199785202));
#79075=CARTESIAN_POINT('',(0.664285714285713,25.2499610186654,-33.6250199785202));
#79076=CARTESIAN_POINT('',(0.,25.2499610186654,-33.6250199785202));
#79077=CARTESIAN_POINT('',(4.16333634234434E-16,24.9201858254425,-33.0972693499844));
#79078=CARTESIAN_POINT('Ctrl Pts',(0.664285714285713,25.2499610186654,-33.6250199785202));
#79079=CARTESIAN_POINT('Ctrl Pts',(0.329657620247448,25.0838488123571,-33.3591848790699));
#79080=CARTESIAN_POINT('Ctrl Pts',(3.46944695195361E-16,24.9201858254425,
-33.0972693499844));
#79081=CARTESIAN_POINT('',(0.,22.8288881795131,-29.7504935167013));
#79082=CARTESIAN_POINT('',(0.,25.2499610186654,-33.6250199785202));
#79083=CARTESIAN_POINT('',(0.,22.8288881795131,-29.7504935167013));
#79084=CARTESIAN_POINT('',(11.,22.9885935327265,-30.0060755079215));
#79085=CARTESIAN_POINT('',(22.,22.8288881795131,-29.7504935167013));
#79086=CARTESIAN_POINT('',(0.,22.8288881795131,-29.7504935167013));
#79087=CARTESIAN_POINT('',(22.,25.2499610186654,-33.6250199785202));
#79088=CARTESIAN_POINT('Origin',(0.,22.9611878610227,-35.2276361967536));
#79089=CARTESIAN_POINT('',(0.664285714285709,22.9611878610227,-35.2276361967536));
#79090=CARTESIAN_POINT('',(0.,22.9611878610227,-35.2276361967536));
#79091=CARTESIAN_POINT('Ctrl Pts',(0.664285714285709,22.9611878610227,-35.2276361967536));
#79092=CARTESIAN_POINT('Ctrl Pts',(0.614556259703007,24.105574439844,-34.4263280876369));
#79093=CARTESIAN_POINT('Ctrl Pts',(0.664285714285713,25.2499610186654,-33.6250199785202));
#79094=CARTESIAN_POINT('Origin',(0.,19.0274339311535,-37.4987900870893));
#79095=CARTESIAN_POINT('',(0.664285714285708,19.0274339311535,-37.4987900870893));
#79096=CARTESIAN_POINT('',(0.,19.0274339311535,-37.4987900870893));
#79097=CARTESIAN_POINT('',(6.93889390390723E-17,18.7943116990243,-36.9217923151073));
#79098=CARTESIAN_POINT('Ctrl Pts',(0.664285714285708,19.0274339311535,-37.4987900870893));
#79099=CARTESIAN_POINT('Ctrl Pts',(0.329657620121465,18.9100071230464,-37.2081485381049));
#79100=CARTESIAN_POINT('Ctrl Pts',(6.93889390390723E-17,18.7943116990243,
-36.9217923151073));
#79101=CARTESIAN_POINT('',(0.,17.3159470879662,-33.2627115017215));
#79102=CARTESIAN_POINT('',(0.,19.0274339311535,-37.4987900870893));
#79103=CARTESIAN_POINT('',(0.,17.3159470879662,-33.2627115017215));
#79104=CARTESIAN_POINT('',(11.,17.4288448109885,-33.5421431717545));
#79105=CARTESIAN_POINT('',(22.,17.3159470879662,-33.2627115017215));
#79106=CARTESIAN_POINT('',(0.,17.3159470879662,-33.2627115017215));
#79107=CARTESIAN_POINT('',(22.,19.0274339311535,-37.4987900870893));
#79108=CARTESIAN_POINT('Origin',(0.,16.4951409948251,-38.6796176759911));
#79109=CARTESIAN_POINT('',(0.664285714285715,16.4951409948251,-38.6796176759911));
#79110=CARTESIAN_POINT('',(0.,16.4951409948251,-38.6796176759911));
#79111=CARTESIAN_POINT('Ctrl Pts',(0.664285714285715,16.4951409948251,-38.6796176759911));
#79112=CARTESIAN_POINT('Ctrl Pts',(0.614556259703004,17.7612874629893,-38.0892038815402));
#79113=CARTESIAN_POINT('Ctrl Pts',(0.664285714285708,19.0274339311535,-37.4987900870893));
#79114=CARTESIAN_POINT('Origin',(0.,12.2267678919897,-40.2331784341656));
#79115=CARTESIAN_POINT('',(0.664285714285713,12.2267678919897,-40.2331784341656));
#79116=CARTESIAN_POINT('',(0.,12.2267678919897,-40.2331784341656));
#79117=CARTESIAN_POINT('',(6.93889390390723E-17,12.0973819220119,-39.6244653040641));
#79118=CARTESIAN_POINT('Ctrl Pts',(0.664285714285713,12.2267678919897,-40.2331784341656));
#79119=CARTESIAN_POINT('Ctrl Pts',(0.329657622858237,12.1615944368228,-39.9265614346487));
#79120=CARTESIAN_POINT('Ctrl Pts',(-1.38777878078145E-16,12.0973819220119,
-39.6244653040641));
#79121=CARTESIAN_POINT('',(0.,11.2768697064435,-35.764258829506));
#79122=CARTESIAN_POINT('',(0.,12.2267678919897,-40.2331784341656));
#79123=CARTESIAN_POINT('',(0.,11.2768697064435,-35.764258829506));
#79124=CARTESIAN_POINT('',(11.,11.3395294590896,-36.0590497884573));
#79125=CARTESIAN_POINT('',(22.,11.2768697064435,-35.764258829506));
#79126=CARTESIAN_POINT('',(0.,11.2768697064435,-35.764258829506));
#79127=CARTESIAN_POINT('',(22.,12.2267678919897,-40.2331784341656));
#79128=CARTESIAN_POINT('Origin',(0.,9.52789761644378,-40.9563385449745));
#79129=CARTESIAN_POINT('',(0.664285714285714,9.52789761644378,-40.9563385449745));
#79130=CARTESIAN_POINT('',(0.,9.52789761644378,-40.9563385449745));
#79131=CARTESIAN_POINT('Ctrl Pts',(0.664285714285714,9.52789761644378,-40.9563385449745));
#79132=CARTESIAN_POINT('Ctrl Pts',(0.614556259703009,10.8773327542168,-40.5947584895701));
#79133=CARTESIAN_POINT('Ctrl Pts',(0.664285714285713,12.2267678919897,-40.2331784341656));
#79134=CARTESIAN_POINT('Origin',(0.,5.0545976974709,-41.7451020134904));
#79135=CARTESIAN_POINT('',(0.664285714285704,5.0545976974709,-41.7451020134904));
#79136=CARTESIAN_POINT('',(0.,5.0545976974709,-41.7451020134904));
#79137=CARTESIAN_POINT('',(6.93889390390723E-17,5.03287931686985,-41.1231689657038));
#79138=CARTESIAN_POINT('Ctrl Pts',(0.664285714285704,5.0545976974709,-41.7451020134904));
#79139=CARTESIAN_POINT('Ctrl Pts',(0.329657625028856,5.04365785681072,-41.4318259654708));
#79140=CARTESIAN_POINT('Ctrl Pts',(-6.93889390390723E-17,5.03287931686985,
-41.1231689657038));
#79141=CARTESIAN_POINT('',(0.,4.89515034526193,-37.1791272503441));
#79142=CARTESIAN_POINT('',(0.,5.0545976974709,-41.7451020134904));
#79143=CARTESIAN_POINT('',(0.,4.89515034526193,-37.1791272503441));
#79144=CARTESIAN_POINT('',(11.,4.90566824265506,-37.4803204240973));
#79145=CARTESIAN_POINT('',(22.,4.89515034526193,-37.1791272503441));
#79146=CARTESIAN_POINT('',(0.,4.89515034526193,-37.1791272503441));
#79147=CARTESIAN_POINT('',(22.,5.0545976974709,-41.7451020134904));
#79148=CARTESIAN_POINT('Origin',(0.,2.2711538903357,-41.9886217921762));
#79149=CARTESIAN_POINT('',(0.6642857142857,2.2711538903357,-41.9886217921762));
#79150=CARTESIAN_POINT('',(0.,2.2711538903357,-41.9886217921762));
#79151=CARTESIAN_POINT('Ctrl Pts',(0.6642857142857,2.2711538903357,-41.9886217921762));
#79152=CARTESIAN_POINT('Ctrl Pts',(0.614556259702998,3.66287579390334,-41.8668619028333));
#79153=CARTESIAN_POINT('Ctrl Pts',(0.664285714285704,5.0545976974709,-41.7451020134904));
#79154=CARTESIAN_POINT('Origin',(0.,-2.27115389033571,-41.9886217921762));
#79155=CARTESIAN_POINT('',(0.6642857142857,-2.27115389033571,-41.9886217921762));
#79156=CARTESIAN_POINT('',(0.,-2.27115389033571,-41.9886217921762));
#79157=CARTESIAN_POINT('',(-6.93889390390723E-17,-2.18454477955551,-41.3723659476482));
#79158=CARTESIAN_POINT('Ctrl Pts',(0.6642857142857,-2.27115389033571,-41.9886217921762));
#79159=CARTESIAN_POINT('Ctrl Pts',(0.329657622906579,-2.2275277151126,-41.6782054258903));
#79160=CARTESIAN_POINT('Ctrl Pts',(-6.93889390390723E-17,-2.18454477955551,
-41.3723659476482));
#79161=CARTESIAN_POINT('',(0.,-1.63530568209482,-37.4643267032267));
#79162=CARTESIAN_POINT('',(0.,-2.27115389033571,-41.9886217921762));
#79163=CARTESIAN_POINT('',(0.,-1.63530568209482,-37.4643267032267));
#79164=CARTESIAN_POINT('',(11.,-1.67724922094465,-37.7627704896084));
#79165=CARTESIAN_POINT('',(22.,-1.63530568209482,-37.4643267032267));
#79166=CARTESIAN_POINT('',(0.,-1.63530568209482,-37.4643267032267));
#79167=CARTESIAN_POINT('',(22.,-2.27115389033571,-41.9886217921762));
#79168=CARTESIAN_POINT('Origin',(0.,-5.05459769747091,-41.7451020134904));
#79169=CARTESIAN_POINT('',(0.664285714285704,-5.05459769747091,-41.7451020134904));
#79170=CARTESIAN_POINT('',(0.,-5.05459769747091,-41.7451020134904));
#79171=CARTESIAN_POINT('Ctrl Pts',(0.664285714285704,-5.05459769747091,
-41.7451020134904));
#79172=CARTESIAN_POINT('Ctrl Pts',(0.614556259702995,-3.66287579390326,
-41.8668619028333));
#79173=CARTESIAN_POINT('Ctrl Pts',(0.6642857142857,-2.27115389033571,-41.9886217921762));
#79174=CARTESIAN_POINT('Origin',(0.,-9.52789761644383,-40.9563385449745));
#79175=CARTESIAN_POINT('',(0.664285714285723,-9.52789761644383,-40.9563385449745));
#79176=CARTESIAN_POINT('',(0.,-9.52789761644383,-40.9563385449745));
#79177=CARTESIAN_POINT('',(-1.38777878078145E-16,-9.33559258828711,-40.3644845257006));
#79178=CARTESIAN_POINT('Ctrl Pts',(0.664285714285723,-9.52789761644383,
-40.9563385449745));
#79179=CARTESIAN_POINT('Ctrl Pts',(0.329657616731471,-9.4310309827389,-40.6582137011193));
#79180=CARTESIAN_POINT('Ctrl Pts',(-2.08166817117217E-16,-9.3355925882871,
-40.3644845257006));
#79181=CARTESIAN_POINT('',(0.,-8.11607377380577,-36.6111915470959));
#79182=CARTESIAN_POINT('',(0.,-9.52789761644383,-40.9563385449745));
#79183=CARTESIAN_POINT('',(0.,-8.11607377380577,-36.6111915470959));
#79184=CARTESIAN_POINT('',(11.,-8.20920431569503,-36.8978178826767));
#79185=CARTESIAN_POINT('',(22.,-8.11607377380577,-36.6111915470959));
#79186=CARTESIAN_POINT('',(0.,-8.11607377380577,-36.6111915470959));
#79187=CARTESIAN_POINT('',(22.,-9.52789761644383,-40.9563385449745));
#79188=CARTESIAN_POINT('Origin',(0.,-12.2267678919898,-40.2331784341656));
#79189=CARTESIAN_POINT('',(0.664285714285714,-12.2267678919898,-40.2331784341656));
#79190=CARTESIAN_POINT('',(0.,-12.2267678919898,-40.2331784341656));
#79191=CARTESIAN_POINT('Ctrl Pts',(0.664285714285714,-12.2267678919898,
-40.2331784341656));
#79192=CARTESIAN_POINT('Ctrl Pts',(0.614556259703017,-10.8773327542167,
-40.5947584895701));
#79193=CARTESIAN_POINT('Ctrl Pts',(0.664285714285723,-9.52789761644383,
-40.9563385449745));
#79194=CARTESIAN_POINT('Origin',(0.,-22.9611878610227,-35.2276361967536));
#79195=CARTESIAN_POINT('',(0.664285714285713,-22.9611878610227,-35.2276361967536));
#79196=CARTESIAN_POINT('',(0.,-22.9611878610227,-35.2276361967536));
#79197=CARTESIAN_POINT('',(2.08166817117217E-16,-22.5780542486238,-34.7372475355518));
#79198=CARTESIAN_POINT('Ctrl Pts',(0.664285714285713,-22.9611878610227,
-35.2276361967536));
#79199=CARTESIAN_POINT('Ctrl Pts',(0.329657622232873,-22.768198301478,-34.9806208249138));
#79200=CARTESIAN_POINT('Ctrl Pts',(-1.38777878078145E-16,-22.5780542486238,
-34.7372475355518));
#79201=CARTESIAN_POINT('',(0.,-20.1483796152605,-31.6274058196267));
#79202=CARTESIAN_POINT('',(0.,-22.9611878610227,-35.2276361967536));
#79203=CARTESIAN_POINT('',(0.,-20.1483796152605,-31.6274058196267));
#79204=CARTESIAN_POINT('',(11.,-20.3339256786199,-31.8648939508099));
#79205=CARTESIAN_POINT('',(22.,-20.1483796152605,-31.6274058196267));
#79206=CARTESIAN_POINT('',(0.,-20.1483796152605,-31.6274058196267));
#79207=CARTESIAN_POINT('',(22.,-22.9611878610227,-35.2276361967536));
#79208=CARTESIAN_POINT('Origin',(0.,-25.2499610186654,-33.6250199785202));
#79209=CARTESIAN_POINT('',(0.664285714285703,-25.2499610186654,-33.6250199785202));
#79210=CARTESIAN_POINT('',(0.,-25.2499610186654,-33.6250199785202));
#79211=CARTESIAN_POINT('Ctrl Pts',(0.664285714285703,-25.2499610186654,
-33.6250199785202));
#79212=CARTESIAN_POINT('Ctrl Pts',(0.614556259703008,-24.105574439844,-34.4263280876369));
#79213=CARTESIAN_POINT('Ctrl Pts',(0.664285714285713,-22.9611878610227,
-35.2276361967536));
#79214=CARTESIAN_POINT('Origin',(0.,-28.7295706529848,-30.7052808177218));
#79215=CARTESIAN_POINT('',(0.664285714285715,-28.7295706529848,-30.7052808177218));
#79216=CARTESIAN_POINT('',(0.,-28.7295706529848,-30.7052808177218));
#79217=CARTESIAN_POINT('',(0.,-28.2671026036886,-30.288872715777));
#79218=CARTESIAN_POINT('Ctrl Pts',(0.664285714285715,-28.7295706529848,
-30.7052808177218));
#79219=CARTESIAN_POINT('Ctrl Pts',(0.329657620568989,-28.4966192681609,
-30.4955304487016));
#79220=CARTESIAN_POINT('Ctrl Pts',(-2.77555756156289E-16,-28.2671026036886,
-30.288872715777));
#79221=CARTESIAN_POINT('',(0.,-25.3343218406523,-27.6481850557002));
#79222=CARTESIAN_POINT('',(0.,-28.7295706529848,-30.7052808177218));
#79223=CARTESIAN_POINT('',(0.,-25.3343218406523,-27.6481850557002));
#79224=CARTESIAN_POINT('',(11.,-25.5582884235871,-27.8498454727622));
#79225=CARTESIAN_POINT('',(22.,-25.3343218406523,-27.6481850557002));
#79226=CARTESIAN_POINT('',(0.,-25.3343218406523,-27.6481850557002));
#79227=CARTESIAN_POINT('',(22.,-28.7295706529848,-30.7052808177218));
#79228=CARTESIAN_POINT('Origin',(0.,-30.7052808177218,-28.7295706529848));
#79229=CARTESIAN_POINT('',(0.664285714285712,-30.7052808177218,-28.7295706529848));
#79230=CARTESIAN_POINT('',(0.,-30.7052808177218,-28.7295706529848));
#79231=CARTESIAN_POINT('Ctrl Pts',(0.664285714285712,-30.7052808177218,
-28.7295706529848));
#79232=CARTESIAN_POINT('Ctrl Pts',(0.614556259703008,-29.7174257353533,
-29.7174257353533));
#79233=CARTESIAN_POINT('Ctrl Pts',(0.664285714285715,-28.7295706529848,
-30.7052808177218));
#79234=CARTESIAN_POINT('Origin',(0.,-33.6250199785202,-25.2499610186653));
#79235=CARTESIAN_POINT('',(0.664285714285705,-33.6250199785202,-25.2499610186653));
#79236=CARTESIAN_POINT('',(0.,-33.6250199785202,-25.2499610186653));
#79237=CARTESIAN_POINT('',(1.38777878078145E-16,-33.0972693499844,-24.9201858254425));
#79238=CARTESIAN_POINT('Ctrl Pts',(0.664285714285705,-33.6250199785202,
-25.2499610186653));
#79239=CARTESIAN_POINT('Ctrl Pts',(0.329657617838466,-33.3591848771564,
-25.0838488111614));
#79240=CARTESIAN_POINT('Ctrl Pts',(0.,-33.0972693499844,-24.9201858254425));
#79241=CARTESIAN_POINT('',(0.,-29.7504935167013,-22.8288881795131));
#79242=CARTESIAN_POINT('',(0.,-33.6250199785202,-25.2499610186653));
#79243=CARTESIAN_POINT('',(0.,-29.7504935167013,-22.8288881795131));
#79244=CARTESIAN_POINT('',(11.,-30.0060755079215,-22.9885935327265));
#79245=CARTESIAN_POINT('',(22.,-29.7504935167013,-22.8288881795131));
#79246=CARTESIAN_POINT('',(0.,-29.7504935167013,-22.8288881795131));
#79247=CARTESIAN_POINT('',(22.,-33.6250199785202,-25.2499610186653));
#79248=CARTESIAN_POINT('Origin',(0.,-35.2276361967536,-22.9611878610227));
#79249=CARTESIAN_POINT('',(0.664285714285712,-35.2276361967536,-22.9611878610227));
#79250=CARTESIAN_POINT('',(0.,-35.2276361967536,-22.9611878610227));
#79251=CARTESIAN_POINT('Ctrl Pts',(0.664285714285712,-35.2276361967536,
-22.9611878610227));
#79252=CARTESIAN_POINT('Ctrl Pts',(0.614556259703,-34.4263280876369,-24.105574439844));
#79253=CARTESIAN_POINT('Ctrl Pts',(0.664285714285705,-33.6250199785202,
-25.2499610186653));
#79254=CARTESIAN_POINT('Origin',(0.,-37.4987900870893,-19.0274339311535));
#79255=CARTESIAN_POINT('',(0.664285714285717,-37.4987900870893,-19.0274339311535));
#79256=CARTESIAN_POINT('',(0.,-37.4987900870893,-19.0274339311535));
#79257=CARTESIAN_POINT('',(0.,-36.9217923151073,-18.7943116990243));
#79258=CARTESIAN_POINT('Ctrl Pts',(0.664285714285717,-37.4987900870893,
-19.0274339311535));
#79259=CARTESIAN_POINT('Ctrl Pts',(0.329657623220786,-37.2081485407966,
-18.910007124134));
#79260=CARTESIAN_POINT('Ctrl Pts',(-6.93889390390723E-17,-36.9217923151073,
-18.7943116990243));
#79261=CARTESIAN_POINT('',(0.,-33.2627115017215,-17.3159470879662));
#79262=CARTESIAN_POINT('',(0.,-37.4987900870893,-19.0274339311535));
#79263=CARTESIAN_POINT('',(0.,-33.2627115017215,-17.3159470879662));
#79264=CARTESIAN_POINT('',(11.,-33.5421431717545,-17.4288448109885));
#79265=CARTESIAN_POINT('',(22.,-33.2627115017215,-17.3159470879662));
#79266=CARTESIAN_POINT('',(0.,-33.2627115017215,-17.3159470879662));
#79267=CARTESIAN_POINT('',(22.,-37.4987900870893,-19.0274339311535));
#79268=CARTESIAN_POINT('Origin',(0.,-38.6796176759911,-16.4951409948251));
#79269=CARTESIAN_POINT('',(0.664285714285701,-38.6796176759911,-16.4951409948251));
#79270=CARTESIAN_POINT('',(0.,-38.6796176759911,-16.4951409948251));
#79271=CARTESIAN_POINT('Ctrl Pts',(0.664285714285701,-38.6796176759911,
-16.4951409948251));
#79272=CARTESIAN_POINT('Ctrl Pts',(0.614556259703013,-38.0892038815402,
-17.7612874629893));
#79273=CARTESIAN_POINT('Ctrl Pts',(0.664285714285718,-37.4987900870893,
-19.0274339311535));
#79274=CARTESIAN_POINT('Origin',(0.,-40.2331784341656,-12.2267678919897));
#79275=CARTESIAN_POINT('',(0.664285714285713,-40.2331784341656,-12.2267678919897));
#79276=CARTESIAN_POINT('',(0.,-40.2331784341656,-12.2267678919897));
#79277=CARTESIAN_POINT('',(6.93889390390723E-17,-39.6244653040641,-12.0973819220119));
#79278=CARTESIAN_POINT('Ctrl Pts',(0.664285714285713,-40.2331784341656,
-12.2267678919897));
#79279=CARTESIAN_POINT('Ctrl Pts',(0.329657622776605,-39.9265614345739,
-12.1615944368069));
#79280=CARTESIAN_POINT('Ctrl Pts',(0.,-39.6244653040641,-12.0973819220119));
#79281=CARTESIAN_POINT('',(0.,-35.764258829506,-11.2768697064435));
#79282=CARTESIAN_POINT('',(0.,-40.2331784341656,-12.2267678919897));
#79283=CARTESIAN_POINT('',(0.,-35.764258829506,-11.2768697064435));
#79284=CARTESIAN_POINT('',(11.,-36.0590497884573,-11.3395294590896));
#79285=CARTESIAN_POINT('',(22.,-35.764258829506,-11.2768697064435));
#79286=CARTESIAN_POINT('',(0.,-35.764258829506,-11.2768697064435));
#79287=CARTESIAN_POINT('',(22.,-40.2331784341656,-12.2267678919897));
#79288=CARTESIAN_POINT('Origin',(0.,-40.9563385449745,-9.52789761644378));
#79289=CARTESIAN_POINT('',(0.664285714285713,-40.9563385449745,-9.52789761644378));
#79290=CARTESIAN_POINT('',(0.,-40.9563385449745,-9.52789761644378));
#79291=CARTESIAN_POINT('Ctrl Pts',(0.664285714285713,-40.9563385449745,
-9.52789761644378));
#79292=CARTESIAN_POINT('Ctrl Pts',(0.614556259703007,-40.5947584895701,
-10.8773327542168));
#79293=CARTESIAN_POINT('Ctrl Pts',(0.664285714285713,-40.2331784341656,
-12.2267678919897));
#79294=CARTESIAN_POINT('Origin',(0.,-41.7451020134904,-5.05459769747091));
#79295=CARTESIAN_POINT('',(0.664285714285704,-41.7451020134904,-5.0545976974709));
#79296=CARTESIAN_POINT('',(0.,-41.7451020134904,-5.05459769747091));
#79297=CARTESIAN_POINT('',(6.93889390390723E-17,-41.1231689657038,-5.03287931686985));
#79298=CARTESIAN_POINT('Ctrl Pts',(0.664285714285704,-41.7451020134904,
-5.0545976974709));
#79299=CARTESIAN_POINT('Ctrl Pts',(0.329657625220838,-41.4318259656505,
-5.043657856817));
#79300=CARTESIAN_POINT('Ctrl Pts',(-6.93889390390723E-17,-41.1231689657038,
-5.03287931686985));
#79301=CARTESIAN_POINT('',(0.,-37.1791272503441,-4.89515034526194));
#79302=CARTESIAN_POINT('',(0.,-41.7451020134904,-5.05459769747091));
#79303=CARTESIAN_POINT('',(0.,-37.1791272503441,-4.89515034526194));
#79304=CARTESIAN_POINT('',(11.,-37.4803204240973,-4.90566824265506));
#79305=CARTESIAN_POINT('',(22.,-37.1791272503441,-4.89515034526194));
#79306=CARTESIAN_POINT('',(0.,-37.1791272503441,-4.89515034526194));
#79307=CARTESIAN_POINT('',(22.,-41.7451020134904,-5.05459769747091));
#79308=CARTESIAN_POINT('Origin',(0.,-41.9886217921762,-2.2711538903357));
#79309=CARTESIAN_POINT('',(0.6642857142857,-41.9886217921762,-2.2711538903357));
#79310=CARTESIAN_POINT('',(0.,-41.9886217921762,-2.2711538903357));
#79311=CARTESIAN_POINT('Ctrl Pts',(0.6642857142857,-41.9886217921762,-2.2711538903357));
#79312=CARTESIAN_POINT('Ctrl Pts',(0.614556259702998,-41.8668619028333,
-3.66287579390334));
#79313=CARTESIAN_POINT('Ctrl Pts',(0.664285714285704,-41.7451020134904,
-5.0545976974709));
#79314=CARTESIAN_POINT('Origin',(0.,-41.9886217921762,2.27115389033572));
#79315=CARTESIAN_POINT('',(0.66428571428571,-41.9886217921762,2.27115389033572));
#79316=CARTESIAN_POINT('',(0.,-41.9886217921762,2.27115389033572));
#79317=CARTESIAN_POINT('',(0.,-41.3723659476482,2.18454477955553));
#79318=CARTESIAN_POINT('Ctrl Pts',(0.66428571428571,-41.9886217921762,2.27115389033572));
#79319=CARTESIAN_POINT('Ctrl Pts',(0.329657628630436,-41.6782054311995,
2.22752771585878));
#79320=CARTESIAN_POINT('Ctrl Pts',(0.,-41.3723659476482,2.18454477955553));
#79321=CARTESIAN_POINT('',(0.,-37.4643267032267,1.63530568209484));
#79322=CARTESIAN_POINT('',(0.,-41.9886217921762,2.27115389033572));
#79323=CARTESIAN_POINT('',(0.,-37.4643267032267,1.63530568209484));
#79324=CARTESIAN_POINT('',(11.,-37.7627704896084,1.67724922094466));
#79325=CARTESIAN_POINT('',(22.,-37.4643267032267,1.63530568209484));
#79326=CARTESIAN_POINT('',(0.,-37.4643267032267,1.63530568209484));
#79327=CARTESIAN_POINT('',(22.,-41.9886217921762,2.27115389033572));
#79328=CARTESIAN_POINT('Origin',(0.,-41.7451020134904,5.05459769747093));
#79329=CARTESIAN_POINT('',(0.664285714285704,-41.7451020134904,5.05459769747093));
#79330=CARTESIAN_POINT('',(0.,-41.7451020134904,5.05459769747093));
#79331=CARTESIAN_POINT('Ctrl Pts',(0.664285714285704,-41.7451020134904,
5.05459769747093));
#79332=CARTESIAN_POINT('Ctrl Pts',(0.614556259703005,-41.8668619028333,
3.66287579390328));
#79333=CARTESIAN_POINT('Ctrl Pts',(0.66428571428571,-41.9886217921762,2.27115389033572));
#79334=CARTESIAN_POINT('Origin',(0.,-40.9563385449745,9.52789761644381));
#79335=CARTESIAN_POINT('',(0.664285714285704,-40.9563385449745,9.5278976164438));
#79336=CARTESIAN_POINT('',(0.,-40.9563385449745,9.52789761644381));
#79337=CARTESIAN_POINT('',(0.,-40.3644845257006,9.33559258828709));
#79338=CARTESIAN_POINT('Ctrl Pts',(0.664285714285704,-40.9563385449745,
9.5278976164438));
#79339=CARTESIAN_POINT('Ctrl Pts',(0.329657625908044,-40.6582137092941,
9.43103098539505));
#79340=CARTESIAN_POINT('Ctrl Pts',(-1.38777878078145E-16,-40.3644845257006,
9.33559258828709));
#79341=CARTESIAN_POINT('',(0.,-36.6111915470959,8.11607377380575));
#79342=CARTESIAN_POINT('',(0.,-40.9563385449745,9.52789761644381));
#79343=CARTESIAN_POINT('',(0.,-36.6111915470959,8.11607377380575));
#79344=CARTESIAN_POINT('',(11.,-36.8978178826767,8.20920431569502));
#79345=CARTESIAN_POINT('',(22.,-36.6111915470959,8.11607377380575));
#79346=CARTESIAN_POINT('',(0.,-36.6111915470959,8.11607377380575));
#79347=CARTESIAN_POINT('',(22.,-40.9563385449745,9.52789761644381));
#79348=CARTESIAN_POINT('Origin',(0.,-40.2331784341656,12.2267678919897));
#79349=CARTESIAN_POINT('',(0.664285714285703,-40.2331784341656,12.2267678919897));
#79350=CARTESIAN_POINT('',(0.,-40.2331784341656,12.2267678919897));
#79351=CARTESIAN_POINT('Ctrl Pts',(0.664285714285703,-40.2331784341656,
12.2267678919897));
#79352=CARTESIAN_POINT('Ctrl Pts',(0.614556259703,-40.5947584895701,10.8773327542167));
#79353=CARTESIAN_POINT('Ctrl Pts',(0.664285714285704,-40.9563385449745,
9.5278976164438));
#79354=CARTESIAN_POINT('Origin',(0.,-38.6796176759911,16.4951409948251));
#79355=CARTESIAN_POINT('',(0.664285714285705,-38.6796176759911,16.4951409948251));
#79356=CARTESIAN_POINT('',(0.,-38.6796176759911,16.4951409948251));
#79357=CARTESIAN_POINT('',(-1.38777878078145E-16,-38.1301486668543,16.2029831402613));
#79358=CARTESIAN_POINT('Ctrl Pts',(0.664285714285705,-38.6796176759911,
16.4951409948251));
#79359=CARTESIAN_POINT('Ctrl Pts',(0.329657624919205,-38.4028427395881,
16.3479771506921));
#79360=CARTESIAN_POINT('Ctrl Pts',(-6.93889390390723E-17,-38.1301486668543,
16.2029831402613));
#79361=CARTESIAN_POINT('',(0.,-34.6456438619633,14.3502390708311));
#79362=CARTESIAN_POINT('',(0.,-38.6796176759911,16.4951409948251));
#79363=CARTESIAN_POINT('',(0.,-34.6456438619633,14.3502390708311));
#79364=CARTESIAN_POINT('',(11.,-34.9117437505765,14.4917268913708));
#79365=CARTESIAN_POINT('',(22.,-34.6456438619633,14.3502390708311));
#79366=CARTESIAN_POINT('',(0.,-34.6456438619633,14.3502390708311));
#79367=CARTESIAN_POINT('',(22.,-38.6796176759911,16.4951409948251));
#79368=CARTESIAN_POINT('Origin',(0.,-37.4987900870893,19.0274339311535));
#79369=CARTESIAN_POINT('',(0.664285714285704,-37.4987900870893,19.0274339311535));
#79370=CARTESIAN_POINT('',(0.,-37.4987900870893,19.0274339311535));
#79371=CARTESIAN_POINT('Ctrl Pts',(0.664285714285704,-37.4987900870893,
19.0274339311535));
#79372=CARTESIAN_POINT('Ctrl Pts',(0.614556259702999,-38.0892038815402,
17.7612874629892));
#79373=CARTESIAN_POINT('Ctrl Pts',(0.664285714285705,-38.6796176759911,
16.4951409948251));
#79374=CARTESIAN_POINT('Origin',(0.,-35.2276361967536,22.9611878610227));
#79375=CARTESIAN_POINT('',(0.664285714285713,-35.2276361967536,22.9611878610227));
#79376=CARTESIAN_POINT('',(0.,-35.2276361967536,22.9611878610227));
#79377=CARTESIAN_POINT('',(4.16333634234434E-16,-34.7372475355518,22.5780542486238));
#79378=CARTESIAN_POINT('Ctrl Pts',(0.664285714285713,-35.2276361967536,
22.9611878610227));
#79379=CARTESIAN_POINT('Ctrl Pts',(0.329657622235105,-34.9806208249155,
22.7681983014793));
#79380=CARTESIAN_POINT('Ctrl Pts',(-6.93889390390723E-17,-34.7372475355518,
22.5780542486238));
#79381=CARTESIAN_POINT('',(0.,-31.6274058196267,20.1483796152605));
#79382=CARTESIAN_POINT('',(0.,-35.2276361967536,22.9611878610227));
#79383=CARTESIAN_POINT('',(0.,-31.6274058196267,20.1483796152605));
#79384=CARTESIAN_POINT('',(11.,-31.8648939508099,20.3339256786199));
#79385=CARTESIAN_POINT('',(22.,-31.6274058196267,20.1483796152605));
#79386=CARTESIAN_POINT('',(0.,-31.6274058196267,20.1483796152605));
#79387=CARTESIAN_POINT('',(22.,-35.2276361967536,22.9611878610227));
#79388=CARTESIAN_POINT('Origin',(0.,-33.6250199785202,25.2499610186654));
#79389=CARTESIAN_POINT('',(0.664285714285703,-33.6250199785202,25.2499610186654));
#79390=CARTESIAN_POINT('',(0.,-33.6250199785202,25.2499610186654));
#79391=CARTESIAN_POINT('Ctrl Pts',(0.664285714285703,-33.6250199785202,
25.2499610186654));
#79392=CARTESIAN_POINT('Ctrl Pts',(0.614556259703008,-34.4263280876369,
24.105574439844));
#79393=CARTESIAN_POINT('Ctrl Pts',(0.664285714285713,-35.2276361967536,
22.9611878610227));
#79394=CARTESIAN_POINT('Origin',(0.,-30.7052808177218,28.7295706529848));
#79395=CARTESIAN_POINT('',(0.664285714285712,-30.7052808177218,28.7295706529848));
#79396=CARTESIAN_POINT('',(0.,-30.7052808177218,28.7295706529848));
#79397=CARTESIAN_POINT('',(2.08166817117217E-16,-30.288872715777,28.2671026036886));
#79398=CARTESIAN_POINT('Ctrl Pts',(0.664285714285712,-30.7052808177218,
28.7295706529848));
#79399=CARTESIAN_POINT('Ctrl Pts',(0.329657619482983,-30.495530448021,28.496619267405));
#79400=CARTESIAN_POINT('Ctrl Pts',(6.93889390390723E-17,-30.288872715777,
28.2671026036886));
#79401=CARTESIAN_POINT('',(0.,-27.6481850557002,25.3343218406523));
#79402=CARTESIAN_POINT('',(0.,-30.7052808177218,28.7295706529848));
#79403=CARTESIAN_POINT('',(0.,-27.6481850557002,25.3343218406523));
#79404=CARTESIAN_POINT('',(11.,-27.8498454727622,25.5582884235871));
#79405=CARTESIAN_POINT('',(22.,-27.6481850557002,25.3343218406523));
#79406=CARTESIAN_POINT('',(0.,-27.6481850557002,25.3343218406523));
#79407=CARTESIAN_POINT('',(22.,-30.7052808177218,28.7295706529848));
#79408=CARTESIAN_POINT('Origin',(0.,-28.7295706529848,30.7052808177218));
#79409=CARTESIAN_POINT('',(0.664285714285709,-28.7295706529848,30.7052808177218));
#79410=CARTESIAN_POINT('',(0.,-28.7295706529848,30.7052808177218));
#79411=CARTESIAN_POINT('Ctrl Pts',(0.664285714285709,-28.7295706529848,
30.7052808177218));
#79412=CARTESIAN_POINT('Ctrl Pts',(0.614556259703005,-29.7174257353533,
29.7174257353533));
#79413=CARTESIAN_POINT('Ctrl Pts',(0.664285714285712,-30.7052808177218,
28.7295706529848));
#79414=CARTESIAN_POINT('Origin',(0.,-19.0274339311535,37.4987900870893));
#79415=CARTESIAN_POINT('',(0.664285714285711,-19.0274339311535,37.4987900870893));
#79416=CARTESIAN_POINT('',(0.,-19.0274339311535,37.4987900870893));
#79417=CARTESIAN_POINT('',(-1.38777878078145E-16,-18.7943116990243,36.9217923151073));
#79418=CARTESIAN_POINT('Ctrl Pts',(0.664285714285711,-19.0274339311535,
37.4987900870893));
#79419=CARTESIAN_POINT('Ctrl Pts',(0.329657619504279,-18.9100071228299,
37.2081485375689));
#79420=CARTESIAN_POINT('Ctrl Pts',(2.08166817117217E-16,-18.7943116990243,
36.9217923151073));
#79421=CARTESIAN_POINT('',(0.,-17.3159470879662,33.2627115017215));
#79422=CARTESIAN_POINT('',(0.,-19.0274339311535,37.4987900870893));
#79423=CARTESIAN_POINT('',(0.,-17.3159470879662,33.2627115017215));
#79424=CARTESIAN_POINT('',(11.,-17.4288448109885,33.5421431717545));
#79425=CARTESIAN_POINT('',(22.,-17.3159470879662,33.2627115017215));
#79426=CARTESIAN_POINT('',(0.,-17.3159470879662,33.2627115017215));
#79427=CARTESIAN_POINT('',(22.,-19.0274339311535,37.4987900870893));
#79428=CARTESIAN_POINT('Origin',(0.,-16.4951409948251,38.6796176759911));
#79429=CARTESIAN_POINT('',(0.66428571428571,-16.4951409948251,38.6796176759911));
#79430=CARTESIAN_POINT('',(0.,-16.4951409948251,38.6796176759911));
#79431=CARTESIAN_POINT('Ctrl Pts',(0.66428571428571,-16.4951409948251,38.6796176759911));
#79432=CARTESIAN_POINT('Ctrl Pts',(0.614556259703007,-17.7612874629893,
38.0892038815402));
#79433=CARTESIAN_POINT('Ctrl Pts',(0.664285714285711,-19.0274339311535,
37.4987900870893));
#79434=CARTESIAN_POINT('Origin',(0.,-12.2267678919897,40.2331784341656));
#79435=CARTESIAN_POINT('',(0.664285714285714,-12.2267678919897,40.2331784341656));
#79436=CARTESIAN_POINT('',(0.,-12.2267678919897,40.2331784341656));
#79437=CARTESIAN_POINT('',(0.,-12.0973819220119,39.6244653040641));
#79438=CARTESIAN_POINT('Ctrl Pts',(0.664285714285714,-12.2267678919897,
40.2331784341656));
#79439=CARTESIAN_POINT('Ctrl Pts',(0.329657619831027,-12.1615944362333,
39.9265614318751));
#79440=CARTESIAN_POINT('Ctrl Pts',(0.,-12.0973819220119,39.6244653040641));
#79441=CARTESIAN_POINT('',(0.,-11.2768697064435,35.764258829506));
#79442=CARTESIAN_POINT('',(0.,-12.2267678919897,40.2331784341656));
#79443=CARTESIAN_POINT('',(0.,-11.2768697064435,35.764258829506));
#79444=CARTESIAN_POINT('',(11.,-11.3395294590896,36.0590497884573));
#79445=CARTESIAN_POINT('',(22.,-11.2768697064435,35.764258829506));
#79446=CARTESIAN_POINT('',(0.,-11.2768697064435,35.764258829506));
#79447=CARTESIAN_POINT('',(22.,-12.2267678919897,40.2331784341656));
#79448=CARTESIAN_POINT('Origin',(0.,-9.52789761644379,40.9563385449745));
#79449=CARTESIAN_POINT('',(0.664285714285714,-9.52789761644379,40.9563385449745));
#79450=CARTESIAN_POINT('',(0.,-9.52789761644379,40.9563385449745));
#79451=CARTESIAN_POINT('Ctrl Pts',(0.664285714285714,-9.52789761644379,
40.9563385449745));
#79452=CARTESIAN_POINT('Ctrl Pts',(0.614556259703009,-10.8773327542168,
40.5947584895701));
#79453=CARTESIAN_POINT('Ctrl Pts',(0.664285714285714,-12.2267678919897,
40.2331784341656));
#79454=CARTESIAN_POINT('Origin',(0.,-5.05459769747091,41.7451020134904));
#79455=CARTESIAN_POINT('',(0.664285714285704,-5.05459769747091,41.7451020134904));
#79456=CARTESIAN_POINT('',(0.,-5.05459769747091,41.7451020134904));
#79457=CARTESIAN_POINT('',(6.93889390390723E-17,-5.03287931686985,41.1231689657038));
#79458=CARTESIAN_POINT('Ctrl Pts',(0.664285714285704,-5.05459769747091,
41.7451020134904));
#79459=CARTESIAN_POINT('Ctrl Pts',(0.329657625021025,-5.04365785681047,
41.4318259654634));
#79460=CARTESIAN_POINT('Ctrl Pts',(6.93889390390723E-17,-5.03287931686985,
41.1231689657038));
#79461=CARTESIAN_POINT('',(0.,-4.89515034526194,37.1791272503441));
#79462=CARTESIAN_POINT('',(0.,-5.05459769747091,41.7451020134904));
#79463=CARTESIAN_POINT('',(0.,-4.89515034526194,37.1791272503441));
#79464=CARTESIAN_POINT('',(11.,-4.90566824265506,37.4803204240973));
#79465=CARTESIAN_POINT('',(22.,-4.89515034526194,37.1791272503441));
#79466=CARTESIAN_POINT('',(0.,-4.89515034526194,37.1791272503441));
#79467=CARTESIAN_POINT('',(22.,-5.05459769747091,41.7451020134904));
#79468=CARTESIAN_POINT('Origin',(0.,-2.2711538903357,41.9886217921762));
#79469=CARTESIAN_POINT('',(0.6642857142857,-2.2711538903357,41.9886217921762));
#79470=CARTESIAN_POINT('',(0.,-2.2711538903357,41.9886217921762));
#79471=CARTESIAN_POINT('Ctrl Pts',(0.6642857142857,-2.2711538903357,41.9886217921762));
#79472=CARTESIAN_POINT('Ctrl Pts',(0.614556259702998,-3.66287579390335,
41.8668619028333));
#79473=CARTESIAN_POINT('Ctrl Pts',(0.664285714285704,-5.05459769747091,
41.7451020134904));
#79474=CARTESIAN_POINT('Origin',(0.,2.27115389033571,41.9886217921762));
#79475=CARTESIAN_POINT('',(0.66428571428571,2.27115389033571,41.9886217921762));
#79476=CARTESIAN_POINT('',(0.,2.27115389033571,41.9886217921762));
#79477=CARTESIAN_POINT('',(-6.93889390390723E-17,2.18454477955552,41.3723659476482));
#79478=CARTESIAN_POINT('Ctrl Pts',(0.66428571428571,2.27115389033571,41.9886217921762));
#79479=CARTESIAN_POINT('Ctrl Pts',(0.329657622668474,2.22752771508157,41.6782054256694));
#79480=CARTESIAN_POINT('Ctrl Pts',(-6.93889390390723E-17,2.18454477955552,
41.3723659476482));
#79481=CARTESIAN_POINT('',(0.,1.63530568209483,37.4643267032268));
#79482=CARTESIAN_POINT('',(0.,2.27115389033571,41.9886217921762));
#79483=CARTESIAN_POINT('',(0.,1.63530568209483,37.4643267032268));
#79484=CARTESIAN_POINT('',(11.,1.67724922094465,37.7627704896084));
#79485=CARTESIAN_POINT('',(22.,1.63530568209483,37.4643267032268));
#79486=CARTESIAN_POINT('',(0.,1.63530568209483,37.4643267032268));
#79487=CARTESIAN_POINT('',(22.,2.27115389033571,41.9886217921762));
#79488=CARTESIAN_POINT('Origin',(0.,5.05459769747092,41.7451020134904));
#79489=CARTESIAN_POINT('',(0.664285714285704,5.05459769747092,41.7451020134904));
#79490=CARTESIAN_POINT('',(0.,5.05459769747092,41.7451020134904));
#79491=CARTESIAN_POINT('Ctrl Pts',(0.664285714285704,5.05459769747092,41.7451020134904));
#79492=CARTESIAN_POINT('Ctrl Pts',(0.614556259703005,3.66287579390327,41.8668619028333));
#79493=CARTESIAN_POINT('Ctrl Pts',(0.66428571428571,2.27115389033571,41.9886217921762));
#79494=CARTESIAN_POINT('Origin',(0.,9.5278976164438,40.9563385449745));
#79495=CARTESIAN_POINT('',(0.664285714285704,9.5278976164438,40.9563385449745));
#79496=CARTESIAN_POINT('',(0.,9.5278976164438,40.9563385449745));
#79497=CARTESIAN_POINT('',(0.,9.33559258828709,40.3644845257006));
#79498=CARTESIAN_POINT('Ctrl Pts',(0.664285714285704,9.5278976164438,40.9563385449745));
#79499=CARTESIAN_POINT('Ctrl Pts',(0.329657623132566,9.43103098459169,40.6582137068217));
#79500=CARTESIAN_POINT('Ctrl Pts',(-6.93889390390723E-17,9.33559258828709,
40.3644845257006));
#79501=CARTESIAN_POINT('',(0.,8.11607377380574,36.6111915470959));
#79502=CARTESIAN_POINT('',(0.,9.5278976164438,40.9563385449745));
#79503=CARTESIAN_POINT('',(0.,8.11607377380574,36.6111915470959));
#79504=CARTESIAN_POINT('',(11.,8.20920431569501,36.8978178826767));
#79505=CARTESIAN_POINT('',(22.,8.11607377380574,36.6111915470959));
#79506=CARTESIAN_POINT('',(0.,8.11607377380574,36.6111915470959));
#79507=CARTESIAN_POINT('',(22.,9.5278976164438,40.9563385449745));
#79508=CARTESIAN_POINT('Origin',(0.,12.2267678919897,40.2331784341656));
#79509=CARTESIAN_POINT('',(0.664285714285704,12.2267678919897,40.2331784341656));
#79510=CARTESIAN_POINT('',(0.,12.2267678919897,40.2331784341656));
#79511=CARTESIAN_POINT('Ctrl Pts',(0.664285714285704,12.2267678919897,40.2331784341656));
#79512=CARTESIAN_POINT('Ctrl Pts',(0.614556259702999,10.8773327542167,40.5947584895701));
#79513=CARTESIAN_POINT('Ctrl Pts',(0.664285714285704,9.5278976164438,40.9563385449745));
#79514=CARTESIAN_POINT('Origin',(0.,16.4951409948251,38.6796176759911));
#79515=CARTESIAN_POINT('',(0.66428571428571,16.4951409948251,38.6796176759911));
#79516=CARTESIAN_POINT('',(0.,16.4951409948251,38.6796176759911));
#79517=CARTESIAN_POINT('',(6.93889390390723E-17,16.2029831402613,38.1301486668542));
#79518=CARTESIAN_POINT('Ctrl Pts',(0.66428571428571,16.4951409948251,38.6796176759911));
#79519=CARTESIAN_POINT('Ctrl Pts',(0.329657621910239,16.3479771493689,38.4028427370996));
#79520=CARTESIAN_POINT('Ctrl Pts',(0.,16.2029831402613,38.1301486668543));
#79521=CARTESIAN_POINT('',(0.,14.3502390708311,34.6456438619633));
#79522=CARTESIAN_POINT('',(0.,16.4951409948251,38.6796176759911));
#79523=CARTESIAN_POINT('',(0.,14.3502390708311,34.6456438619633));
#79524=CARTESIAN_POINT('',(11.,14.4917268913708,34.9117437505765));
#79525=CARTESIAN_POINT('',(22.,14.3502390708311,34.6456438619633));
#79526=CARTESIAN_POINT('',(0.,14.3502390708311,34.6456438619633));
#79527=CARTESIAN_POINT('',(22.,16.4951409948251,38.6796176759911));
#79528=CARTESIAN_POINT('Origin',(0.,19.0274339311535,37.4987900870893));
#79529=CARTESIAN_POINT('',(0.664285714285716,19.0274339311535,37.4987900870893));
#79530=CARTESIAN_POINT('',(0.,19.0274339311535,37.4987900870893));
#79531=CARTESIAN_POINT('Ctrl Pts',(0.664285714285716,19.0274339311535,37.4987900870893));
#79532=CARTESIAN_POINT('Ctrl Pts',(0.614556259703006,17.7612874629893,38.0892038815402));
#79533=CARTESIAN_POINT('Ctrl Pts',(0.66428571428571,16.4951409948251,38.6796176759911));
#79534=CARTESIAN_POINT('Origin',(0.,22.9611878610227,35.2276361967536));
#79535=CARTESIAN_POINT('',(0.664285714285716,22.9611878610227,35.2276361967536));
#79536=CARTESIAN_POINT('',(0.,22.9611878610227,35.2276361967536));
#79537=CARTESIAN_POINT('',(-2.77555756156289E-16,22.5780542486238,34.7372475355518));
#79538=CARTESIAN_POINT('Ctrl Pts',(0.664285714285716,22.9611878610227,35.2276361967536));
#79539=CARTESIAN_POINT('Ctrl Pts',(0.329657619188245,22.7681982997223,34.9806208226665));
#79540=CARTESIAN_POINT('Ctrl Pts',(-2.77555756156289E-16,22.5780542486238,
34.7372475355518));
#79541=CARTESIAN_POINT('',(0.,20.1483796152605,31.6274058196267));
#79542=CARTESIAN_POINT('',(0.,22.9611878610227,35.2276361967536));
#79543=CARTESIAN_POINT('',(0.,20.1483796152605,31.6274058196267));
#79544=CARTESIAN_POINT('',(11.,20.3339256786199,31.8648939508099));
#79545=CARTESIAN_POINT('',(22.,20.1483796152605,31.6274058196267));
#79546=CARTESIAN_POINT('',(0.,20.1483796152605,31.6274058196267));
#79547=CARTESIAN_POINT('',(22.,22.9611878610227,35.2276361967536));
#79548=CARTESIAN_POINT('Origin',(0.,25.2499610186653,33.6250199785202));
#79549=CARTESIAN_POINT('',(0.664285714285713,25.2499610186653,33.6250199785202));
#79550=CARTESIAN_POINT('',(0.,25.2499610186653,33.6250199785202));
#79551=CARTESIAN_POINT('Ctrl Pts',(0.664285714285713,25.2499610186653,33.6250199785202));
#79552=CARTESIAN_POINT('Ctrl Pts',(0.614556259703012,24.105574439844,34.4263280876369));
#79553=CARTESIAN_POINT('Ctrl Pts',(0.664285714285716,22.9611878610227,35.2276361967536));
#79554=CARTESIAN_POINT('Origin',(0.,28.7295706529848,30.7052808177218));
#79555=CARTESIAN_POINT('',(0.664285714285715,28.7295706529848,30.7052808177218));
#79556=CARTESIAN_POINT('',(0.,28.7295706529848,30.7052808177218));
#79557=CARTESIAN_POINT('',(0.,28.2671026036886,30.288872715777));
#79558=CARTESIAN_POINT('Ctrl Pts',(0.664285714285715,28.7295706529848,30.7052808177218));
#79559=CARTESIAN_POINT('Ctrl Pts',(0.329657620568989,28.4966192681609,30.4955304487016));
#79560=CARTESIAN_POINT('Ctrl Pts',(-2.77555756156289E-16,28.2671026036886,
30.288872715777));
#79561=CARTESIAN_POINT('',(0.,25.3343218406523,27.6481850557002));
#79562=CARTESIAN_POINT('',(0.,28.7295706529848,30.7052808177218));
#79563=CARTESIAN_POINT('',(0.,25.3343218406523,27.6481850557002));
#79564=CARTESIAN_POINT('',(11.,25.5582884235871,27.8498454727622));
#79565=CARTESIAN_POINT('',(22.,25.3343218406523,27.6481850557002));
#79566=CARTESIAN_POINT('',(0.,25.3343218406523,27.6481850557002));
#79567=CARTESIAN_POINT('',(22.,28.7295706529848,30.7052808177218));
#79568=CARTESIAN_POINT('Origin',(0.,30.7052808177218,28.7295706529848));
#79569=CARTESIAN_POINT('',(0.664285714285712,30.7052808177218,28.7295706529848));
#79570=CARTESIAN_POINT('',(0.,30.7052808177218,28.7295706529848));
#79571=CARTESIAN_POINT('Ctrl Pts',(0.664285714285712,30.7052808177218,28.7295706529848));
#79572=CARTESIAN_POINT('Ctrl Pts',(0.614556259703008,29.7174257353533,29.7174257353533));
#79573=CARTESIAN_POINT('Ctrl Pts',(0.664285714285715,28.7295706529848,30.7052808177218));
#79574=CARTESIAN_POINT('Origin',(0.,33.6250199785202,25.2499610186653));
#79575=CARTESIAN_POINT('',(0.664285714285709,33.6250199785202,25.2499610186653));
#79576=CARTESIAN_POINT('',(0.,33.6250199785202,25.2499610186653));
#79577=CARTESIAN_POINT('',(1.38777878078145E-16,33.0972693499844,24.9201858254425));
#79578=CARTESIAN_POINT('Ctrl Pts',(0.664285714285709,33.6250199785202,25.2499610186653));
#79579=CARTESIAN_POINT('Ctrl Pts',(0.329657623920708,33.3591848819878,25.0838488141804));
#79580=CARTESIAN_POINT('Ctrl Pts',(4.16333634234434E-16,33.0972693499844,
24.9201858254425));
#79581=CARTESIAN_POINT('',(0.,29.7504935167013,22.8288881795131));
#79582=CARTESIAN_POINT('',(0.,33.6250199785202,25.2499610186653));
#79583=CARTESIAN_POINT('',(0.,29.7504935167013,22.8288881795131));
#79584=CARTESIAN_POINT('',(11.,30.0060755079215,22.9885935327265));
#79585=CARTESIAN_POINT('',(22.,29.7504935167013,22.8288881795131));
#79586=CARTESIAN_POINT('',(0.,29.7504935167013,22.8288881795131));
#79587=CARTESIAN_POINT('',(22.,33.6250199785202,25.2499610186653));
#79588=CARTESIAN_POINT('Origin',(0.,35.2276361967536,22.9611878610227));
#79589=CARTESIAN_POINT('',(0.664285714285705,35.2276361967536,22.9611878610227));
#79590=CARTESIAN_POINT('',(0.,35.2276361967536,22.9611878610227));
#79591=CARTESIAN_POINT('Ctrl Pts',(0.664285714285705,35.2276361967536,22.9611878610227));
#79592=CARTESIAN_POINT('Ctrl Pts',(0.614556259703003,34.4263280876369,24.105574439844));
#79593=CARTESIAN_POINT('Ctrl Pts',(0.664285714285709,33.6250199785202,25.2499610186653));
#79594=CARTESIAN_POINT('Origin',(0.,37.4987900870893,19.0274339311535));
#79595=CARTESIAN_POINT('',(0.664285714285711,37.4987900870893,19.0274339311535));
#79596=CARTESIAN_POINT('',(0.,37.4987900870893,19.0274339311535));
#79597=CARTESIAN_POINT('',(-1.38777878078145E-16,36.9217923151073,18.7943116990243));
#79598=CARTESIAN_POINT('Ctrl Pts',(0.664285714285711,37.4987900870893,19.0274339311535));
#79599=CARTESIAN_POINT('Ctrl Pts',(0.329657629073952,37.2081485458799,18.9100071261878));
#79600=CARTESIAN_POINT('Ctrl Pts',(2.08166817117217E-16,36.9217923151073,
18.7943116990243));
#79601=CARTESIAN_POINT('',(0.,33.2627115017215,17.3159470879662));
#79602=CARTESIAN_POINT('',(0.,37.4987900870893,19.0274339311535));
#79603=CARTESIAN_POINT('',(0.,33.2627115017215,17.3159470879662));
#79604=CARTESIAN_POINT('',(11.,33.5421431717545,17.4288448109885));
#79605=CARTESIAN_POINT('',(22.,33.2627115017215,17.3159470879662));
#79606=CARTESIAN_POINT('',(0.,33.2627115017215,17.3159470879662));
#79607=CARTESIAN_POINT('',(22.,37.4987900870893,19.0274339311535));
#79608=CARTESIAN_POINT('Origin',(0.,38.6796176759911,16.4951409948251));
#79609=CARTESIAN_POINT('',(0.66428571428571,38.6796176759911,16.4951409948251));
#79610=CARTESIAN_POINT('',(0.,38.6796176759911,16.4951409948251));
#79611=CARTESIAN_POINT('Ctrl Pts',(0.66428571428571,38.6796176759911,16.4951409948251));
#79612=CARTESIAN_POINT('Ctrl Pts',(0.614556259703007,38.0892038815402,17.7612874629893));
#79613=CARTESIAN_POINT('Ctrl Pts',(0.664285714285711,37.4987900870893,19.0274339311535));
#79614=CARTESIAN_POINT('Origin',(0.,40.2331784341656,12.2267678919897));
#79615=CARTESIAN_POINT('',(0.664285714285714,40.2331784341656,12.2267678919897));
#79616=CARTESIAN_POINT('',(0.,40.2331784341656,12.2267678919897));
#79617=CARTESIAN_POINT('',(0.,39.6244653040641,12.0973819220119));
#79618=CARTESIAN_POINT('Ctrl Pts',(0.664285714285714,40.2331784341656,12.2267678919897));
#79619=CARTESIAN_POINT('Ctrl Pts',(0.329657622780289,39.9265614345773,12.1615944368077));
#79620=CARTESIAN_POINT('Ctrl Pts',(-6.93889390390723E-17,39.6244653040641,
12.0973819220119));
#79621=CARTESIAN_POINT('',(0.,35.764258829506,11.2768697064435));
#79622=CARTESIAN_POINT('',(0.,40.2331784341656,12.2267678919897));
#79623=CARTESIAN_POINT('',(0.,35.764258829506,11.2768697064435));
#79624=CARTESIAN_POINT('',(11.,36.0590497884573,11.3395294590896));
#79625=CARTESIAN_POINT('',(22.,35.764258829506,11.2768697064435));
#79626=CARTESIAN_POINT('',(0.,35.764258829506,11.2768697064435));
#79627=CARTESIAN_POINT('',(22.,40.2331784341656,12.2267678919897));
#79628=CARTESIAN_POINT('Origin',(0.,40.9563385449745,9.5278976164438));
#79629=CARTESIAN_POINT('',(0.664285714285714,40.9563385449745,9.52789761644379));
#79630=CARTESIAN_POINT('',(0.,40.9563385449745,9.5278976164438));
#79631=CARTESIAN_POINT('Ctrl Pts',(0.664285714285714,40.9563385449745,9.52789761644379));
#79632=CARTESIAN_POINT('Ctrl Pts',(0.614556259703009,40.5947584895701,10.8773327542168));
#79633=CARTESIAN_POINT('Ctrl Pts',(0.664285714285714,40.2331784341656,12.2267678919897));
#79634=CARTESIAN_POINT('Origin',(0.45,0.,0.));
#79635=CARTESIAN_POINT('',(0.,40.3644845257006,9.33559258828708));
#79636=CARTESIAN_POINT('Ctrl Pts',(6.93889390390723E-17,40.3644845257006,
9.33559258828708));
#79637=CARTESIAN_POINT('Ctrl Pts',(0.32965762598791,40.6582137093653,9.43103098541816));
#79638=CARTESIAN_POINT('Ctrl Pts',(0.664285714285714,40.9563385449745,9.52789761644379));
#79639=CARTESIAN_POINT('Origin',(0.,0.,0.));
#79640=CARTESIAN_POINT('Origin',(0.45,0.,0.));
#79641=CARTESIAN_POINT('',(0.,38.1301486668543,16.2029831402613));
#79642=CARTESIAN_POINT('Ctrl Pts',(-2.08166817117217E-16,38.1301486668543,
16.2029831402613));
#79643=CARTESIAN_POINT('Ctrl Pts',(0.32965762185849,38.4028427370567,16.3479771493462));
#79644=CARTESIAN_POINT('Ctrl Pts',(0.66428571428571,38.6796176759911,16.4951409948251));
#79645=CARTESIAN_POINT('Origin',(0.,0.,0.));
#79646=CARTESIAN_POINT('Origin',(0.45,0.,0.));
#79647=CARTESIAN_POINT('',(-3.46944695195361E-16,34.7372475355518,22.5780542486238));
#79648=CARTESIAN_POINT('Ctrl Pts',(-3.46944695195361E-16,34.7372475355518,
22.5780542486238));
#79649=CARTESIAN_POINT('Ctrl Pts',(0.329657620646495,34.9806208237429,22.7681983005632));
#79650=CARTESIAN_POINT('Ctrl Pts',(0.664285714285705,35.2276361967536,22.9611878610227));
#79651=CARTESIAN_POINT('Origin',(0.,0.,0.));
#79652=CARTESIAN_POINT('Origin',(0.45,0.,0.));
#79653=CARTESIAN_POINT('',(5.55111512312578E-16,30.288872715777,28.2671026036886));
#79654=CARTESIAN_POINT('Ctrl Pts',(6.93889390390723E-17,30.288872715777,
28.2671026036886));
#79655=CARTESIAN_POINT('Ctrl Pts',(0.329657619423762,30.4955304479838,28.4966192673637));
#79656=CARTESIAN_POINT('Ctrl Pts',(0.664285714285712,30.7052808177218,28.7295706529848));
#79657=CARTESIAN_POINT('Origin',(0.,0.,0.));
#79658=CARTESIAN_POINT('Origin',(0.45,0.,0.));
#79659=CARTESIAN_POINT('',(0.,24.9201858254425,33.0972693499844));
#79660=CARTESIAN_POINT('Ctrl Pts',(2.08166817117217E-16,24.9201858254425,
33.0972693499844));
#79661=CARTESIAN_POINT('Ctrl Pts',(0.329657620988788,25.0838488127251,33.3591848796588));
#79662=CARTESIAN_POINT('Ctrl Pts',(0.664285714285713,25.2499610186653,33.6250199785202));
#79663=CARTESIAN_POINT('Origin',(0.,0.,0.));
#79664=CARTESIAN_POINT('Origin',(0.45,0.,0.));
#79665=CARTESIAN_POINT('',(1.38777878078145E-16,18.7943116990243,36.9217923151073));
#79666=CARTESIAN_POINT('Ctrl Pts',(-6.93889390390723E-17,18.7943116990243,
36.9217923151073));
#79667=CARTESIAN_POINT('Ctrl Pts',(0.329657618925708,18.9100071226269,37.2081485370664));
#79668=CARTESIAN_POINT('Ctrl Pts',(0.664285714285716,19.0274339311535,37.4987900870893));
#79669=CARTESIAN_POINT('Origin',(0.,0.,0.));
#79670=CARTESIAN_POINT('Origin',(0.45,0.,0.));
#79671=CARTESIAN_POINT('',(6.93889390390723E-17,12.097381922012,39.6244653040641));
#79672=CARTESIAN_POINT('Ctrl Pts',(1.38777878078145E-16,12.097381922012,
39.6244653040641));
#79673=CARTESIAN_POINT('Ctrl Pts',(0.329657622650879,12.1615944367825,39.9265614344587));
#79674=CARTESIAN_POINT('Ctrl Pts',(0.664285714285704,12.2267678919897,40.2331784341656));
#79675=CARTESIAN_POINT('Origin',(0.,0.,0.));
#79676=CARTESIAN_POINT('Origin',(0.45,0.,0.));
#79677=CARTESIAN_POINT('',(6.93889390390723E-17,5.03287931686986,41.1231689657038));
#79678=CARTESIAN_POINT('Ctrl Pts',(0.,5.03287931686986,41.1231689657038));
#79679=CARTESIAN_POINT('Ctrl Pts',(0.329657625188712,5.04365785681596,41.4318259656204));
#79680=CARTESIAN_POINT('Ctrl Pts',(0.664285714285704,5.05459769747092,41.7451020134904));
#79681=CARTESIAN_POINT('Origin',(0.,0.,0.));
#79682=CARTESIAN_POINT('Origin',(0.45,0.,0.));
#79683=CARTESIAN_POINT('',(-6.93889390390723E-17,-2.18454477955551,41.3723659476482));
#79684=CARTESIAN_POINT('Ctrl Pts',(0.,-2.18454477955551,41.3723659476482));
#79685=CARTESIAN_POINT('Ctrl Pts',(0.32965762278925,-2.2275277150973,41.6782054257814));
#79686=CARTESIAN_POINT('Ctrl Pts',(0.6642857142857,-2.2711538903357,41.9886217921762));
#79687=CARTESIAN_POINT('Origin',(0.,0.,0.));
#79688=CARTESIAN_POINT('Origin',(0.45,0.,0.));
#79689=CARTESIAN_POINT('',(1.38777878078145E-16,-9.33559258828708,40.3644845257006));
#79690=CARTESIAN_POINT('Ctrl Pts',(0.,-9.33559258828708,40.3644845257006));
#79691=CARTESIAN_POINT('Ctrl Pts',(0.329657625964886,-9.43103098541149,
40.6582137093448));
#79692=CARTESIAN_POINT('Ctrl Pts',(0.664285714285714,-9.52789761644379,
40.9563385449745));
#79693=CARTESIAN_POINT('Origin',(0.,0.,0.));
#79694=CARTESIAN_POINT('Origin',(0.45,0.,0.));
#79695=CARTESIAN_POINT('',(0.,-16.2029831402613,38.1301486668543));
#79696=CARTESIAN_POINT('Ctrl Pts',(-1.38777878078145E-16,-16.2029831402613,
38.1301486668543));
#79697=CARTESIAN_POINT('Ctrl Pts',(0.329657621211232,-16.3479771490615,
38.4028427365214));
#79698=CARTESIAN_POINT('Ctrl Pts',(0.66428571428571,-16.4951409948251,38.6796176759911));
#79699=CARTESIAN_POINT('Origin',(0.,0.,0.));
#79700=CARTESIAN_POINT('Origin',(0.45,0.,0.));
#79701=CARTESIAN_POINT('',(3.46944695195361E-16,-28.2671026036886,30.288872715777));
#79702=CARTESIAN_POINT('Ctrl Pts',(1.38777878078145E-16,-28.2671026036886,
30.288872715777));
#79703=CARTESIAN_POINT('Ctrl Pts',(0.329657622690223,-28.4966192696375,
30.4955304500311));
#79704=CARTESIAN_POINT('Ctrl Pts',(0.664285714285709,-28.7295706529848,
30.7052808177218));
#79705=CARTESIAN_POINT('Origin',(0.,0.,0.));
#79706=CARTESIAN_POINT('Origin',(0.45,0.,0.));
#79707=CARTESIAN_POINT('',(6.93889390390723E-17,-33.0972693499844,24.9201858254425));
#79708=CARTESIAN_POINT('Ctrl Pts',(4.16333634234434E-16,-33.0972693499844,
24.9201858254425));
#79709=CARTESIAN_POINT('Ctrl Pts',(0.329657624090997,-33.3591848821231,
25.0838488142649));
#79710=CARTESIAN_POINT('Ctrl Pts',(0.664285714285703,-33.6250199785202,
25.2499610186654));
#79711=CARTESIAN_POINT('Origin',(0.,0.,0.));
#79712=CARTESIAN_POINT('Origin',(0.45,0.,0.));
#79713=CARTESIAN_POINT('',(-1.38777878078145E-16,-36.9217923151073,18.7943116990243));
#79714=CARTESIAN_POINT('Ctrl Pts',(1.38777878078145E-16,-36.9217923151073,
18.7943116990243));
#79715=CARTESIAN_POINT('Ctrl Pts',(0.329657619578977,-37.2081485376338,
18.9100071228561));
#79716=CARTESIAN_POINT('Ctrl Pts',(0.664285714285704,-37.4987900870893,
19.0274339311535));
#79717=CARTESIAN_POINT('Origin',(0.,0.,0.));
#79718=CARTESIAN_POINT('Origin',(0.45,0.,0.));
#79719=CARTESIAN_POINT('',(0.,-39.6244653040641,12.097381922012));
#79720=CARTESIAN_POINT('Ctrl Pts',(0.,-39.6244653040641,12.097381922012));
#79721=CARTESIAN_POINT('Ctrl Pts',(0.329657619736489,-39.9265614317885,
12.1615944362149));
#79722=CARTESIAN_POINT('Ctrl Pts',(0.664285714285703,-40.2331784341656,
12.2267678919897));
#79723=CARTESIAN_POINT('Origin',(0.,0.,0.));
#79724=CARTESIAN_POINT('Origin',(0.45,0.,0.));
#79725=CARTESIAN_POINT('',(-6.93889390390723E-17,-41.1231689657038,5.03287931686987));
#79726=CARTESIAN_POINT('Ctrl Pts',(0.,-41.1231689657038,5.03287931686987));
#79727=CARTESIAN_POINT('Ctrl Pts',(0.329657625064268,-41.4318259655039,
5.0436578568119));
#79728=CARTESIAN_POINT('Ctrl Pts',(0.664285714285704,-41.7451020134904,
5.05459769747093));
#79729=CARTESIAN_POINT('Origin',(0.,0.,0.));
#79730=CARTESIAN_POINT('Origin',(0.45,0.,0.));
#79731=CARTESIAN_POINT('',(-6.93889390390723E-17,-41.3723659476482,-2.18454477955551));
#79732=CARTESIAN_POINT('Ctrl Pts',(6.93889390390723E-17,-41.3723659476482,
-2.18454477955551));
#79733=CARTESIAN_POINT('Ctrl Pts',(0.329657625843401,-41.6782054286144,
-2.22752771549544));
#79734=CARTESIAN_POINT('Ctrl Pts',(0.6642857142857,-41.9886217921762,-2.2711538903357));
#79735=CARTESIAN_POINT('Origin',(0.,0.,0.));
#79736=CARTESIAN_POINT('Origin',(0.45,0.,0.));
#79737=CARTESIAN_POINT('',(1.38777878078145E-16,-40.3644845257006,-9.33559258828707));
#79738=CARTESIAN_POINT('Ctrl Pts',(2.77555756156289E-16,-40.3644845257006,
-9.33559258828707));
#79739=CARTESIAN_POINT('Ctrl Pts',(0.329657625997959,-40.6582137093743,
-9.43103098542106));
#79740=CARTESIAN_POINT('Ctrl Pts',(0.664285714285713,-40.9563385449745,
-9.52789761644378));
#79741=CARTESIAN_POINT('Origin',(0.,0.,0.));
#79742=CARTESIAN_POINT('Origin',(0.45,0.,0.));
#79743=CARTESIAN_POINT('',(-2.08166817117217E-16,-38.1301486668543,-16.2029831402613));
#79744=CARTESIAN_POINT('Ctrl Pts',(1.38777878078145E-16,-38.1301486668543,
-16.2029831402613));
#79745=CARTESIAN_POINT('Ctrl Pts',(0.329657621863082,-38.4028427370606,
-16.3479771493482));
#79746=CARTESIAN_POINT('Ctrl Pts',(0.664285714285701,-38.6796176759911,
-16.4951409948251));
#79747=CARTESIAN_POINT('Origin',(0.,0.,0.));
#79748=CARTESIAN_POINT('Origin',(0.45,0.,0.));
#79749=CARTESIAN_POINT('',(-2.08166817117217E-16,-34.7372475355518,-22.5780542486238));
#79750=CARTESIAN_POINT('Ctrl Pts',(-4.16333634234434E-16,-34.7372475355518,
-22.5780542486238));
#79751=CARTESIAN_POINT('Ctrl Pts',(0.329657621436075,-34.9806208243257,
-22.7681983010185));
#79752=CARTESIAN_POINT('Ctrl Pts',(0.664285714285711,-35.2276361967536,
-22.9611878610227));
#79753=CARTESIAN_POINT('Origin',(0.,0.,0.));
#79754=CARTESIAN_POINT('Origin',(0.45,0.,0.));
#79755=CARTESIAN_POINT('',(5.55111512312578E-16,-30.288872715777,-28.2671026036886));
#79756=CARTESIAN_POINT('Ctrl Pts',(6.93889390390723E-17,-30.288872715777,
-28.2671026036886));
#79757=CARTESIAN_POINT('Ctrl Pts',(0.329657619423762,-30.4955304479838,
-28.4966192673637));
#79758=CARTESIAN_POINT('Ctrl Pts',(0.664285714285712,-30.7052808177218,
-28.7295706529848));
#79759=CARTESIAN_POINT('Origin',(0.,0.,0.));
#79760=CARTESIAN_POINT('Origin',(0.45,0.,0.));
#79761=CARTESIAN_POINT('',(0.,-24.9201858254425,-33.0972693499844));
#79762=CARTESIAN_POINT('Ctrl Pts',(2.77555756156289E-16,-24.9201858254425,
-33.0972693499844));
#79763=CARTESIAN_POINT('Ctrl Pts',(0.329657623996619,-25.0838488142181,
-33.3591848820481));
#79764=CARTESIAN_POINT('Ctrl Pts',(0.664285714285703,-25.2499610186654,
-33.6250199785202));
#79765=CARTESIAN_POINT('Origin',(0.,0.,0.));
#79766=CARTESIAN_POINT('Origin',(0.45,0.,0.));
#79767=CARTESIAN_POINT('',(-6.93889390390723E-17,-12.097381922012,-39.6244653040641));
#79768=CARTESIAN_POINT('Ctrl Pts',(-6.93889390390723E-17,-12.097381922012,
-39.6244653040641));
#79769=CARTESIAN_POINT('Ctrl Pts',(0.329657619756358,-12.1615944362188,
-39.9265614318067));
#79770=CARTESIAN_POINT('Ctrl Pts',(0.664285714285714,-12.2267678919898,
-40.2331784341656));
#79771=CARTESIAN_POINT('Origin',(0.,0.,0.));
#79772=CARTESIAN_POINT('Origin',(0.45,0.,0.));
#79773=CARTESIAN_POINT('',(-6.93889390390723E-17,-5.03287931686986,-41.1231689657038));
#79774=CARTESIAN_POINT('Ctrl Pts',(0.,-5.03287931686986,-41.1231689657038));
#79775=CARTESIAN_POINT('Ctrl Pts',(0.329657619114913,-5.04365785661741,
-41.4318259599347));
#79776=CARTESIAN_POINT('Ctrl Pts',(0.664285714285704,-5.05459769747091,
-41.7451020134904));
#79777=CARTESIAN_POINT('Origin',(0.,0.,0.));
#79778=CARTESIAN_POINT('Origin',(0.45,0.,0.));
#79779=CARTESIAN_POINT('',(0.,2.1845447795555,-41.3723659476482));
#79780=CARTESIAN_POINT('Ctrl Pts',(6.93889390390723E-17,2.1845447795555,
-41.3723659476482));
#79781=CARTESIAN_POINT('Ctrl Pts',(0.32965762590867,2.22752771550395,-41.6782054286749));
#79782=CARTESIAN_POINT('Ctrl Pts',(0.6642857142857,2.2711538903357,-41.9886217921762));
#79783=CARTESIAN_POINT('Origin',(0.,0.,0.));
#79784=CARTESIAN_POINT('Origin',(0.45,0.,0.));
#79785=CARTESIAN_POINT('',(2.77555756156289E-16,9.33559258828707,-40.3644845257006));
#79786=CARTESIAN_POINT('Ctrl Pts',(2.77555756156289E-16,9.33559258828707,
-40.3644845257006));
#79787=CARTESIAN_POINT('Ctrl Pts',(0.329657625970749,9.43103098541318,-40.65821370935));
#79788=CARTESIAN_POINT('Ctrl Pts',(0.664285714285714,9.52789761644378,-40.9563385449745));
#79789=CARTESIAN_POINT('Origin',(0.,0.,0.));
#79790=CARTESIAN_POINT('Origin',(0.45,0.,0.));
#79791=CARTESIAN_POINT('',(0.,16.2029831402613,-38.1301486668543));
#79792=CARTESIAN_POINT('Ctrl Pts',(1.38777878078145E-16,16.2029831402613,
-38.1301486668543));
#79793=CARTESIAN_POINT('Ctrl Pts',(0.329657621074924,16.3479771490016,-38.4028427364087));
#79794=CARTESIAN_POINT('Ctrl Pts',(0.664285714285715,16.4951409948251,-38.6796176759911));
#79795=CARTESIAN_POINT('Origin',(0.,0.,0.));
#79796=CARTESIAN_POINT('Origin',(0.45,0.,0.));
#79797=CARTESIAN_POINT('',(3.46944695195361E-16,22.5780542486238,-34.7372475355518));
#79798=CARTESIAN_POINT('Ctrl Pts',(4.16333634234434E-16,22.5780542486238,
-34.7372475355518));
#79799=CARTESIAN_POINT('Ctrl Pts',(0.329657618264121,22.7681982991893,-34.9806208219844));
#79800=CARTESIAN_POINT('Ctrl Pts',(0.664285714285709,22.9611878610227,-35.2276361967536));
#79801=CARTESIAN_POINT('Origin',(0.,0.,0.));
#79802=CARTESIAN_POINT('Origin',(0.45,0.,0.));
#79803=CARTESIAN_POINT('',(-4.16333634234434E-16,28.2671026036886,-30.288872715777));
#79804=CARTESIAN_POINT('Ctrl Pts',(-2.77555756156289E-16,28.2671026036886,
-30.288872715777));
#79805=CARTESIAN_POINT('Ctrl Pts',(0.329657616385251,28.4966192652486,-30.4955304460794));
#79806=CARTESIAN_POINT('Ctrl Pts',(0.664285714285712,28.7295706529848,-30.7052808177218));
#79807=CARTESIAN_POINT('Origin',(0.,0.,0.));
#79808=CARTESIAN_POINT('Origin',(0.45,0.,0.));
#79809=CARTESIAN_POINT('',(6.93889390390723E-17,33.0972693499844,-24.9201858254425));
#79810=CARTESIAN_POINT('Ctrl Pts',(0.,33.0972693499844,-24.9201858254425));
#79811=CARTESIAN_POINT('Ctrl Pts',(0.329657624117467,33.3591848821441,-25.0838488142781));
#79812=CARTESIAN_POINT('Ctrl Pts',(0.66428571428571,33.6250199785202,-25.2499610186654));
#79813=CARTESIAN_POINT('Origin',(0.,0.,0.));
#79814=CARTESIAN_POINT('Origin',(0.45,0.,0.));
#79815=CARTESIAN_POINT('',(6.93889390390723E-17,36.9217923151073,-18.7943116990244));
#79816=CARTESIAN_POINT('Ctrl Pts',(1.38777878078145E-16,36.9217923151073,
-18.7943116990244));
#79817=CARTESIAN_POINT('Ctrl Pts',(0.329657623048166,37.2081485406466,-18.9100071240734));
#79818=CARTESIAN_POINT('Ctrl Pts',(0.664285714285706,37.4987900870893,-19.0274339311535));
#79819=CARTESIAN_POINT('Origin',(0.,0.,0.));
#79820=CARTESIAN_POINT('Origin',(0.45,0.,0.));
#79821=CARTESIAN_POINT('',(6.93889390390723E-17,39.6244653040641,-12.097381922012));
#79822=CARTESIAN_POINT('Ctrl Pts',(6.93889390390723E-17,39.6244653040641,
-12.097381922012));
#79823=CARTESIAN_POINT('Ctrl Pts',(0.32965762272503,39.9265614345266,-12.1615944367969));
#79824=CARTESIAN_POINT('Ctrl Pts',(0.664285714285704,40.2331784341656,-12.2267678919898));
#79825=CARTESIAN_POINT('Origin',(0.,0.,0.));
#79826=CARTESIAN_POINT('Origin',(0.45,0.,0.));
#79827=CARTESIAN_POINT('',(6.93889390390723E-17,41.1231689657038,-5.03287931686986));
#79828=CARTESIAN_POINT('Ctrl Pts',(0.,41.1231689657038,-5.03287931686986));
#79829=CARTESIAN_POINT('Ctrl Pts',(0.329657622067524,41.4318259626987,-5.04365785671393));
#79830=CARTESIAN_POINT('Ctrl Pts',(0.664285714285704,41.7451020134904,-5.05459769747091));
#79831=CARTESIAN_POINT('Origin',(0.,0.,0.));
#79832=CARTESIAN_POINT('Origin',(0.,37.1791272503441,-4.89515034526195));
#79833=CARTESIAN_POINT('',(22.,37.1791272503441,-4.89515034526195));
#79834=CARTESIAN_POINT('',(22.,37.1791272503441,-4.89515034526195));
#79835=CARTESIAN_POINT('',(0.,37.1791272503441,-4.89515034526195));
#79836=CARTESIAN_POINT('',(11.,37.4803204240973,-4.90566824265507));
#79837=CARTESIAN_POINT('',(0.,37.1791272503441,-4.89515034526195));
#79838=CARTESIAN_POINT('',(0.,37.1791272503441,-4.89515034526195));
#79839=CARTESIAN_POINT('',(0.,37.1791272503441,-4.89515034526195));
#79840=CARTESIAN_POINT('Origin',(0.,35.764258829506,-11.2768697064435));
#79841=CARTESIAN_POINT('',(22.,35.764258829506,-11.2768697064435));
#79842=CARTESIAN_POINT('',(22.,35.764258829506,-11.2768697064435));
#79843=CARTESIAN_POINT('',(0.,35.764258829506,-11.2768697064435));
#79844=CARTESIAN_POINT('',(11.,36.0590497884572,-11.3395294590896));
#79845=CARTESIAN_POINT('',(0.,35.764258829506,-11.2768697064435));
#79846=CARTESIAN_POINT('',(0.,35.764258829506,-11.2768697064435));
#79847=CARTESIAN_POINT('',(0.,35.764258829506,-11.2768697064435));
#79848=CARTESIAN_POINT('Origin',(0.,33.2627115017215,-17.3159470879662));
#79849=CARTESIAN_POINT('',(22.,33.2627115017215,-17.3159470879662));
#79850=CARTESIAN_POINT('',(22.,33.2627115017215,-17.3159470879662));
#79851=CARTESIAN_POINT('',(0.,33.2627115017215,-17.3159470879662));
#79852=CARTESIAN_POINT('',(11.,33.5421431717545,-17.4288448109885));
#79853=CARTESIAN_POINT('',(0.,33.2627115017215,-17.3159470879662));
#79854=CARTESIAN_POINT('',(0.,33.2627115017215,-17.3159470879662));
#79855=CARTESIAN_POINT('',(0.,33.2627115017215,-17.3159470879662));
#79856=CARTESIAN_POINT('Origin',(0.,29.7504935167013,-22.8288881795131));
#79857=CARTESIAN_POINT('',(22.,29.7504935167013,-22.8288881795131));
#79858=CARTESIAN_POINT('',(22.,29.7504935167013,-22.8288881795131));
#79859=CARTESIAN_POINT('',(0.,29.7504935167013,-22.8288881795131));
#79860=CARTESIAN_POINT('',(11.,30.0060755079215,-22.9885935327265));
#79861=CARTESIAN_POINT('',(0.,29.7504935167013,-22.8288881795131));
#79862=CARTESIAN_POINT('',(0.,29.7504935167013,-22.8288881795131));
#79863=CARTESIAN_POINT('',(0.,29.7504935167013,-22.8288881795131));
#79864=CARTESIAN_POINT('Origin',(0.,25.3343218406523,-27.6481850557002));
#79865=CARTESIAN_POINT('',(22.,25.3343218406523,-27.6481850557002));
#79866=CARTESIAN_POINT('',(22.,25.3343218406523,-27.6481850557002));
#79867=CARTESIAN_POINT('',(0.,25.3343218406523,-27.6481850557002));
#79868=CARTESIAN_POINT('',(11.,25.5582884235871,-27.8498454727622));
#79869=CARTESIAN_POINT('',(0.,25.3343218406523,-27.6481850557002));
#79870=CARTESIAN_POINT('',(0.,25.3343218406523,-27.6481850557002));
#79871=CARTESIAN_POINT('',(0.,25.3343218406523,-27.6481850557002));
#79872=CARTESIAN_POINT('Origin',(0.,20.1483796152605,-31.6274058196267));
#79873=CARTESIAN_POINT('',(22.,20.1483796152605,-31.6274058196267));
#79874=CARTESIAN_POINT('',(22.,20.1483796152605,-31.6274058196267));
#79875=CARTESIAN_POINT('',(0.,20.1483796152605,-31.6274058196267));
#79876=CARTESIAN_POINT('',(11.,20.3339256786199,-31.8648939508099));
#79877=CARTESIAN_POINT('',(0.,20.1483796152605,-31.6274058196267));
#79878=CARTESIAN_POINT('',(0.,20.1483796152605,-31.6274058196267));
#79879=CARTESIAN_POINT('',(0.,20.1483796152605,-31.6274058196267));
#79880=CARTESIAN_POINT('Origin',(0.,14.350239070831,-34.6456438619633));
#79881=CARTESIAN_POINT('',(22.,14.350239070831,-34.6456438619633));
#79882=CARTESIAN_POINT('',(22.,14.350239070831,-34.6456438619633));
#79883=CARTESIAN_POINT('',(0.,14.350239070831,-34.6456438619633));
#79884=CARTESIAN_POINT('',(11.,14.4917268913708,-34.9117437505765));
#79885=CARTESIAN_POINT('',(0.,14.350239070831,-34.6456438619633));
#79886=CARTESIAN_POINT('',(0.,14.350239070831,-34.6456438619633));
#79887=CARTESIAN_POINT('',(0.,14.350239070831,-34.6456438619633));
#79888=CARTESIAN_POINT('Origin',(0.,8.11607377380573,-36.6111915470959));
#79889=CARTESIAN_POINT('',(22.,8.11607377380573,-36.6111915470959));
#79890=CARTESIAN_POINT('',(22.,8.11607377380573,-36.6111915470959));
#79891=CARTESIAN_POINT('',(0.,8.11607377380573,-36.6111915470959));
#79892=CARTESIAN_POINT('',(11.,8.209204315695,-36.8978178826767));
#79893=CARTESIAN_POINT('',(0.,8.11607377380573,-36.6111915470959));
#79894=CARTESIAN_POINT('',(0.,8.11607377380573,-36.6111915470959));
#79895=CARTESIAN_POINT('',(0.,8.11607377380573,-36.6111915470959));
#79896=CARTESIAN_POINT('Origin',(0.,1.63530568209482,-37.4643267032267));
#79897=CARTESIAN_POINT('',(22.,1.63530568209482,-37.4643267032267));
#79898=CARTESIAN_POINT('',(22.,1.63530568209482,-37.4643267032267));
#79899=CARTESIAN_POINT('',(0.,1.63530568209482,-37.4643267032267));
#79900=CARTESIAN_POINT('',(11.,1.67724922094464,-37.7627704896084));
#79901=CARTESIAN_POINT('',(0.,1.63530568209482,-37.4643267032267));
#79902=CARTESIAN_POINT('',(0.,1.63530568209482,-37.4643267032267));
#79903=CARTESIAN_POINT('',(0.,1.63530568209482,-37.4643267032267));
#79904=CARTESIAN_POINT('Origin',(0.,-4.89515034526194,-37.1791272503441));
#79905=CARTESIAN_POINT('',(22.,-4.89515034526194,-37.1791272503441));
#79906=CARTESIAN_POINT('',(22.,-4.89515034526194,-37.1791272503441));
#79907=CARTESIAN_POINT('',(0.,-4.89515034526194,-37.1791272503441));
#79908=CARTESIAN_POINT('',(11.,-4.90566824265507,-37.4803204240973));
#79909=CARTESIAN_POINT('',(0.,-4.89515034526194,-37.1791272503441));
#79910=CARTESIAN_POINT('',(0.,-4.89515034526194,-37.1791272503441));
#79911=CARTESIAN_POINT('',(0.,-4.89515034526194,-37.1791272503441));
#79912=CARTESIAN_POINT('Origin',(0.,-11.2768697064435,-35.764258829506));
#79913=CARTESIAN_POINT('',(22.,-11.2768697064435,-35.764258829506));
#79914=CARTESIAN_POINT('',(22.,-11.2768697064435,-35.764258829506));
#79915=CARTESIAN_POINT('',(0.,-11.2768697064435,-35.764258829506));
#79916=CARTESIAN_POINT('',(0.,-11.2768697064435,-35.764258829506));
#79917=CARTESIAN_POINT('',(0.,-11.2768697064435,-35.764258829506));
#79918=CARTESIAN_POINT('',(0.,-11.2768697064435,-35.764258829506));
#79919=CARTESIAN_POINT('Origin',(0.,-22.8288881795131,-29.7504935167013));
#79920=CARTESIAN_POINT('',(22.,-22.8288881795131,-29.7504935167013));
#79921=CARTESIAN_POINT('',(22.,-22.8288881795131,-29.7504935167013));
#79922=CARTESIAN_POINT('',(0.,-22.8288881795131,-29.7504935167013));
#79923=CARTESIAN_POINT('',(11.,-22.9885935327265,-30.0060755079215));
#79924=CARTESIAN_POINT('',(0.,-22.8288881795131,-29.7504935167013));
#79925=CARTESIAN_POINT('',(0.,-22.8288881795131,-29.7504935167013));
#79926=CARTESIAN_POINT('',(0.,-22.8288881795131,-29.7504935167013));
#79927=CARTESIAN_POINT('Origin',(0.,-27.6481850557002,-25.3343218406523));
#79928=CARTESIAN_POINT('',(22.,-27.6481850557002,-25.3343218406523));
#79929=CARTESIAN_POINT('',(22.,-27.6481850557002,-25.3343218406523));
#79930=CARTESIAN_POINT('',(0.,-27.6481850557002,-25.3343218406523));
#79931=CARTESIAN_POINT('',(11.,-27.8498454727622,-25.5582884235871));
#79932=CARTESIAN_POINT('',(0.,-27.6481850557002,-25.3343218406523));
#79933=CARTESIAN_POINT('',(0.,-27.6481850557002,-25.3343218406523));
#79934=CARTESIAN_POINT('',(0.,-27.6481850557002,-25.3343218406523));
#79935=CARTESIAN_POINT('Origin',(0.,-31.6274058196267,-20.1483796152605));
#79936=CARTESIAN_POINT('',(22.,-31.6274058196267,-20.1483796152605));
#79937=CARTESIAN_POINT('',(22.,-31.6274058196267,-20.1483796152605));
#79938=CARTESIAN_POINT('',(0.,-31.6274058196267,-20.1483796152605));
#79939=CARTESIAN_POINT('',(11.,-31.8648939508099,-20.3339256786199));
#79940=CARTESIAN_POINT('',(0.,-31.6274058196267,-20.1483796152605));
#79941=CARTESIAN_POINT('',(0.,-31.6274058196267,-20.1483796152605));
#79942=CARTESIAN_POINT('',(0.,-31.6274058196267,-20.1483796152605));
#79943=CARTESIAN_POINT('Origin',(0.,-34.6456438619633,-14.3502390708311));
#79944=CARTESIAN_POINT('',(22.,-34.6456438619633,-14.3502390708311));
#79945=CARTESIAN_POINT('',(22.,-34.6456438619633,-14.3502390708311));
#79946=CARTESIAN_POINT('',(0.,-34.6456438619633,-14.3502390708311));
#79947=CARTESIAN_POINT('',(11.,-34.9117437505765,-14.4917268913708));
#79948=CARTESIAN_POINT('',(0.,-34.6456438619633,-14.3502390708311));
#79949=CARTESIAN_POINT('',(0.,-34.6456438619633,-14.3502390708311));
#79950=CARTESIAN_POINT('',(0.,-34.6456438619633,-14.3502390708311));
#79951=CARTESIAN_POINT('Origin',(0.,-36.6111915470959,-8.11607377380573));
#79952=CARTESIAN_POINT('',(22.,-36.6111915470959,-8.11607377380573));
#79953=CARTESIAN_POINT('',(22.,-36.6111915470959,-8.11607377380573));
#79954=CARTESIAN_POINT('',(0.,-36.6111915470959,-8.11607377380573));
#79955=CARTESIAN_POINT('',(11.,-36.8978178826767,-8.209204315695));
#79956=CARTESIAN_POINT('',(0.,-36.6111915470959,-8.11607377380573));
#79957=CARTESIAN_POINT('',(0.,-36.6111915470959,-8.11607377380573));
#79958=CARTESIAN_POINT('',(0.,-36.6111915470959,-8.11607377380573));
#79959=CARTESIAN_POINT('Origin',(0.,-37.4643267032267,-1.63530568209482));
#79960=CARTESIAN_POINT('',(22.,-37.4643267032267,-1.63530568209482));
#79961=CARTESIAN_POINT('',(22.,-37.4643267032267,-1.63530568209482));
#79962=CARTESIAN_POINT('',(0.,-37.4643267032267,-1.63530568209482));
#79963=CARTESIAN_POINT('',(11.,-37.7627704896084,-1.67724922094464));
#79964=CARTESIAN_POINT('',(0.,-37.4643267032267,-1.63530568209482));
#79965=CARTESIAN_POINT('',(0.,-37.4643267032267,-1.63530568209482));
#79966=CARTESIAN_POINT('',(0.,-37.4643267032267,-1.63530568209482));
#79967=CARTESIAN_POINT('Origin',(0.,-37.1791272503441,4.89515034526196));
#79968=CARTESIAN_POINT('',(22.,-37.1791272503441,4.89515034526196));
#79969=CARTESIAN_POINT('',(22.,-37.1791272503441,4.89515034526196));
#79970=CARTESIAN_POINT('',(0.,-37.1791272503441,4.89515034526196));
#79971=CARTESIAN_POINT('',(11.,-37.4803204240973,4.90566824265508));
#79972=CARTESIAN_POINT('',(0.,-37.1791272503441,4.89515034526196));
#79973=CARTESIAN_POINT('',(0.,-37.1791272503441,4.89515034526196));
#79974=CARTESIAN_POINT('',(0.,-37.1791272503441,4.89515034526196));
#79975=CARTESIAN_POINT('Origin',(0.,-35.764258829506,11.2768697064435));
#79976=CARTESIAN_POINT('',(22.,-35.764258829506,11.2768697064435));
#79977=CARTESIAN_POINT('',(22.,-35.764258829506,11.2768697064435));
#79978=CARTESIAN_POINT('',(0.,-35.764258829506,11.2768697064435));
#79979=CARTESIAN_POINT('',(11.,-36.0590497884572,11.3395294590896));
#79980=CARTESIAN_POINT('',(0.,-35.764258829506,11.2768697064435));
#79981=CARTESIAN_POINT('',(0.,-35.764258829506,11.2768697064435));
#79982=CARTESIAN_POINT('',(0.,-35.764258829506,11.2768697064435));
#79983=CARTESIAN_POINT('Origin',(0.,-33.2627115017215,17.3159470879662));
#79984=CARTESIAN_POINT('',(22.,-33.2627115017215,17.3159470879662));
#79985=CARTESIAN_POINT('',(22.,-33.2627115017215,17.3159470879662));
#79986=CARTESIAN_POINT('',(0.,-33.2627115017215,17.3159470879662));
#79987=CARTESIAN_POINT('',(11.,-33.5421431717545,17.4288448109885));
#79988=CARTESIAN_POINT('',(0.,-33.2627115017215,17.3159470879662));
#79989=CARTESIAN_POINT('',(0.,-33.2627115017215,17.3159470879662));
#79990=CARTESIAN_POINT('',(0.,-33.2627115017215,17.3159470879662));
#79991=CARTESIAN_POINT('Origin',(0.,-29.7504935167013,22.8288881795131));
#79992=CARTESIAN_POINT('',(22.,-29.7504935167013,22.8288881795131));
#79993=CARTESIAN_POINT('',(22.,-29.7504935167013,22.8288881795131));
#79994=CARTESIAN_POINT('',(0.,-29.7504935167013,22.8288881795131));
#79995=CARTESIAN_POINT('',(11.,-30.0060755079215,22.9885935327265));
#79996=CARTESIAN_POINT('',(0.,-29.7504935167013,22.8288881795131));
#79997=CARTESIAN_POINT('',(0.,-29.7504935167013,22.8288881795131));
#79998=CARTESIAN_POINT('',(0.,-29.7504935167013,22.8288881795131));
#79999=CARTESIAN_POINT('Origin',(0.,-25.3343218406523,27.6481850557002));
#80000=CARTESIAN_POINT('',(22.,-25.3343218406523,27.6481850557002));
#80001=CARTESIAN_POINT('',(22.,-25.3343218406523,27.6481850557002));
#80002=CARTESIAN_POINT('',(0.,-25.3343218406523,27.6481850557002));
#80003=CARTESIAN_POINT('',(0.,-25.3343218406523,27.6481850557002));
#80004=CARTESIAN_POINT('',(0.,-25.3343218406523,27.6481850557002));
#80005=CARTESIAN_POINT('',(0.,-25.3343218406523,27.6481850557002));
#80006=CARTESIAN_POINT('Origin',(0.,-14.3502390708311,34.6456438619633));
#80007=CARTESIAN_POINT('',(22.,-14.3502390708311,34.6456438619633));
#80008=CARTESIAN_POINT('',(22.,-14.3502390708311,34.6456438619633));
#80009=CARTESIAN_POINT('',(0.,-14.3502390708311,34.6456438619633));
#80010=CARTESIAN_POINT('',(11.,-14.4917268913708,34.9117437505765));
#80011=CARTESIAN_POINT('',(0.,-14.3502390708311,34.6456438619633));
#80012=CARTESIAN_POINT('',(0.,-14.3502390708311,34.6456438619633));
#80013=CARTESIAN_POINT('',(0.,-14.3502390708311,34.6456438619633));
#80014=CARTESIAN_POINT('Origin',(0.,-8.11607377380574,36.6111915470959));
#80015=CARTESIAN_POINT('',(22.,-8.11607377380574,36.6111915470959));
#80016=CARTESIAN_POINT('',(22.,-8.11607377380574,36.6111915470959));
#80017=CARTESIAN_POINT('',(0.,-8.11607377380574,36.6111915470959));
#80018=CARTESIAN_POINT('',(11.,-8.20920431569501,36.8978178826767));
#80019=CARTESIAN_POINT('',(0.,-8.11607377380574,36.6111915470959));
#80020=CARTESIAN_POINT('',(0.,-8.11607377380574,36.6111915470959));
#80021=CARTESIAN_POINT('',(0.,-8.11607377380574,36.6111915470959));
#80022=CARTESIAN_POINT('Origin',(0.,-1.63530568209482,37.4643267032267));
#80023=CARTESIAN_POINT('',(22.,-1.63530568209482,37.4643267032267));
#80024=CARTESIAN_POINT('',(22.,-1.63530568209482,37.4643267032267));
#80025=CARTESIAN_POINT('',(0.,-1.63530568209482,37.4643267032267));
#80026=CARTESIAN_POINT('',(11.,-1.67724922094464,37.7627704896084));
#80027=CARTESIAN_POINT('',(0.,-1.63530568209482,37.4643267032267));
#80028=CARTESIAN_POINT('',(0.,-1.63530568209482,37.4643267032267));
#80029=CARTESIAN_POINT('',(0.,-1.63530568209482,37.4643267032267));
#80030=CARTESIAN_POINT('Origin',(0.,4.89515034526195,37.1791272503441));
#80031=CARTESIAN_POINT('',(22.,4.89515034526195,37.1791272503441));
#80032=CARTESIAN_POINT('',(22.,4.89515034526195,37.1791272503441));
#80033=CARTESIAN_POINT('',(0.,4.89515034526195,37.1791272503441));
#80034=CARTESIAN_POINT('',(11.,4.90566824265507,37.4803204240973));
#80035=CARTESIAN_POINT('',(0.,4.89515034526195,37.1791272503441));
#80036=CARTESIAN_POINT('',(0.,4.89515034526195,37.1791272503441));
#80037=CARTESIAN_POINT('',(0.,4.89515034526195,37.1791272503441));
#80038=CARTESIAN_POINT('Origin',(0.,11.2768697064435,35.764258829506));
#80039=CARTESIAN_POINT('',(22.,11.2768697064435,35.764258829506));
#80040=CARTESIAN_POINT('',(22.,11.2768697064435,35.764258829506));
#80041=CARTESIAN_POINT('',(0.,11.2768697064435,35.764258829506));
#80042=CARTESIAN_POINT('',(11.,11.3395294590896,36.0590497884572));
#80043=CARTESIAN_POINT('',(0.,11.2768697064435,35.764258829506));
#80044=CARTESIAN_POINT('',(0.,11.2768697064435,35.764258829506));
#80045=CARTESIAN_POINT('',(0.,11.2768697064435,35.764258829506));
#80046=CARTESIAN_POINT('Origin',(0.,17.3159470879662,33.2627115017215));
#80047=CARTESIAN_POINT('',(22.,17.3159470879662,33.2627115017215));
#80048=CARTESIAN_POINT('',(22.,17.3159470879662,33.2627115017215));
#80049=CARTESIAN_POINT('',(0.,17.3159470879662,33.2627115017215));
#80050=CARTESIAN_POINT('',(11.,17.4288448109885,33.5421431717545));
#80051=CARTESIAN_POINT('',(0.,17.3159470879662,33.2627115017215));
#80052=CARTESIAN_POINT('',(0.,17.3159470879662,33.2627115017215));
#80053=CARTESIAN_POINT('',(0.,17.3159470879662,33.2627115017215));
#80054=CARTESIAN_POINT('Origin',(0.,22.8288881795131,29.7504935167013));
#80055=CARTESIAN_POINT('',(22.,22.8288881795131,29.7504935167013));
#80056=CARTESIAN_POINT('',(22.,22.8288881795131,29.7504935167013));
#80057=CARTESIAN_POINT('',(0.,22.8288881795131,29.7504935167013));
#80058=CARTESIAN_POINT('',(11.,22.9885935327265,30.0060755079215));
#80059=CARTESIAN_POINT('',(0.,22.8288881795131,29.7504935167013));
#80060=CARTESIAN_POINT('',(0.,22.8288881795131,29.7504935167013));
#80061=CARTESIAN_POINT('',(0.,22.8288881795131,29.7504935167013));
#80062=CARTESIAN_POINT('Origin',(0.,27.6481850557002,25.3343218406523));
#80063=CARTESIAN_POINT('',(22.,27.6481850557002,25.3343218406523));
#80064=CARTESIAN_POINT('',(22.,27.6481850557002,25.3343218406523));
#80065=CARTESIAN_POINT('',(0.,27.6481850557002,25.3343218406523));
#80066=CARTESIAN_POINT('',(11.,27.8498454727622,25.5582884235871));
#80067=CARTESIAN_POINT('',(0.,27.6481850557002,25.3343218406523));
#80068=CARTESIAN_POINT('',(0.,27.6481850557002,25.3343218406523));
#80069=CARTESIAN_POINT('',(0.,27.6481850557002,25.3343218406523));
#80070=CARTESIAN_POINT('Origin',(0.,31.6274058196267,20.1483796152605));
#80071=CARTESIAN_POINT('',(22.,31.6274058196267,20.1483796152605));
#80072=CARTESIAN_POINT('',(22.,31.6274058196267,20.1483796152605));
#80073=CARTESIAN_POINT('',(0.,31.6274058196267,20.1483796152605));
#80074=CARTESIAN_POINT('',(11.,31.8648939508099,20.3339256786199));
#80075=CARTESIAN_POINT('',(0.,31.6274058196267,20.1483796152605));
#80076=CARTESIAN_POINT('',(0.,31.6274058196267,20.1483796152605));
#80077=CARTESIAN_POINT('',(0.,31.6274058196267,20.1483796152605));
#80078=CARTESIAN_POINT('Origin',(0.,34.6456438619633,14.3502390708311));
#80079=CARTESIAN_POINT('',(22.,34.6456438619633,14.3502390708311));
#80080=CARTESIAN_POINT('',(22.,34.6456438619633,14.3502390708311));
#80081=CARTESIAN_POINT('',(0.,34.6456438619633,14.3502390708311));
#80082=CARTESIAN_POINT('',(11.,34.9117437505765,14.4917268913708));
#80083=CARTESIAN_POINT('',(0.,34.6456438619633,14.3502390708311));
#80084=CARTESIAN_POINT('',(0.,34.6456438619633,14.3502390708311));
#80085=CARTESIAN_POINT('',(0.,34.6456438619633,14.3502390708311));
#80086=CARTESIAN_POINT('Origin',(0.,36.6111915470959,8.11607377380574));
#80087=CARTESIAN_POINT('',(22.,36.6111915470959,8.11607377380574));
#80088=CARTESIAN_POINT('',(22.,36.6111915470959,8.11607377380574));
#80089=CARTESIAN_POINT('',(0.,36.6111915470959,8.11607377380574));
#80090=CARTESIAN_POINT('',(0.,36.6111915470959,8.11607377380574));
#80091=CARTESIAN_POINT('',(0.,36.6111915470959,8.11607377380574));
#80092=CARTESIAN_POINT('',(0.,36.6111915470959,8.11607377380574));
#80093=CARTESIAN_POINT('Origin',(0.,37.4643267032267,-1.63530568209483));
#80094=CARTESIAN_POINT('',(0.,37.4643267032267,-1.63530568209483));
#80095=CARTESIAN_POINT('Origin',(0.,37.4643267032267,-1.63530568209483));
#80096=CARTESIAN_POINT('',(22.,37.4643267032267,-1.63530568209483));
#80097=CARTESIAN_POINT('Origin',(22.,39.5633512881141,-3.57953331806381));
#80098=CARTESIAN_POINT('Origin',(0.,39.5633512881141,-3.57953331806381));
#80099=CARTESIAN_POINT('Origin',(11.,0.,0.));
#80100=CARTESIAN_POINT('Origin',(11.,0.,0.));
#80101=CARTESIAN_POINT('Origin',(0.,36.6111915470958,-8.11607377380577));
#80102=CARTESIAN_POINT('',(0.,36.6111915470958,-8.11607377380577));
#80103=CARTESIAN_POINT('Origin',(0.,36.6111915470958,-8.11607377380577));
#80104=CARTESIAN_POINT('',(22.,36.6111915470958,-8.11607377380577));
#80105=CARTESIAN_POINT('Origin',(22.,38.3407156461005,-10.3952560173724));
#80106=CARTESIAN_POINT('Origin',(0.,38.3407156461005,-10.3952560173724));
#80107=CARTESIAN_POINT('Origin',(11.,0.,0.));
#80108=CARTESIAN_POINT('Origin',(0.,34.6456438619633,-14.3502390708311));
#80109=CARTESIAN_POINT('',(0.,34.6456438619633,-14.3502390708311));
#80110=CARTESIAN_POINT('Origin',(0.,34.6456438619633,-14.3502390708311));
#80111=CARTESIAN_POINT('',(22.,34.6456438619633,-14.3502390708311));
#80112=CARTESIAN_POINT('Origin',(22.,35.9531167605183,-16.8951241228465));
#80113=CARTESIAN_POINT('Origin',(0.,35.9531167605183,-16.8951241228465));
#80114=CARTESIAN_POINT('Origin',(11.,0.,0.));
#80115=CARTESIAN_POINT('Origin',(0.,31.6274058196267,-20.1483796152605));
#80116=CARTESIAN_POINT('',(0.,31.6274058196267,-20.1483796152605));
#80117=CARTESIAN_POINT('Origin',(0.,31.6274058196267,-20.1483796152605));
#80118=CARTESIAN_POINT('',(22.,31.6274058196267,-20.1483796152605));
#80119=CARTESIAN_POINT('Origin',(22.,32.4731006153227,-22.8816424311931));
#80120=CARTESIAN_POINT('Origin',(0.,32.4731006153227,-22.8816424311931));
#80121=CARTESIAN_POINT('Origin',(11.,0.,0.));
#80122=CARTESIAN_POINT('Origin',(0.,27.6481850557002,-25.3343218406523));
#80123=CARTESIAN_POINT('',(0.,27.6481850557002,-25.3343218406523));
#80124=CARTESIAN_POINT('Origin',(0.,27.6481850557002,-25.3343218406523));
#80125=CARTESIAN_POINT('',(22.,27.6481850557002,-25.3343218406523));
#80126=CARTESIAN_POINT('Origin',(22.,28.0064057401123,-28.1729136129378));
#80127=CARTESIAN_POINT('Origin',(0.,28.0064057401123,-28.1729136129378));
#80128=CARTESIAN_POINT('Origin',(11.,0.,0.));
#80129=CARTESIAN_POINT('Origin',(0.,22.8288881795131,-29.7504935167013));
#80130=CARTESIAN_POINT('',(0.,22.8288881795131,-29.7504935167013));
#80131=CARTESIAN_POINT('Origin',(0.,22.8288881795131,-29.7504935167013));
#80132=CARTESIAN_POINT('',(22.,22.8288881795131,-29.7504935167013));
#80133=CARTESIAN_POINT('Origin',(22.,22.6887503984137,-32.6081650707355));
#80134=CARTESIAN_POINT('Origin',(0.,22.6887503984137,-32.6081650707355));
#80135=CARTESIAN_POINT('Origin',(11.,0.,0.));
#80136=CARTESIAN_POINT('Origin',(0.,17.3159470879662,-33.2627115017215));
#80137=CARTESIAN_POINT('',(0.,17.3159470879662,-33.2627115017215));
#80138=CARTESIAN_POINT('Origin',(0.,17.3159470879662,-33.2627115017215));
#80139=CARTESIAN_POINT('',(22.,17.3159470879662,-33.2627115017215));
#80140=CARTESIAN_POINT('Origin',(22.,16.681708856921,-36.0526339333865));
#80141=CARTESIAN_POINT('Origin',(0.,16.681708856921,-36.0526339333865));
#80142=CARTESIAN_POINT('Origin',(11.,0.,0.));
#80143=CARTESIAN_POINT('Origin',(0.,11.2768697064435,-35.764258829506));
#80144=CARTESIAN_POINT('',(0.,11.2768697064435,-35.764258829506));
#80145=CARTESIAN_POINT('Origin',(0.,11.2768697064435,-35.764258829506));
#80146=CARTESIAN_POINT('',(22.,11.2768697064435,-35.764258829506));
#80147=CARTESIAN_POINT('Origin',(22.,10.1678020331627,-38.4016617574847));
#80148=CARTESIAN_POINT('Origin',(0.,10.1678020331627,-38.4016617574847));
#80149=CARTESIAN_POINT('Origin',(11.,0.,0.));
#80150=CARTESIAN_POINT('Origin',(0.,4.89515034526193,-37.1791272503441));
#80151=CARTESIAN_POINT('',(0.,4.89515034526193,-37.1791272503441));
#80152=CARTESIAN_POINT('Origin',(0.,4.89515034526193,-37.1791272503441));
#80153=CARTESIAN_POINT('',(22.,4.89515034526193,-37.1791272503441));
#80154=CARTESIAN_POINT('Origin',(22.,3.34495168978286,-39.5838745212602));
#80155=CARTESIAN_POINT('Origin',(0.,3.34495168978286,-39.5838745212602));
#80156=CARTESIAN_POINT('Origin',(11.,0.,0.));
#80157=CARTESIAN_POINT('Origin',(0.,-1.63530568209482,-37.4643267032267));
#80158=CARTESIAN_POINT('',(0.,-1.63530568209482,-37.4643267032267));
#80159=CARTESIAN_POINT('Origin',(0.,-1.63530568209482,-37.4643267032267));
#80160=CARTESIAN_POINT('',(22.,-1.63530568209482,-37.4643267032267));
#80161=CARTESIAN_POINT('Origin',(22.,-3.57953331806381,-39.5633512881141));
#80162=CARTESIAN_POINT('Origin',(0.,-3.57953331806381,-39.5633512881141));
#80163=CARTESIAN_POINT('Origin',(11.,0.,0.));
#80164=CARTESIAN_POINT('Origin',(0.,-8.11607377380577,-36.6111915470959));
#80165=CARTESIAN_POINT('',(0.,-8.11607377380577,-36.6111915470959));
#80166=CARTESIAN_POINT('Origin',(0.,-8.11607377380577,-36.6111915470959));
#80167=CARTESIAN_POINT('',(22.,-8.11607377380577,-36.6111915470959));
#80168=CARTESIAN_POINT('Origin',(22.,-10.3952560173724,-38.3407156461005));
#80169=CARTESIAN_POINT('Origin',(0.,-10.3952560173724,-38.3407156461005));
#80170=CARTESIAN_POINT('Origin',(11.,0.,0.));
#80171=CARTESIAN_POINT('Origin',(0.,-20.1483796152605,-31.6274058196267));
#80172=CARTESIAN_POINT('',(0.,-20.1483796152605,-31.6274058196267));
#80173=CARTESIAN_POINT('Origin',(0.,-20.1483796152605,-31.6274058196267));
#80174=CARTESIAN_POINT('',(22.,-20.1483796152605,-31.6274058196267));
#80175=CARTESIAN_POINT('Origin',(22.,-22.8816424311931,-32.4731006153227));
#80176=CARTESIAN_POINT('Origin',(0.,-22.8816424311931,-32.4731006153227));
#80177=CARTESIAN_POINT('Origin',(11.,0.,0.));
#80178=CARTESIAN_POINT('Origin',(0.,-25.3343218406523,-27.6481850557002));
#80179=CARTESIAN_POINT('',(0.,-25.3343218406523,-27.6481850557002));
#80180=CARTESIAN_POINT('Origin',(0.,-25.3343218406523,-27.6481850557002));
#80181=CARTESIAN_POINT('',(22.,-25.3343218406523,-27.6481850557002));
#80182=CARTESIAN_POINT('Origin',(22.,-28.1729136129378,-28.0064057401123));
#80183=CARTESIAN_POINT('Origin',(0.,-28.1729136129378,-28.0064057401123));
#80184=CARTESIAN_POINT('Origin',(11.,0.,0.));
#80185=CARTESIAN_POINT('Origin',(0.,-29.7504935167013,-22.8288881795131));
#80186=CARTESIAN_POINT('',(0.,-29.7504935167013,-22.8288881795131));
#80187=CARTESIAN_POINT('Origin',(0.,-29.7504935167013,-22.8288881795131));
#80188=CARTESIAN_POINT('',(22.,-29.7504935167013,-22.8288881795131));
#80189=CARTESIAN_POINT('Origin',(22.,-32.6081650707355,-22.6887503984137));
#80190=CARTESIAN_POINT('Origin',(0.,-32.6081650707355,-22.6887503984137));
#80191=CARTESIAN_POINT('Origin',(11.,0.,0.));
#80192=CARTESIAN_POINT('Origin',(0.,-33.2627115017215,-17.3159470879662));
#80193=CARTESIAN_POINT('',(0.,-33.2627115017215,-17.3159470879662));
#80194=CARTESIAN_POINT('Origin',(0.,-33.2627115017215,-17.3159470879662));
#80195=CARTESIAN_POINT('',(22.,-33.2627115017215,-17.3159470879662));
#80196=CARTESIAN_POINT('Origin',(22.,-36.0526339333865,-16.681708856921));
#80197=CARTESIAN_POINT('Origin',(0.,-36.0526339333865,-16.681708856921));
#80198=CARTESIAN_POINT('Origin',(11.,0.,0.));
#80199=CARTESIAN_POINT('Origin',(0.,-35.764258829506,-11.2768697064435));
#80200=CARTESIAN_POINT('',(0.,-35.764258829506,-11.2768697064435));
#80201=CARTESIAN_POINT('Origin',(0.,-35.764258829506,-11.2768697064435));
#80202=CARTESIAN_POINT('',(22.,-35.764258829506,-11.2768697064435));
#80203=CARTESIAN_POINT('Origin',(22.,-38.4016617574847,-10.1678020331627));
#80204=CARTESIAN_POINT('Origin',(0.,-38.4016617574847,-10.1678020331627));
#80205=CARTESIAN_POINT('Origin',(11.,0.,0.));
#80206=CARTESIAN_POINT('Origin',(0.,-37.1791272503441,-4.89515034526194));
#80207=CARTESIAN_POINT('',(0.,-37.1791272503441,-4.89515034526194));
#80208=CARTESIAN_POINT('Origin',(0.,-37.1791272503441,-4.89515034526194));
#80209=CARTESIAN_POINT('',(22.,-37.1791272503441,-4.89515034526194));
#80210=CARTESIAN_POINT('Origin',(22.,-39.5838745212602,-3.34495168978286));
#80211=CARTESIAN_POINT('Origin',(0.,-39.5838745212602,-3.34495168978286));
#80212=CARTESIAN_POINT('Origin',(11.,0.,0.));
#80213=CARTESIAN_POINT('Origin',(0.,-37.4643267032267,1.63530568209484));
#80214=CARTESIAN_POINT('',(0.,-37.4643267032267,1.63530568209484));
#80215=CARTESIAN_POINT('Origin',(0.,-37.4643267032267,1.63530568209484));
#80216=CARTESIAN_POINT('',(22.,-37.4643267032267,1.63530568209484));
#80217=CARTESIAN_POINT('Origin',(22.,-39.5633512881141,3.57953331806382));
#80218=CARTESIAN_POINT('Origin',(0.,-39.5633512881141,3.57953331806382));
#80219=CARTESIAN_POINT('Origin',(11.,0.,0.));
#80220=CARTESIAN_POINT('Origin',(0.,-36.6111915470959,8.11607377380575));
#80221=CARTESIAN_POINT('',(0.,-36.6111915470959,8.11607377380575));
#80222=CARTESIAN_POINT('Origin',(0.,-36.6111915470959,8.11607377380575));
#80223=CARTESIAN_POINT('',(22.,-36.6111915470959,8.11607377380575));
#80224=CARTESIAN_POINT('Origin',(22.,-38.3407156461005,10.3952560173724));
#80225=CARTESIAN_POINT('Origin',(0.,-38.3407156461005,10.3952560173724));
#80226=CARTESIAN_POINT('Origin',(11.,0.,0.));
#80227=CARTESIAN_POINT('Origin',(0.,-34.6456438619633,14.3502390708311));
#80228=CARTESIAN_POINT('',(0.,-34.6456438619633,14.3502390708311));
#80229=CARTESIAN_POINT('Origin',(0.,-34.6456438619633,14.3502390708311));
#80230=CARTESIAN_POINT('',(22.,-34.6456438619633,14.3502390708311));
#80231=CARTESIAN_POINT('Origin',(22.,-35.9531167605183,16.8951241228464));
#80232=CARTESIAN_POINT('Origin',(0.,-35.9531167605183,16.8951241228464));
#80233=CARTESIAN_POINT('Origin',(11.,0.,0.));
#80234=CARTESIAN_POINT('Origin',(0.,-31.6274058196267,20.1483796152605));
#80235=CARTESIAN_POINT('',(0.,-31.6274058196267,20.1483796152605));
#80236=CARTESIAN_POINT('Origin',(0.,-31.6274058196267,20.1483796152605));
#80237=CARTESIAN_POINT('',(22.,-31.6274058196267,20.1483796152605));
#80238=CARTESIAN_POINT('Origin',(22.,-32.4731006153227,22.8816424311931));
#80239=CARTESIAN_POINT('Origin',(0.,-32.4731006153227,22.8816424311931));
#80240=CARTESIAN_POINT('Origin',(11.,0.,0.));
#80241=CARTESIAN_POINT('Origin',(0.,-27.6481850557002,25.3343218406523));
#80242=CARTESIAN_POINT('',(0.,-27.6481850557002,25.3343218406523));
#80243=CARTESIAN_POINT('Origin',(0.,-27.6481850557002,25.3343218406523));
#80244=CARTESIAN_POINT('',(22.,-27.6481850557002,25.3343218406523));
#80245=CARTESIAN_POINT('Origin',(22.,-28.0064057401123,28.1729136129378));
#80246=CARTESIAN_POINT('Origin',(0.,-28.0064057401123,28.1729136129378));
#80247=CARTESIAN_POINT('Origin',(11.,0.,0.));
#80248=CARTESIAN_POINT('Origin',(0.,-17.3159470879662,33.2627115017215));
#80249=CARTESIAN_POINT('',(0.,-17.3159470879662,33.2627115017215));
#80250=CARTESIAN_POINT('Origin',(0.,-17.3159470879662,33.2627115017215));
#80251=CARTESIAN_POINT('',(22.,-17.3159470879662,33.2627115017215));
#80252=CARTESIAN_POINT('Origin',(22.,-16.681708856921,36.0526339333865));
#80253=CARTESIAN_POINT('Origin',(0.,-16.681708856921,36.0526339333865));
#80254=CARTESIAN_POINT('Origin',(11.,0.,0.));
#80255=CARTESIAN_POINT('Origin',(0.,-11.2768697064435,35.764258829506));
#80256=CARTESIAN_POINT('',(0.,-11.2768697064435,35.764258829506));
#80257=CARTESIAN_POINT('Origin',(0.,-11.2768697064435,35.764258829506));
#80258=CARTESIAN_POINT('',(22.,-11.2768697064435,35.764258829506));
#80259=CARTESIAN_POINT('Origin',(22.,-10.1678020331627,38.4016617574847));
#80260=CARTESIAN_POINT('Origin',(0.,-10.1678020331627,38.4016617574847));
#80261=CARTESIAN_POINT('Origin',(11.,0.,0.));
#80262=CARTESIAN_POINT('Origin',(0.,-4.89515034526194,37.1791272503441));
#80263=CARTESIAN_POINT('',(0.,-4.89515034526194,37.1791272503441));
#80264=CARTESIAN_POINT('Origin',(0.,-4.89515034526194,37.1791272503441));
#80265=CARTESIAN_POINT('',(22.,-4.89515034526194,37.1791272503441));
#80266=CARTESIAN_POINT('Origin',(22.,-3.34495168978286,39.5838745212602));
#80267=CARTESIAN_POINT('Origin',(0.,-3.34495168978286,39.5838745212602));
#80268=CARTESIAN_POINT('Origin',(11.,0.,0.));
#80269=CARTESIAN_POINT('Origin',(0.,1.63530568209483,37.4643267032268));
#80270=CARTESIAN_POINT('',(0.,1.63530568209483,37.4643267032268));
#80271=CARTESIAN_POINT('Origin',(0.,1.63530568209483,37.4643267032268));
#80272=CARTESIAN_POINT('',(22.,1.63530568209483,37.4643267032268));
#80273=CARTESIAN_POINT('Origin',(22.,3.57953331806381,39.5633512881141));
#80274=CARTESIAN_POINT('Origin',(0.,3.57953331806381,39.5633512881141));
#80275=CARTESIAN_POINT('Origin',(11.,0.,0.));
#80276=CARTESIAN_POINT('Origin',(0.,8.11607377380574,36.6111915470959));
#80277=CARTESIAN_POINT('',(0.,8.11607377380574,36.6111915470959));
#80278=CARTESIAN_POINT('Origin',(0.,8.11607377380574,36.6111915470959));
#80279=CARTESIAN_POINT('',(22.,8.11607377380574,36.6111915470959));
#80280=CARTESIAN_POINT('Origin',(22.,10.3952560173724,38.3407156461005));
#80281=CARTESIAN_POINT('Origin',(0.,10.3952560173724,38.3407156461005));
#80282=CARTESIAN_POINT('Origin',(11.,0.,0.));
#80283=CARTESIAN_POINT('Origin',(0.,14.3502390708311,34.6456438619633));
#80284=CARTESIAN_POINT('',(0.,14.3502390708311,34.6456438619633));
#80285=CARTESIAN_POINT('Origin',(0.,14.3502390708311,34.6456438619633));
#80286=CARTESIAN_POINT('',(22.,14.3502390708311,34.6456438619633));
#80287=CARTESIAN_POINT('Origin',(22.,16.8951241228464,35.9531167605183));
#80288=CARTESIAN_POINT('Origin',(0.,16.8951241228464,35.9531167605183));
#80289=CARTESIAN_POINT('Origin',(11.,0.,0.));
#80290=CARTESIAN_POINT('Origin',(0.,20.1483796152605,31.6274058196267));
#80291=CARTESIAN_POINT('',(0.,20.1483796152605,31.6274058196267));
#80292=CARTESIAN_POINT('Origin',(0.,20.1483796152605,31.6274058196267));
#80293=CARTESIAN_POINT('',(22.,20.1483796152605,31.6274058196267));
#80294=CARTESIAN_POINT('Origin',(22.,22.8816424311931,32.4731006153227));
#80295=CARTESIAN_POINT('Origin',(0.,22.8816424311931,32.4731006153227));
#80296=CARTESIAN_POINT('Origin',(11.,0.,0.));
#80297=CARTESIAN_POINT('Origin',(0.,25.3343218406523,27.6481850557002));
#80298=CARTESIAN_POINT('',(0.,25.3343218406523,27.6481850557002));
#80299=CARTESIAN_POINT('Origin',(0.,25.3343218406523,27.6481850557002));
#80300=CARTESIAN_POINT('',(22.,25.3343218406523,27.6481850557002));
#80301=CARTESIAN_POINT('Origin',(22.,28.1729136129378,28.0064057401123));
#80302=CARTESIAN_POINT('Origin',(0.,28.1729136129378,28.0064057401123));
#80303=CARTESIAN_POINT('Origin',(11.,0.,0.));
#80304=CARTESIAN_POINT('Origin',(0.,29.7504935167013,22.8288881795131));
#80305=CARTESIAN_POINT('',(0.,29.7504935167013,22.8288881795131));
#80306=CARTESIAN_POINT('Origin',(0.,29.7504935167013,22.8288881795131));
#80307=CARTESIAN_POINT('',(22.,29.7504935167013,22.8288881795131));
#80308=CARTESIAN_POINT('Origin',(22.,32.6081650707355,22.6887503984137));
#80309=CARTESIAN_POINT('Origin',(0.,32.6081650707355,22.6887503984137));
#80310=CARTESIAN_POINT('Origin',(11.,0.,0.));
#80311=CARTESIAN_POINT('Origin',(0.,33.2627115017215,17.3159470879662));
#80312=CARTESIAN_POINT('',(0.,33.2627115017215,17.3159470879662));
#80313=CARTESIAN_POINT('Origin',(0.,33.2627115017215,17.3159470879662));
#80314=CARTESIAN_POINT('',(22.,33.2627115017215,17.3159470879662));
#80315=CARTESIAN_POINT('Origin',(22.,36.0526339333865,16.681708856921));
#80316=CARTESIAN_POINT('Origin',(0.,36.0526339333865,16.681708856921));
#80317=CARTESIAN_POINT('Origin',(11.,0.,0.));
#80318=CARTESIAN_POINT('Origin',(0.,35.764258829506,11.2768697064435));
#80319=CARTESIAN_POINT('',(0.,35.764258829506,11.2768697064435));
#80320=CARTESIAN_POINT('Origin',(0.,35.764258829506,11.2768697064435));
#80321=CARTESIAN_POINT('',(22.,35.764258829506,11.2768697064435));
#80322=CARTESIAN_POINT('Origin',(22.,38.4016617574847,10.1678020331627));
#80323=CARTESIAN_POINT('Origin',(0.,38.4016617574847,10.1678020331627));
#80324=CARTESIAN_POINT('Origin',(19.,0.,0.));
#80325=CARTESIAN_POINT('',(19.,-34.,-4.163799117101E-15));
#80326=CARTESIAN_POINT('',(19.,-4.163799117101E-15,34.));
#80327=CARTESIAN_POINT('Origin',(19.,0.,0.));
#80328=CARTESIAN_POINT('',(18.,-4.04133443718627E-15,33.));
#80329=CARTESIAN_POINT('Origin',(19.,-4.04133443718627E-15,33.));
#80330=CARTESIAN_POINT('Origin',(18.,0.,0.));
#80331=CARTESIAN_POINT('Origin',(19.,0.,0.));
#80332=CARTESIAN_POINT('Origin',(18.,24.,0.));
#80333=CARTESIAN_POINT('',(18.,-3.06161699786838E-15,25.));
#80334=CARTESIAN_POINT('Origin',(18.,0.,0.));
#80335=CARTESIAN_POINT('Origin',(20.,0.,0.));
#80336=CARTESIAN_POINT('',(22.,-34.,-4.163799117101E-15));
#80337=CARTESIAN_POINT('Origin',(22.,0.,0.));
#80338=CARTESIAN_POINT('',(20.,-34.,-4.163799117101E-15));
#80339=CARTESIAN_POINT('Origin',(3.,0.,0.));
#80340=CARTESIAN_POINT('',(4.,-4.04133443718627E-15,33.));
#80341=CARTESIAN_POINT('Origin',(4.,0.,0.));
#80342=CARTESIAN_POINT('',(3.,-4.163799117101E-15,34.));
#80343=CARTESIAN_POINT('Origin',(3.,-4.04133443718627E-15,33.));
#80344=CARTESIAN_POINT('',(3.,-34.,-4.163799117101E-15));
#80345=CARTESIAN_POINT('Origin',(3.,0.,0.));
#80346=CARTESIAN_POINT('Origin',(3.,0.,0.));
#80347=CARTESIAN_POINT('Origin',(4.,34.,0.));
#80348=CARTESIAN_POINT('',(4.,-3.06161699786838E-15,25.));
#80349=CARTESIAN_POINT('Origin',(4.,0.,0.));
#80350=CARTESIAN_POINT('Origin',(2.,0.,0.));
#80351=CARTESIAN_POINT('',(2.,-34.,-4.163799117101E-15));
#80352=CARTESIAN_POINT('Origin',(19.,0.,0.));
#80353=CARTESIAN_POINT('',(19.,-2.93915231795365E-15,24.));
#80354=CARTESIAN_POINT('Origin',(19.,-3.06161699786838E-15,25.));
#80355=CARTESIAN_POINT('',(19.,-24.,-2.93915231795365E-15));
#80356=CARTESIAN_POINT('Origin',(19.,0.,0.));
#80357=CARTESIAN_POINT('Origin',(19.,0.,0.));
#80358=CARTESIAN_POINT('Origin',(20.,0.,0.));
#80359=CARTESIAN_POINT('',(22.,-24.,-2.93915231795365E-15));
#80360=CARTESIAN_POINT('Origin',(22.,0.,0.));
#80361=CARTESIAN_POINT('',(20.,-24.,-2.93915231795365E-15));
#80362=CARTESIAN_POINT('Origin',(3.,0.,0.));
#80363=CARTESIAN_POINT('',(3.,-24.,-2.93915231795365E-15));
#80364=CARTESIAN_POINT('',(3.,-2.93915231795365E-15,24.));
#80365=CARTESIAN_POINT('Origin',(3.,0.,0.));
#80366=CARTESIAN_POINT('Origin',(3.,-3.06161699786838E-15,25.));
#80367=CARTESIAN_POINT('Origin',(3.,0.,0.));
#80368=CARTESIAN_POINT('Origin',(2.,0.,0.));
#80369=CARTESIAN_POINT('',(0.,-24.,-2.93915231795365E-15));
#80370=CARTESIAN_POINT('',(2.,-24.,-2.93915231795365E-15));
#80371=CARTESIAN_POINT('Origin',(0.,0.,0.));
#80372=CARTESIAN_POINT('Origin',(11.,0.,0.));
#80373=CARTESIAN_POINT('',(21.2,-15.01,-1.83819484552018E-15));
#80374=CARTESIAN_POINT('Origin',(21.2,0.,0.));
#80375=CARTESIAN_POINT('',(0.800000000000001,-15.01,-1.83819484552018E-15));
#80376=CARTESIAN_POINT('',(11.,-15.01,-1.83819484552018E-15));
#80377=CARTESIAN_POINT('Origin',(0.800000000000001,0.,0.));
#80378=CARTESIAN_POINT('Origin',(0.4,0.,0.));
#80379=CARTESIAN_POINT('',(-4.85722573273506E-16,-15.81,-1.93616658945197E-15));
#80380=CARTESIAN_POINT('',(0.4,-15.41,-1.88718071748607E-15));
#80381=CARTESIAN_POINT('Origin',(0.,0.,0.));
#80382=CARTESIAN_POINT('Origin',(0.,24.,0.));
#80383=CARTESIAN_POINT('Origin',(22.,34.,0.));
#80384=CARTESIAN_POINT('Origin',(22.,15.81,0.));
#80385=CARTESIAN_POINT('',(22.,-15.81,-1.93616658945197E-15));
#80386=CARTESIAN_POINT('Origin',(22.,0.,0.));
#80387=CARTESIAN_POINT('Origin',(21.6,0.,0.));
#80388=CARTESIAN_POINT('',(21.6,-15.41,-1.88718071748607E-15));
#94272=UNCERTAINTY_MEASURE_WITH_UNIT(LENGTH_MEASURE(0.01),#94302,
'DISTANCE_ACCURACY_VALUE',
'Maximum model space distance between geometric entities at asserted c
onnectivities');
#94285=UNCERTAINTY_MEASURE_WITH_UNIT(LENGTH_MEASURE(0.01),#94302,
'DISTANCE_ACCURACY_VALUE',
'Maximum model space distance between geometric entities at asserted c
onnectivities');
#94288=(
GEOMETRIC_REPRESENTATION_CONTEXT(3)
GLOBAL_UNCERTAINTY_ASSIGNED_CONTEXT((#94272))
GLOBAL_UNIT_ASSIGNED_CONTEXT((#94302,#94304,#94305))
REPRESENTATION_CONTEXT('','3D')
);
#94301=(
GEOMETRIC_REPRESENTATION_CONTEXT(3)
GLOBAL_UNCERTAINTY_ASSIGNED_CONTEXT((#94285))
GLOBAL_UNIT_ASSIGNED_CONTEXT((#94302,#94304,#94305))
REPRESENTATION_CONTEXT('','3D')
);
#94302=(
LENGTH_UNIT()
NAMED_UNIT(*)
SI_UNIT(.MILLI.,.METRE.)
);
#94304=(
NAMED_UNIT(*)
PLANE_ANGLE_UNIT()
SI_UNIT($,.RADIAN.)
);
#94305=(
NAMED_UNIT(*)
SI_UNIT($,.STERADIAN.)
SOLID_ANGLE_UNIT()
);
#94308=SHAPE_DEFINITION_REPRESENTATION(#94323,#94372);
#94323=PRODUCT_DEFINITION_SHAPE('',$,#94388);
#94372=SHAPE_REPRESENTATION('',(#53608),#94288);
#94385=PRODUCT_DEFINITION_CONTEXT('part definition',#94432,'design');
#94388=PRODUCT_DEFINITION('2026-10-11-08-26-33-125',
'02_Splined_Display_Hub_36T',#94403,#94385);
#94403=PRODUCT_DEFINITION_FORMATION('',$,#94436);
#94432=APPLICATION_CONTEXT(
'Core Data for Automotive Mechanical Design Process');
#94433=PRODUCT_CONTEXT('part definition',#94432,'mechanical');
#94436=PRODUCT('2026-10-11-08-26-33-125','02_Splined_Display_Hub_36T',$,
(#94433));
#94589=COLOUR_RGB('Off White',0.89,0.88,0.83);
#94590=FILL_AREA_STYLE_COLOUR('',#94589);
#94591=FILL_AREA_STYLE('',(#94590));
#94592=SURFACE_STYLE_FILL_AREA(#94591);
#94593=SURFACE_SIDE_STYLE('',(#94592));
#94594=SURFACE_STYLE_USAGE(.BOTH.,#94593);
#94595=PRESENTATION_STYLE_ASSIGNMENT((#94594));
ENDSEC;
END-ISO-10303-21;
